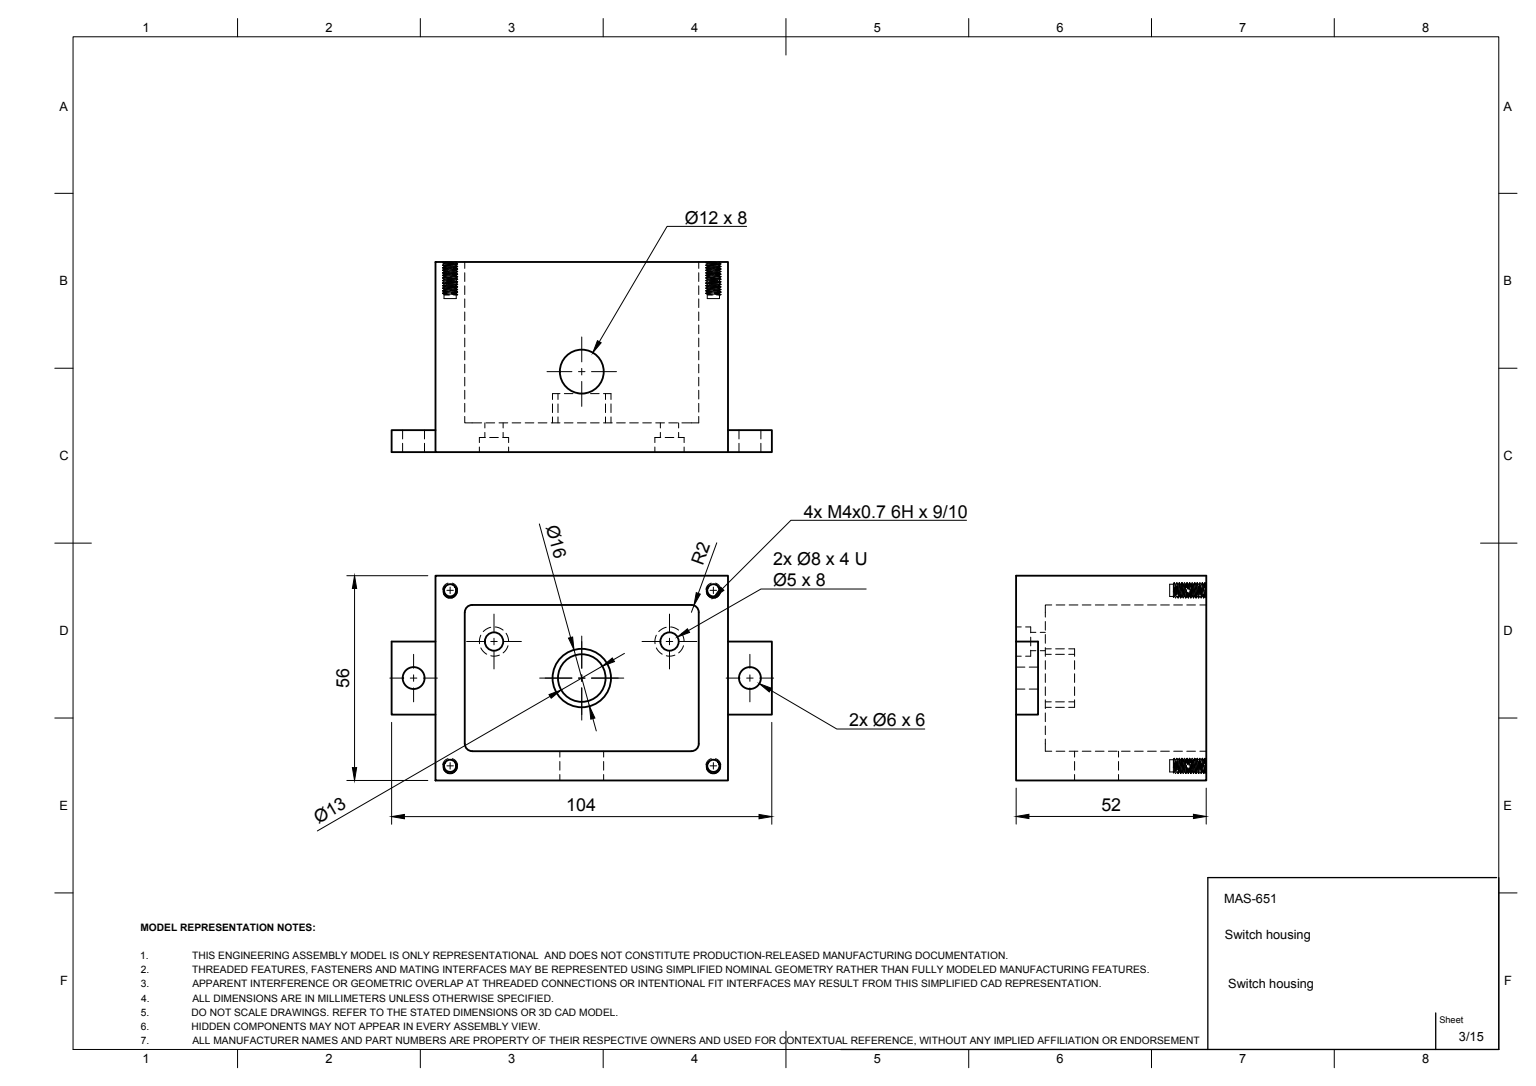
ISO-10303-21;
HEADER;
/* Generated by software containing ST-Developer
 * from STEP Tools, Inc. (www.steptools.com) 
 */

FILE_DESCRIPTION(
/* description */ ('Independent direct-acting normally-closed roller-plunger limit-switch
 CAD. Removable cover, insulated terminal supports, captured bus/conta
ct bridge, native Coil return spring, integral lower travel stop, reus
able instanced hardware and free roller. Manual geometric contact open
ing4mm; no snap-action/contact-force, electrical/current/voltage, envi
ronmental seal, safety-switch, wear, load or life certification. Exter
nal wiring and anchors omitted; fits and application engineering requi
red.'),
/* implementation_level */ '2;1');

FILE_NAME(
/* name */ 'Switch housing.step',
/* time_stamp */ '2026-11-08T07:32:43-08:00',
/* author */ (''),
/* organization */ (''),
/* preprocessor_version */ 'ST-DEVELOPER v20.2',
/* originating_system */ 'Autodesk Translation Framework v15.17.0.0',
/* authorisation */ '');

FILE_SCHEMA (('AUTOMOTIVE_DESIGN { 1 0 10303 214 3 1 1 }'));
ENDSEC;

DATA;
#10=MECHANICAL_DESIGN_GEOMETRIC_PRESENTATION_REPRESENTATION('',(#176),#36482);
#142=SHAPE_REPRESENTATION_RELATIONSHIP('SRR','None',#36555,#159);
#159=ADVANCED_BREP_SHAPE_REPRESENTATION('',(#193),#36465);
#176=STYLED_ITEM('',(#36649),#193);
#193=MANIFOLD_SOLID_BREP('Body1',#9767);
#210=B_SPLINE_SURFACE_WITH_KNOTS('',3,3,((#16536,#16537,#16538,#16539,#16540,
#16541,#16542,#16543,#16544,#16545,#16546,#16547,#16548,#16549,#16550,#16551,
#16552,#16553,#16554,#16555,#16556,#16557,#16558,#16559,#16560,#16561,#16562,
#16563,#16564,#16565,#16566,#16567,#16568,#16569,#16570,#16571,#16572,#16573,
#16574,#16575,#16576,#16577,#16578,#16579,#16580,#16581,#16582,#16583,#16584,
#16585,#16586,#16587,#16588,#16589,#16590,#16591,#16592,#16593,#16594,#16595,
#16596,#16597,#16598,#16599,#16600,#16601,#16602,#16603,#16604,#16605,#16606,
#16607,#16608,#16609,#16610,#16611,#16612,#16613,#16614,#16615,#16616,#16617,
#16618,#16619,#16620,#16621),(#16622,#16623,#16624,#16625,#16626,#16627,
#16628,#16629,#16630,#16631,#16632,#16633,#16634,#16635,#16636,#16637,#16638,
#16639,#16640,#16641,#16642,#16643,#16644,#16645,#16646,#16647,#16648,#16649,
#16650,#16651,#16652,#16653,#16654,#16655,#16656,#16657,#16658,#16659,#16660,
#16661,#16662,#16663,#16664,#16665,#16666,#16667,#16668,#16669,#16670,#16671,
#16672,#16673,#16674,#16675,#16676,#16677,#16678,#16679,#16680,#16681,#16682,
#16683,#16684,#16685,#16686,#16687,#16688,#16689,#16690,#16691,#16692,#16693,
#16694,#16695,#16696,#16697,#16698,#16699,#16700,#16701,#16702,#16703,#16704,
#16705,#16706,#16707),(#16708,#16709,#16710,#16711,#16712,#16713,#16714,
#16715,#16716,#16717,#16718,#16719,#16720,#16721,#16722,#16723,#16724,#16725,
#16726,#16727,#16728,#16729,#16730,#16731,#16732,#16733,#16734,#16735,#16736,
#16737,#16738,#16739,#16740,#16741,#16742,#16743,#16744,#16745,#16746,#16747,
#16748,#16749,#16750,#16751,#16752,#16753,#16754,#16755,#16756,#16757,#16758,
#16759,#16760,#16761,#16762,#16763,#16764,#16765,#16766,#16767,#16768,#16769,
#16770,#16771,#16772,#16773,#16774,#16775,#16776,#16777,#16778,#16779,#16780,
#16781,#16782,#16783,#16784,#16785,#16786,#16787,#16788,#16789,#16790,#16791,
#16792,#16793),(#16794,#16795,#16796,#16797,#16798,#16799,#16800,#16801,
#16802,#16803,#16804,#16805,#16806,#16807,#16808,#16809,#16810,#16811,#16812,
#16813,#16814,#16815,#16816,#16817,#16818,#16819,#16820,#16821,#16822,#16823,
#16824,#16825,#16826,#16827,#16828,#16829,#16830,#16831,#16832,#16833,#16834,
#16835,#16836,#16837,#16838,#16839,#16840,#16841,#16842,#16843,#16844,#16845,
#16846,#16847,#16848,#16849,#16850,#16851,#16852,#16853,#16854,#16855,#16856,
#16857,#16858,#16859,#16860,#16861,#16862,#16863,#16864,#16865,#16866,#16867,
#16868,#16869,#16870,#16871,#16872,#16873,#16874,#16875,#16876,#16877,#16878,
#16879)),.UNSPECIFIED.,.F.,.F.,.F.,(4,4),(4,1,1,1,1,1,1,1,1,1,1,1,1,1,1,
1,1,1,1,1,1,1,1,1,1,1,1,1,1,1,1,1,1,1,1,1,1,1,1,1,1,1,1,1,1,1,1,1,1,1,1,
1,1,1,1,1,1,1,1,1,1,1,1,1,1,1,1,1,1,1,1,1,1,1,1,1,1,1,1,1,1,1,1,4),(0.,
0.0448889834294937),(11.8615800042567,12.8591513772396,13.8567227502226,
14.8542941232055,15.8518654961884,16.8494368691714,17.8470082421543,18.8445796151372,
19.8421509881202,20.8397223611031,21.837293734086,22.834865107069,23.8324364800519,
24.8300078530348,25.8275792260178,26.8251505990007,27.8227219719836,28.8202933449666,
29.8178647179495,30.8154360909324,31.8130074639154,32.8105788368983,33.8081502098812,
34.8057215828642,35.8032929558471,36.80086432883,37.798435701813,38.7960070747959,
39.7935784477789,40.7911498207618,41.7887211937447,42.7862925667277,43.7838639397106,
44.7814353126935,45.7790066856765,46.7765780586594,47.7741494316423,48.7717208046253,
49.7692921776082,50.7668635505911,51.7644349235741,52.762006296557,53.7595776695399,
54.7571490425229,55.7547204155058,56.7522917884887,57.7498631614717,58.7474345344546,
59.7450059074375,60.7425772804205,61.7401486534034,62.7377200263864,63.7352913993693,
64.7328627723522,65.7304341453352,66.7280055183181,67.725576891301,68.723148264284,
69.7207196372669,70.7182910102498,71.7158623832328,72.7134337562157,73.7110051291986,
74.7085765021816,75.7061478751645,76.7037192481474,77.7012906211304,78.6988619941133,
79.6964333670962,80.6940047400792,81.6915761130621,82.689147486045,83.686718859028,
84.6842902320109,85.6818616049939,86.6794329779768,87.6770043509597,88.6745757239427,
89.6721470969256,90.6697184699085,91.6672898428915,92.6648612158744,93.6624325888573,
94.6600039618403),.UNSPECIFIED.);
#211=B_SPLINE_SURFACE_WITH_KNOTS('',3,3,((#16957,#16958,#16959,#16960,#16961,
#16962,#16963,#16964,#16965,#16966,#16967,#16968,#16969,#16970,#16971,#16972,
#16973,#16974,#16975,#16976,#16977,#16978,#16979,#16980,#16981,#16982,#16983,
#16984,#16985,#16986,#16987,#16988,#16989,#16990,#16991,#16992,#16993,#16994,
#16995,#16996,#16997,#16998,#16999,#17000,#17001,#17002,#17003,#17004,#17005,
#17006,#17007,#17008,#17009,#17010,#17011,#17012,#17013,#17014,#17015,#17016,
#17017,#17018,#17019,#17020,#17021,#17022,#17023,#17024,#17025,#17026,#17027,
#17028,#17029,#17030,#17031,#17032,#17033,#17034,#17035,#17036,#17037,#17038,
#17039,#17040,#17041,#17042),(#17043,#17044,#17045,#17046,#17047,#17048,
#17049,#17050,#17051,#17052,#17053,#17054,#17055,#17056,#17057,#17058,#17059,
#17060,#17061,#17062,#17063,#17064,#17065,#17066,#17067,#17068,#17069,#17070,
#17071,#17072,#17073,#17074,#17075,#17076,#17077,#17078,#17079,#17080,#17081,
#17082,#17083,#17084,#17085,#17086,#17087,#17088,#17089,#17090,#17091,#17092,
#17093,#17094,#17095,#17096,#17097,#17098,#17099,#17100,#17101,#17102,#17103,
#17104,#17105,#17106,#17107,#17108,#17109,#17110,#17111,#17112,#17113,#17114,
#17115,#17116,#17117,#17118,#17119,#17120,#17121,#17122,#17123,#17124,#17125,
#17126,#17127,#17128),(#17129,#17130,#17131,#17132,#17133,#17134,#17135,
#17136,#17137,#17138,#17139,#17140,#17141,#17142,#17143,#17144,#17145,#17146,
#17147,#17148,#17149,#17150,#17151,#17152,#17153,#17154,#17155,#17156,#17157,
#17158,#17159,#17160,#17161,#17162,#17163,#17164,#17165,#17166,#17167,#17168,
#17169,#17170,#17171,#17172,#17173,#17174,#17175,#17176,#17177,#17178,#17179,
#17180,#17181,#17182,#17183,#17184,#17185,#17186,#17187,#17188,#17189,#17190,
#17191,#17192,#17193,#17194,#17195,#17196,#17197,#17198,#17199,#17200,#17201,
#17202,#17203,#17204,#17205,#17206,#17207,#17208,#17209,#17210,#17211,#17212,
#17213,#17214),(#17215,#17216,#17217,#17218,#17219,#17220,#17221,#17222,
#17223,#17224,#17225,#17226,#17227,#17228,#17229,#17230,#17231,#17232,#17233,
#17234,#17235,#17236,#17237,#17238,#17239,#17240,#17241,#17242,#17243,#17244,
#17245,#17246,#17247,#17248,#17249,#17250,#17251,#17252,#17253,#17254,#17255,
#17256,#17257,#17258,#17259,#17260,#17261,#17262,#17263,#17264,#17265,#17266,
#17267,#17268,#17269,#17270,#17271,#17272,#17273,#17274,#17275,#17276,#17277,
#17278,#17279,#17280,#17281,#17282,#17283,#17284,#17285,#17286,#17287,#17288,
#17289,#17290,#17291,#17292,#17293,#17294,#17295,#17296,#17297,#17298,#17299,
#17300)),.UNSPECIFIED.,.F.,.F.,.F.,(4,4),(4,1,1,1,1,1,1,1,1,1,1,1,1,1,1,
1,1,1,1,1,1,1,1,1,1,1,1,1,1,1,1,1,1,1,1,1,1,1,1,1,1,1,1,1,1,1,1,1,1,1,1,
1,1,1,1,1,1,1,1,1,1,1,1,1,1,1,1,1,1,1,1,1,1,1,1,1,1,1,1,1,1,1,1,4),(0.,
0.0448889834294937),(14.3981410127769,15.3957123857599,16.3932837587428,
17.3908551317257,18.3884265047087,19.3859978776916,20.3835692506745,21.3811406236575,
22.3787119966404,23.3762833696233,24.3738547426063,25.3714261155892,26.3689974885721,
27.3665688615551,28.364140234538,29.3617116075209,30.3592829805039,31.3568543534868,
32.3544257264697,33.3519970994527,34.3495684724356,35.3471398454185,36.3447112184015,
37.3422825913844,38.3398539643674,39.3374253373503,40.3349967103332,41.3325680833162,
42.3301394562991,43.327710829282,44.325282202265,45.3228535752479,46.3204249482308,
47.3179963212138,48.3155676941967,49.3131390671796,50.3107104401626,51.3082818131455,
52.3058531861284,53.3034245591114,54.3009959320943,55.2985673050772,56.2961386780602,
57.2937100510431,58.291281424026,59.288852797009,60.2864241699919,61.2839955429748,
62.2815669159578,63.2791382889407,64.2767096619236,65.2742810349066,66.2718524078895,
67.2694237808725,68.2669951538554,69.2645665268383,70.2621378998213,71.2597092728042,
72.2572806457871,73.2548520187701,74.252423391753,75.2499947647359,76.2475661377189,
77.2451375107018,78.2427088836847,79.2402802566677,80.2378516296506,81.2354230026336,
82.2329943756165,83.2305657485994,84.2281371215823,85.2257084945653,86.2232798675482,
87.2208512405312,88.2184226135141,89.215993986497,90.21356535948,91.2111367324629,
92.2087081054458,93.2062794784288,94.2038508514117,95.2014222243946,96.1989935973776,
97.1965649703605),.UNSPECIFIED.);
#212=B_SPLINE_SURFACE_WITH_KNOTS('',3,3,((#17509,#17510,#17511,#17512,#17513,
#17514,#17515,#17516,#17517,#17518,#17519,#17520,#17521,#17522,#17523,#17524,
#17525,#17526,#17527,#17528,#17529,#17530,#17531,#17532,#17533,#17534,#17535,
#17536,#17537,#17538,#17539,#17540,#17541,#17542,#17543,#17544,#17545,#17546,
#17547,#17548,#17549,#17550,#17551,#17552,#17553,#17554,#17555,#17556,#17557,
#17558,#17559,#17560,#17561,#17562,#17563,#17564,#17565,#17566,#17567,#17568,
#17569,#17570,#17571,#17572,#17573,#17574,#17575,#17576,#17577,#17578,#17579,
#17580,#17581,#17582,#17583,#17584,#17585,#17586,#17587,#17588,#17589,#17590,
#17591,#17592,#17593,#17594),(#17595,#17596,#17597,#17598,#17599,#17600,
#17601,#17602,#17603,#17604,#17605,#17606,#17607,#17608,#17609,#17610,#17611,
#17612,#17613,#17614,#17615,#17616,#17617,#17618,#17619,#17620,#17621,#17622,
#17623,#17624,#17625,#17626,#17627,#17628,#17629,#17630,#17631,#17632,#17633,
#17634,#17635,#17636,#17637,#17638,#17639,#17640,#17641,#17642,#17643,#17644,
#17645,#17646,#17647,#17648,#17649,#17650,#17651,#17652,#17653,#17654,#17655,
#17656,#17657,#17658,#17659,#17660,#17661,#17662,#17663,#17664,#17665,#17666,
#17667,#17668,#17669,#17670,#17671,#17672,#17673,#17674,#17675,#17676,#17677,
#17678,#17679,#17680),(#17681,#17682,#17683,#17684,#17685,#17686,#17687,
#17688,#17689,#17690,#17691,#17692,#17693,#17694,#17695,#17696,#17697,#17698,
#17699,#17700,#17701,#17702,#17703,#17704,#17705,#17706,#17707,#17708,#17709,
#17710,#17711,#17712,#17713,#17714,#17715,#17716,#17717,#17718,#17719,#17720,
#17721,#17722,#17723,#17724,#17725,#17726,#17727,#17728,#17729,#17730,#17731,
#17732,#17733,#17734,#17735,#17736,#17737,#17738,#17739,#17740,#17741,#17742,
#17743,#17744,#17745,#17746,#17747,#17748,#17749,#17750,#17751,#17752,#17753,
#17754,#17755,#17756,#17757,#17758,#17759,#17760,#17761,#17762,#17763,#17764,
#17765,#17766),(#17767,#17768,#17769,#17770,#17771,#17772,#17773,#17774,
#17775,#17776,#17777,#17778,#17779,#17780,#17781,#17782,#17783,#17784,#17785,
#17786,#17787,#17788,#17789,#17790,#17791,#17792,#17793,#17794,#17795,#17796,
#17797,#17798,#17799,#17800,#17801,#17802,#17803,#17804,#17805,#17806,#17807,
#17808,#17809,#17810,#17811,#17812,#17813,#17814,#17815,#17816,#17817,#17818,
#17819,#17820,#17821,#17822,#17823,#17824,#17825,#17826,#17827,#17828,#17829,
#17830,#17831,#17832,#17833,#17834,#17835,#17836,#17837,#17838,#17839,#17840,
#17841,#17842,#17843,#17844,#17845,#17846,#17847,#17848,#17849,#17850,#17851,
#17852)),.UNSPECIFIED.,.F.,.F.,.F.,(4,4),(4,1,1,1,1,1,1,1,1,1,1,1,1,1,1,
1,1,1,1,1,1,1,1,1,1,1,1,1,1,1,1,1,1,1,1,1,1,1,1,1,1,1,1,1,1,1,1,1,1,1,1,
1,1,1,1,1,1,1,1,1,1,1,1,1,1,1,1,1,1,1,1,1,1,1,1,1,1,1,1,1,1,1,1,4),(0.,
0.0448889834294937),(11.8615800042567,12.8591513772396,13.8567227502226,
14.8542941232055,15.8518654961884,16.8494368691714,17.8470082421543,18.8445796151372,
19.8421509881202,20.8397223611031,21.837293734086,22.834865107069,23.8324364800519,
24.8300078530348,25.8275792260178,26.8251505990007,27.8227219719836,28.8202933449666,
29.8178647179495,30.8154360909324,31.8130074639154,32.8105788368983,33.8081502098812,
34.8057215828642,35.8032929558471,36.80086432883,37.798435701813,38.7960070747959,
39.7935784477789,40.7911498207618,41.7887211937447,42.7862925667277,43.7838639397106,
44.7814353126935,45.7790066856765,46.7765780586594,47.7741494316423,48.7717208046253,
49.7692921776082,50.7668635505911,51.7644349235741,52.762006296557,53.7595776695399,
54.7571490425229,55.7547204155058,56.7522917884887,57.7498631614717,58.7474345344546,
59.7450059074375,60.7425772804205,61.7401486534034,62.7377200263864,63.7352913993693,
64.7328627723522,65.7304341453352,66.7280055183181,67.725576891301,68.723148264284,
69.7207196372669,70.7182910102498,71.7158623832328,72.7134337562157,73.7110051291986,
74.7085765021816,75.7061478751645,76.7037192481474,77.7012906211304,78.6988619941133,
79.6964333670962,80.6940047400792,81.6915761130621,82.689147486045,83.686718859028,
84.6842902320109,85.6818616049939,86.6794329779768,87.6770043509597,88.6745757239427,
89.6721470969256,90.6697184699085,91.6672898428915,92.6648612158744,93.6624325888573,
94.6600039618403),.UNSPECIFIED.);
#213=B_SPLINE_SURFACE_WITH_KNOTS('',3,3,((#17930,#17931,#17932,#17933,#17934,
#17935,#17936,#17937,#17938,#17939,#17940,#17941,#17942,#17943,#17944,#17945,
#17946,#17947,#17948,#17949,#17950,#17951,#17952,#17953,#17954,#17955,#17956,
#17957,#17958,#17959,#17960,#17961,#17962,#17963,#17964,#17965,#17966,#17967,
#17968,#17969,#17970,#17971,#17972,#17973,#17974,#17975,#17976,#17977,#17978,
#17979,#17980,#17981,#17982,#17983,#17984,#17985,#17986,#17987,#17988,#17989,
#17990,#17991,#17992,#17993,#17994,#17995,#17996,#17997,#17998,#17999,#18000,
#18001,#18002,#18003,#18004,#18005,#18006,#18007,#18008,#18009,#18010,#18011,
#18012,#18013,#18014,#18015),(#18016,#18017,#18018,#18019,#18020,#18021,
#18022,#18023,#18024,#18025,#18026,#18027,#18028,#18029,#18030,#18031,#18032,
#18033,#18034,#18035,#18036,#18037,#18038,#18039,#18040,#18041,#18042,#18043,
#18044,#18045,#18046,#18047,#18048,#18049,#18050,#18051,#18052,#18053,#18054,
#18055,#18056,#18057,#18058,#18059,#18060,#18061,#18062,#18063,#18064,#18065,
#18066,#18067,#18068,#18069,#18070,#18071,#18072,#18073,#18074,#18075,#18076,
#18077,#18078,#18079,#18080,#18081,#18082,#18083,#18084,#18085,#18086,#18087,
#18088,#18089,#18090,#18091,#18092,#18093,#18094,#18095,#18096,#18097,#18098,
#18099,#18100,#18101),(#18102,#18103,#18104,#18105,#18106,#18107,#18108,
#18109,#18110,#18111,#18112,#18113,#18114,#18115,#18116,#18117,#18118,#18119,
#18120,#18121,#18122,#18123,#18124,#18125,#18126,#18127,#18128,#18129,#18130,
#18131,#18132,#18133,#18134,#18135,#18136,#18137,#18138,#18139,#18140,#18141,
#18142,#18143,#18144,#18145,#18146,#18147,#18148,#18149,#18150,#18151,#18152,
#18153,#18154,#18155,#18156,#18157,#18158,#18159,#18160,#18161,#18162,#18163,
#18164,#18165,#18166,#18167,#18168,#18169,#18170,#18171,#18172,#18173,#18174,
#18175,#18176,#18177,#18178,#18179,#18180,#18181,#18182,#18183,#18184,#18185,
#18186,#18187),(#18188,#18189,#18190,#18191,#18192,#18193,#18194,#18195,
#18196,#18197,#18198,#18199,#18200,#18201,#18202,#18203,#18204,#18205,#18206,
#18207,#18208,#18209,#18210,#18211,#18212,#18213,#18214,#18215,#18216,#18217,
#18218,#18219,#18220,#18221,#18222,#18223,#18224,#18225,#18226,#18227,#18228,
#18229,#18230,#18231,#18232,#18233,#18234,#18235,#18236,#18237,#18238,#18239,
#18240,#18241,#18242,#18243,#18244,#18245,#18246,#18247,#18248,#18249,#18250,
#18251,#18252,#18253,#18254,#18255,#18256,#18257,#18258,#18259,#18260,#18261,
#18262,#18263,#18264,#18265,#18266,#18267,#18268,#18269,#18270,#18271,#18272,
#18273)),.UNSPECIFIED.,.F.,.F.,.F.,(4,4),(4,1,1,1,1,1,1,1,1,1,1,1,1,1,1,
1,1,1,1,1,1,1,1,1,1,1,1,1,1,1,1,1,1,1,1,1,1,1,1,1,1,1,1,1,1,1,1,1,1,1,1,
1,1,1,1,1,1,1,1,1,1,1,1,1,1,1,1,1,1,1,1,1,1,1,1,1,1,1,1,1,1,1,1,4),(0.,
0.0448889834294937),(14.3981410127769,15.3957123857599,16.3932837587428,
17.3908551317257,18.3884265047087,19.3859978776916,20.3835692506745,21.3811406236575,
22.3787119966404,23.3762833696233,24.3738547426063,25.3714261155892,26.3689974885721,
27.3665688615551,28.364140234538,29.3617116075209,30.3592829805039,31.3568543534868,
32.3544257264697,33.3519970994527,34.3495684724356,35.3471398454185,36.3447112184015,
37.3422825913844,38.3398539643674,39.3374253373503,40.3349967103332,41.3325680833162,
42.3301394562991,43.327710829282,44.325282202265,45.3228535752479,46.3204249482308,
47.3179963212138,48.3155676941967,49.3131390671796,50.3107104401626,51.3082818131455,
52.3058531861284,53.3034245591114,54.3009959320943,55.2985673050772,56.2961386780602,
57.2937100510431,58.291281424026,59.288852797009,60.2864241699919,61.2839955429748,
62.2815669159578,63.2791382889407,64.2767096619237,65.2742810349066,66.2718524078895,
67.2694237808725,68.2669951538554,69.2645665268383,70.2621378998213,71.2597092728042,
72.2572806457871,73.2548520187701,74.252423391753,75.2499947647359,76.2475661377189,
77.2451375107018,78.2427088836847,79.2402802566677,80.2378516296506,81.2354230026336,
82.2329943756165,83.2305657485994,84.2281371215823,85.2257084945653,86.2232798675482,
87.2208512405312,88.2184226135141,89.215993986497,90.21356535948,91.2111367324629,
92.2087081054458,93.2062794784288,94.2038508514117,95.2014222243946,96.1989935973776,
97.1965649703605),.UNSPECIFIED.);
#214=B_SPLINE_SURFACE_WITH_KNOTS('',3,3,((#18482,#18483,#18484,#18485,#18486,
#18487,#18488,#18489,#18490,#18491,#18492,#18493,#18494,#18495,#18496,#18497,
#18498,#18499,#18500,#18501,#18502,#18503,#18504,#18505,#18506,#18507,#18508,
#18509,#18510,#18511,#18512,#18513,#18514,#18515,#18516,#18517,#18518,#18519,
#18520,#18521,#18522,#18523,#18524,#18525,#18526,#18527,#18528,#18529,#18530,
#18531,#18532,#18533,#18534,#18535,#18536,#18537,#18538,#18539,#18540,#18541,
#18542,#18543,#18544,#18545,#18546,#18547,#18548,#18549,#18550,#18551,#18552,
#18553,#18554,#18555,#18556,#18557,#18558,#18559,#18560,#18561,#18562,#18563,
#18564,#18565,#18566,#18567),(#18568,#18569,#18570,#18571,#18572,#18573,
#18574,#18575,#18576,#18577,#18578,#18579,#18580,#18581,#18582,#18583,#18584,
#18585,#18586,#18587,#18588,#18589,#18590,#18591,#18592,#18593,#18594,#18595,
#18596,#18597,#18598,#18599,#18600,#18601,#18602,#18603,#18604,#18605,#18606,
#18607,#18608,#18609,#18610,#18611,#18612,#18613,#18614,#18615,#18616,#18617,
#18618,#18619,#18620,#18621,#18622,#18623,#18624,#18625,#18626,#18627,#18628,
#18629,#18630,#18631,#18632,#18633,#18634,#18635,#18636,#18637,#18638,#18639,
#18640,#18641,#18642,#18643,#18644,#18645,#18646,#18647,#18648,#18649,#18650,
#18651,#18652,#18653),(#18654,#18655,#18656,#18657,#18658,#18659,#18660,
#18661,#18662,#18663,#18664,#18665,#18666,#18667,#18668,#18669,#18670,#18671,
#18672,#18673,#18674,#18675,#18676,#18677,#18678,#18679,#18680,#18681,#18682,
#18683,#18684,#18685,#18686,#18687,#18688,#18689,#18690,#18691,#18692,#18693,
#18694,#18695,#18696,#18697,#18698,#18699,#18700,#18701,#18702,#18703,#18704,
#18705,#18706,#18707,#18708,#18709,#18710,#18711,#18712,#18713,#18714,#18715,
#18716,#18717,#18718,#18719,#18720,#18721,#18722,#18723,#18724,#18725,#18726,
#18727,#18728,#18729,#18730,#18731,#18732,#18733,#18734,#18735,#18736,#18737,
#18738,#18739),(#18740,#18741,#18742,#18743,#18744,#18745,#18746,#18747,
#18748,#18749,#18750,#18751,#18752,#18753,#18754,#18755,#18756,#18757,#18758,
#18759,#18760,#18761,#18762,#18763,#18764,#18765,#18766,#18767,#18768,#18769,
#18770,#18771,#18772,#18773,#18774,#18775,#18776,#18777,#18778,#18779,#18780,
#18781,#18782,#18783,#18784,#18785,#18786,#18787,#18788,#18789,#18790,#18791,
#18792,#18793,#18794,#18795,#18796,#18797,#18798,#18799,#18800,#18801,#18802,
#18803,#18804,#18805,#18806,#18807,#18808,#18809,#18810,#18811,#18812,#18813,
#18814,#18815,#18816,#18817,#18818,#18819,#18820,#18821,#18822,#18823,#18824,
#18825)),.UNSPECIFIED.,.F.,.F.,.F.,(4,4),(4,1,1,1,1,1,1,1,1,1,1,1,1,1,1,
1,1,1,1,1,1,1,1,1,1,1,1,1,1,1,1,1,1,1,1,1,1,1,1,1,1,1,1,1,1,1,1,1,1,1,1,
1,1,1,1,1,1,1,1,1,1,1,1,1,1,1,1,1,1,1,1,1,1,1,1,1,1,1,1,1,1,1,1,4),(0.,
0.0448889834294937),(11.8615800042567,12.8591513772396,13.8567227502225,
14.8542941232055,15.8518654961884,16.8494368691713,17.8470082421543,18.8445796151372,
19.8421509881201,20.8397223611031,21.837293734086,22.8348651070689,23.8324364800519,
24.8300078530348,25.8275792260178,26.8251505990007,27.8227219719836,28.8202933449666,
29.8178647179495,30.8154360909324,31.8130074639154,32.8105788368983,33.8081502098812,
34.8057215828642,35.8032929558471,36.80086432883,37.798435701813,38.7960070747959,
39.7935784477788,40.7911498207618,41.7887211937447,42.7862925667276,43.7838639397106,
44.7814353126935,45.7790066856764,46.7765780586594,47.7741494316423,48.7717208046252,
49.7692921776082,50.7668635505911,51.764434923574,52.762006296557,53.7595776695399,
54.7571490425228,55.7547204155058,56.7522917884887,57.7498631614716,58.7474345344546,
59.7450059074375,60.7425772804204,61.7401486534034,62.7377200263863,63.7352913993692,
64.7328627723522,65.7304341453351,66.728005518318,67.725576891301,68.7231482642839,
69.7207196372668,70.7182910102498,71.7158623832327,72.7134337562156,73.7110051291986,
74.7085765021815,75.7061478751644,76.7037192481474,77.7012906211303,78.6988619941132,
79.6964333670962,80.6940047400791,81.6915761130621,82.689147486045,83.6867188590279,
84.6842902320109,85.6818616049938,86.6794329779767,87.6770043509596,88.6745757239426,
89.6721470969255,90.6697184699085,91.6672898428914,92.6648612158743,93.6624325888573,
94.6600039618402),.UNSPECIFIED.);
#215=B_SPLINE_SURFACE_WITH_KNOTS('',3,3,((#18903,#18904,#18905,#18906,#18907,
#18908,#18909,#18910,#18911,#18912,#18913,#18914,#18915,#18916,#18917,#18918,
#18919,#18920,#18921,#18922,#18923,#18924,#18925,#18926,#18927,#18928,#18929,
#18930,#18931,#18932,#18933,#18934,#18935,#18936,#18937,#18938,#18939,#18940,
#18941,#18942,#18943,#18944,#18945,#18946,#18947,#18948,#18949,#18950,#18951,
#18952,#18953,#18954,#18955,#18956,#18957,#18958,#18959,#18960,#18961,#18962,
#18963,#18964,#18965,#18966,#18967,#18968,#18969,#18970,#18971,#18972,#18973,
#18974,#18975,#18976,#18977,#18978,#18979,#18980,#18981,#18982,#18983,#18984,
#18985,#18986,#18987,#18988),(#18989,#18990,#18991,#18992,#18993,#18994,
#18995,#18996,#18997,#18998,#18999,#19000,#19001,#19002,#19003,#19004,#19005,
#19006,#19007,#19008,#19009,#19010,#19011,#19012,#19013,#19014,#19015,#19016,
#19017,#19018,#19019,#19020,#19021,#19022,#19023,#19024,#19025,#19026,#19027,
#19028,#19029,#19030,#19031,#19032,#19033,#19034,#19035,#19036,#19037,#19038,
#19039,#19040,#19041,#19042,#19043,#19044,#19045,#19046,#19047,#19048,#19049,
#19050,#19051,#19052,#19053,#19054,#19055,#19056,#19057,#19058,#19059,#19060,
#19061,#19062,#19063,#19064,#19065,#19066,#19067,#19068,#19069,#19070,#19071,
#19072,#19073,#19074),(#19075,#19076,#19077,#19078,#19079,#19080,#19081,
#19082,#19083,#19084,#19085,#19086,#19087,#19088,#19089,#19090,#19091,#19092,
#19093,#19094,#19095,#19096,#19097,#19098,#19099,#19100,#19101,#19102,#19103,
#19104,#19105,#19106,#19107,#19108,#19109,#19110,#19111,#19112,#19113,#19114,
#19115,#19116,#19117,#19118,#19119,#19120,#19121,#19122,#19123,#19124,#19125,
#19126,#19127,#19128,#19129,#19130,#19131,#19132,#19133,#19134,#19135,#19136,
#19137,#19138,#19139,#19140,#19141,#19142,#19143,#19144,#19145,#19146,#19147,
#19148,#19149,#19150,#19151,#19152,#19153,#19154,#19155,#19156,#19157,#19158,
#19159,#19160),(#19161,#19162,#19163,#19164,#19165,#19166,#19167,#19168,
#19169,#19170,#19171,#19172,#19173,#19174,#19175,#19176,#19177,#19178,#19179,
#19180,#19181,#19182,#19183,#19184,#19185,#19186,#19187,#19188,#19189,#19190,
#19191,#19192,#19193,#19194,#19195,#19196,#19197,#19198,#19199,#19200,#19201,
#19202,#19203,#19204,#19205,#19206,#19207,#19208,#19209,#19210,#19211,#19212,
#19213,#19214,#19215,#19216,#19217,#19218,#19219,#19220,#19221,#19222,#19223,
#19224,#19225,#19226,#19227,#19228,#19229,#19230,#19231,#19232,#19233,#19234,
#19235,#19236,#19237,#19238,#19239,#19240,#19241,#19242,#19243,#19244,#19245,
#19246)),.UNSPECIFIED.,.F.,.F.,.F.,(4,4),(4,1,1,1,1,1,1,1,1,1,1,1,1,1,1,
1,1,1,1,1,1,1,1,1,1,1,1,1,1,1,1,1,1,1,1,1,1,1,1,1,1,1,1,1,1,1,1,1,1,1,1,
1,1,1,1,1,1,1,1,1,1,1,1,1,1,1,1,1,1,1,1,1,1,1,1,1,1,1,1,1,1,1,1,4),(0.,
0.0448889834294937),(14.3981410127769,15.3957123857599,16.3932837587428,
17.3908551317257,18.3884265047087,19.3859978776916,20.3835692506745,21.3811406236575,
22.3787119966404,23.3762833696233,24.3738547426063,25.3714261155892,26.3689974885721,
27.3665688615551,28.364140234538,29.3617116075209,30.3592829805039,31.3568543534868,
32.3544257264697,33.3519970994527,34.3495684724356,35.3471398454185,36.3447112184015,
37.3422825913844,38.3398539643673,39.3374253373503,40.3349967103332,41.3325680833161,
42.3301394562991,43.327710829282,44.3252822022649,45.3228535752479,46.3204249482308,
47.3179963212137,48.3155676941967,49.3131390671796,50.3107104401625,51.3082818131455,
52.3058531861284,53.3034245591113,54.3009959320943,55.2985673050772,56.2961386780601,
57.2937100510431,58.291281424026,59.2888527970089,60.2864241699919,61.2839955429748,
62.2815669159577,63.2791382889407,64.2767096619236,65.2742810349065,66.2718524078895,
67.2694237808724,68.2669951538553,69.2645665268383,70.2621378998212,71.2597092728041,
72.2572806457871,73.25485201877,74.2524233917529,75.2499947647359,76.2475661377188,
77.2451375107017,78.2427088836847,79.2402802566676,80.2378516296505,81.2354230026335,
82.2329943756164,83.2305657485993,84.2281371215823,85.2257084945652,86.2232798675481,
87.2208512405311,88.218422613514,89.2159939864969,90.2135653594799,91.2111367324628,
92.2087081054457,93.2062794784287,94.2038508514116,95.2014222243945,96.1989935973775,
97.1965649703604),.UNSPECIFIED.);
#216=B_SPLINE_SURFACE_WITH_KNOTS('',3,3,((#19455,#19456,#19457,#19458,#19459,
#19460,#19461,#19462,#19463,#19464,#19465,#19466,#19467,#19468,#19469,#19470,
#19471,#19472,#19473,#19474,#19475,#19476,#19477,#19478,#19479,#19480,#19481,
#19482,#19483,#19484,#19485,#19486,#19487,#19488,#19489,#19490,#19491,#19492,
#19493,#19494,#19495,#19496,#19497,#19498,#19499,#19500,#19501,#19502,#19503,
#19504,#19505,#19506,#19507,#19508,#19509,#19510,#19511,#19512,#19513,#19514,
#19515,#19516,#19517,#19518,#19519,#19520,#19521,#19522,#19523,#19524,#19525,
#19526,#19527,#19528,#19529,#19530,#19531,#19532,#19533,#19534,#19535,#19536,
#19537,#19538,#19539,#19540),(#19541,#19542,#19543,#19544,#19545,#19546,
#19547,#19548,#19549,#19550,#19551,#19552,#19553,#19554,#19555,#19556,#19557,
#19558,#19559,#19560,#19561,#19562,#19563,#19564,#19565,#19566,#19567,#19568,
#19569,#19570,#19571,#19572,#19573,#19574,#19575,#19576,#19577,#19578,#19579,
#19580,#19581,#19582,#19583,#19584,#19585,#19586,#19587,#19588,#19589,#19590,
#19591,#19592,#19593,#19594,#19595,#19596,#19597,#19598,#19599,#19600,#19601,
#19602,#19603,#19604,#19605,#19606,#19607,#19608,#19609,#19610,#19611,#19612,
#19613,#19614,#19615,#19616,#19617,#19618,#19619,#19620,#19621,#19622,#19623,
#19624,#19625,#19626),(#19627,#19628,#19629,#19630,#19631,#19632,#19633,
#19634,#19635,#19636,#19637,#19638,#19639,#19640,#19641,#19642,#19643,#19644,
#19645,#19646,#19647,#19648,#19649,#19650,#19651,#19652,#19653,#19654,#19655,
#19656,#19657,#19658,#19659,#19660,#19661,#19662,#19663,#19664,#19665,#19666,
#19667,#19668,#19669,#19670,#19671,#19672,#19673,#19674,#19675,#19676,#19677,
#19678,#19679,#19680,#19681,#19682,#19683,#19684,#19685,#19686,#19687,#19688,
#19689,#19690,#19691,#19692,#19693,#19694,#19695,#19696,#19697,#19698,#19699,
#19700,#19701,#19702,#19703,#19704,#19705,#19706,#19707,#19708,#19709,#19710,
#19711,#19712),(#19713,#19714,#19715,#19716,#19717,#19718,#19719,#19720,
#19721,#19722,#19723,#19724,#19725,#19726,#19727,#19728,#19729,#19730,#19731,
#19732,#19733,#19734,#19735,#19736,#19737,#19738,#19739,#19740,#19741,#19742,
#19743,#19744,#19745,#19746,#19747,#19748,#19749,#19750,#19751,#19752,#19753,
#19754,#19755,#19756,#19757,#19758,#19759,#19760,#19761,#19762,#19763,#19764,
#19765,#19766,#19767,#19768,#19769,#19770,#19771,#19772,#19773,#19774,#19775,
#19776,#19777,#19778,#19779,#19780,#19781,#19782,#19783,#19784,#19785,#19786,
#19787,#19788,#19789,#19790,#19791,#19792,#19793,#19794,#19795,#19796,#19797,
#19798)),.UNSPECIFIED.,.F.,.F.,.F.,(4,4),(4,1,1,1,1,1,1,1,1,1,1,1,1,1,1,
1,1,1,1,1,1,1,1,1,1,1,1,1,1,1,1,1,1,1,1,1,1,1,1,1,1,1,1,1,1,1,1,1,1,1,1,
1,1,1,1,1,1,1,1,1,1,1,1,1,1,1,1,1,1,1,1,1,1,1,1,1,1,1,1,1,1,1,1,4),(0.,
0.0448889834294937),(11.8615800042567,12.8591513772396,13.8567227502225,
14.8542941232055,15.8518654961884,16.8494368691713,17.8470082421543,18.8445796151372,
19.8421509881202,20.8397223611031,21.837293734086,22.834865107069,23.8324364800519,
24.8300078530348,25.8275792260178,26.8251505990007,27.8227219719836,28.8202933449666,
29.8178647179495,30.8154360909324,31.8130074639154,32.8105788368983,33.8081502098812,
34.8057215828642,35.8032929558471,36.80086432883,37.798435701813,38.7960070747959,
39.7935784477788,40.7911498207618,41.7887211937447,42.7862925667276,43.7838639397106,
44.7814353126935,45.7790066856764,46.7765780586594,47.7741494316423,48.7717208046252,
49.7692921776082,50.7668635505911,51.764434923574,52.762006296557,53.7595776695399,
54.7571490425228,55.7547204155058,56.7522917884887,57.7498631614716,58.7474345344546,
59.7450059074375,60.7425772804204,61.7401486534034,62.7377200263863,63.7352913993692,
64.7328627723522,65.7304341453351,66.728005518318,67.725576891301,68.7231482642839,
69.7207196372669,70.7182910102498,71.7158623832327,72.7134337562156,73.7110051291986,
74.7085765021815,75.7061478751644,76.7037192481474,77.7012906211303,78.6988619941132,
79.6964333670962,80.6940047400791,81.6915761130621,82.689147486045,83.6867188590279,
84.6842902320109,85.6818616049938,86.6794329779767,87.6770043509596,88.6745757239426,
89.6721470969255,90.6697184699085,91.6672898428914,92.6648612158743,93.6624325888573,
94.6600039618402),.UNSPECIFIED.);
#217=B_SPLINE_SURFACE_WITH_KNOTS('',3,3,((#19876,#19877,#19878,#19879,#19880,
#19881,#19882,#19883,#19884,#19885,#19886,#19887,#19888,#19889,#19890,#19891,
#19892,#19893,#19894,#19895,#19896,#19897,#19898,#19899,#19900,#19901,#19902,
#19903,#19904,#19905,#19906,#19907,#19908,#19909,#19910,#19911,#19912,#19913,
#19914,#19915,#19916,#19917,#19918,#19919,#19920,#19921,#19922,#19923,#19924,
#19925,#19926,#19927,#19928,#19929,#19930,#19931,#19932,#19933,#19934,#19935,
#19936,#19937,#19938,#19939,#19940,#19941,#19942,#19943,#19944,#19945,#19946,
#19947,#19948,#19949,#19950,#19951,#19952,#19953,#19954,#19955,#19956,#19957,
#19958,#19959,#19960,#19961),(#19962,#19963,#19964,#19965,#19966,#19967,
#19968,#19969,#19970,#19971,#19972,#19973,#19974,#19975,#19976,#19977,#19978,
#19979,#19980,#19981,#19982,#19983,#19984,#19985,#19986,#19987,#19988,#19989,
#19990,#19991,#19992,#19993,#19994,#19995,#19996,#19997,#19998,#19999,#20000,
#20001,#20002,#20003,#20004,#20005,#20006,#20007,#20008,#20009,#20010,#20011,
#20012,#20013,#20014,#20015,#20016,#20017,#20018,#20019,#20020,#20021,#20022,
#20023,#20024,#20025,#20026,#20027,#20028,#20029,#20030,#20031,#20032,#20033,
#20034,#20035,#20036,#20037,#20038,#20039,#20040,#20041,#20042,#20043,#20044,
#20045,#20046,#20047),(#20048,#20049,#20050,#20051,#20052,#20053,#20054,
#20055,#20056,#20057,#20058,#20059,#20060,#20061,#20062,#20063,#20064,#20065,
#20066,#20067,#20068,#20069,#20070,#20071,#20072,#20073,#20074,#20075,#20076,
#20077,#20078,#20079,#20080,#20081,#20082,#20083,#20084,#20085,#20086,#20087,
#20088,#20089,#20090,#20091,#20092,#20093,#20094,#20095,#20096,#20097,#20098,
#20099,#20100,#20101,#20102,#20103,#20104,#20105,#20106,#20107,#20108,#20109,
#20110,#20111,#20112,#20113,#20114,#20115,#20116,#20117,#20118,#20119,#20120,
#20121,#20122,#20123,#20124,#20125,#20126,#20127,#20128,#20129,#20130,#20131,
#20132,#20133),(#20134,#20135,#20136,#20137,#20138,#20139,#20140,#20141,
#20142,#20143,#20144,#20145,#20146,#20147,#20148,#20149,#20150,#20151,#20152,
#20153,#20154,#20155,#20156,#20157,#20158,#20159,#20160,#20161,#20162,#20163,
#20164,#20165,#20166,#20167,#20168,#20169,#20170,#20171,#20172,#20173,#20174,
#20175,#20176,#20177,#20178,#20179,#20180,#20181,#20182,#20183,#20184,#20185,
#20186,#20187,#20188,#20189,#20190,#20191,#20192,#20193,#20194,#20195,#20196,
#20197,#20198,#20199,#20200,#20201,#20202,#20203,#20204,#20205,#20206,#20207,
#20208,#20209,#20210,#20211,#20212,#20213,#20214,#20215,#20216,#20217,#20218,
#20219)),.UNSPECIFIED.,.F.,.F.,.F.,(4,4),(4,1,1,1,1,1,1,1,1,1,1,1,1,1,1,
1,1,1,1,1,1,1,1,1,1,1,1,1,1,1,1,1,1,1,1,1,1,1,1,1,1,1,1,1,1,1,1,1,1,1,1,
1,1,1,1,1,1,1,1,1,1,1,1,1,1,1,1,1,1,1,1,1,1,1,1,1,1,1,1,1,1,1,1,4),(0.,
0.0448889834294937),(14.3981410127769,15.3957123857599,16.3932837587428,
17.3908551317257,18.3884265047087,19.3859978776916,20.3835692506745,21.3811406236575,
22.3787119966404,23.3762833696233,24.3738547426063,25.3714261155892,26.3689974885721,
27.3665688615551,28.364140234538,29.3617116075209,30.3592829805039,31.3568543534868,
32.3544257264697,33.3519970994527,34.3495684724356,35.3471398454185,36.3447112184015,
37.3422825913844,38.3398539643673,39.3374253373503,40.3349967103332,41.3325680833161,
42.3301394562991,43.327710829282,44.3252822022649,45.3228535752479,46.3204249482308,
47.3179963212137,48.3155676941967,49.3131390671796,50.3107104401625,51.3082818131455,
52.3058531861284,53.3034245591113,54.3009959320943,55.2985673050772,56.2961386780601,
57.2937100510431,58.291281424026,59.2888527970089,60.2864241699919,61.2839955429748,
62.2815669159577,63.2791382889407,64.2767096619236,65.2742810349065,66.2718524078895,
67.2694237808724,68.2669951538553,69.2645665268383,70.2621378998212,71.2597092728041,
72.2572806457871,73.25485201877,74.2524233917529,75.2499947647359,76.2475661377188,
77.2451375107017,78.2427088836847,79.2402802566676,80.2378516296505,81.2354230026335,
82.2329943756164,83.2305657485993,84.2281371215823,85.2257084945652,86.2232798675481,
87.2208512405311,88.218422613514,89.2159939864969,90.2135653594799,91.2111367324628,
92.2087081054457,93.2062794784287,94.2038508514116,95.2014222243945,96.1989935973775,
97.1965649703604),.UNSPECIFIED.);
#235=FACE_BOUND('',#1083,.T.);
#236=FACE_BOUND('',#1084,.T.);
#237=FACE_BOUND('',#1085,.T.);
#238=FACE_BOUND('',#1087,.T.);
#239=FACE_BOUND('',#1091,.T.);
#240=FACE_BOUND('',#1095,.T.);
#241=FACE_BOUND('',#1128,.T.);
#242=FACE_BOUND('',#1133,.T.);
#243=FACE_BOUND('',#1137,.T.);
#244=FACE_BOUND('',#1143,.T.);
#245=FACE_BOUND('',#1146,.T.);
#246=FACE_BOUND('',#1147,.T.);
#247=FACE_BOUND('',#1148,.T.);
#248=FACE_BOUND('',#1149,.T.);
#249=FACE_BOUND('',#1150,.T.);
#250=FACE_BOUND('',#1152,.T.);
#251=FACE_BOUND('',#1153,.T.);
#252=FACE_BOUND('',#1154,.T.);
#253=FACE_BOUND('',#1155,.T.);
#302=PLANE('',#10097);
#303=PLANE('',#10101);
#304=PLANE('',#10105);
#305=PLANE('',#10110);
#306=PLANE('',#10116);
#307=PLANE('',#10122);
#308=PLANE('',#10128);
#309=PLANE('',#10131);
#310=PLANE('',#10134);
#311=PLANE('',#10137);
#312=PLANE('',#10140);
#313=PLANE('',#10141);
#314=PLANE('',#10142);
#315=PLANE('',#10143);
#316=PLANE('',#10150);
#317=PLANE('',#10151);
#318=PLANE('',#10152);
#319=PLANE('',#10153);
#320=PLANE('',#10154);
#321=PLANE('',#10155);
#322=PLANE('',#10156);
#323=PLANE('',#10157);
#324=PLANE('',#10163);
#325=PLANE('',#10164);
#326=PLANE('',#10165);
#327=PLANE('',#10166);
#328=PLANE('',#10167);
#329=PLANE('',#10168);
#330=PLANE('',#10169);
#331=PLANE('',#10170);
#332=PLANE('',#10171);
#439=FACE_OUTER_BOUND('',#977,.T.);
#440=FACE_OUTER_BOUND('',#978,.T.);
#441=FACE_OUTER_BOUND('',#979,.T.);
#442=FACE_OUTER_BOUND('',#980,.T.);
#443=FACE_OUTER_BOUND('',#981,.T.);
#444=FACE_OUTER_BOUND('',#982,.T.);
#445=FACE_OUTER_BOUND('',#983,.T.);
#446=FACE_OUTER_BOUND('',#984,.T.);
#447=FACE_OUTER_BOUND('',#985,.T.);
#448=FACE_OUTER_BOUND('',#986,.T.);
#449=FACE_OUTER_BOUND('',#987,.T.);
#450=FACE_OUTER_BOUND('',#988,.T.);
#451=FACE_OUTER_BOUND('',#989,.T.);
#452=FACE_OUTER_BOUND('',#990,.T.);
#453=FACE_OUTER_BOUND('',#991,.T.);
#454=FACE_OUTER_BOUND('',#992,.T.);
#455=FACE_OUTER_BOUND('',#993,.T.);
#456=FACE_OUTER_BOUND('',#994,.T.);
#457=FACE_OUTER_BOUND('',#995,.T.);
#458=FACE_OUTER_BOUND('',#996,.T.);
#459=FACE_OUTER_BOUND('',#997,.T.);
#460=FACE_OUTER_BOUND('',#998,.T.);
#461=FACE_OUTER_BOUND('',#999,.T.);
#462=FACE_OUTER_BOUND('',#1000,.T.);
#463=FACE_OUTER_BOUND('',#1001,.T.);
#464=FACE_OUTER_BOUND('',#1002,.T.);
#465=FACE_OUTER_BOUND('',#1003,.T.);
#466=FACE_OUTER_BOUND('',#1004,.T.);
#467=FACE_OUTER_BOUND('',#1005,.T.);
#468=FACE_OUTER_BOUND('',#1006,.T.);
#469=FACE_OUTER_BOUND('',#1007,.T.);
#470=FACE_OUTER_BOUND('',#1008,.T.);
#471=FACE_OUTER_BOUND('',#1009,.T.);
#472=FACE_OUTER_BOUND('',#1010,.T.);
#473=FACE_OUTER_BOUND('',#1011,.T.);
#474=FACE_OUTER_BOUND('',#1012,.T.);
#475=FACE_OUTER_BOUND('',#1013,.T.);
#476=FACE_OUTER_BOUND('',#1014,.T.);
#477=FACE_OUTER_BOUND('',#1015,.T.);
#478=FACE_OUTER_BOUND('',#1016,.T.);
#479=FACE_OUTER_BOUND('',#1017,.T.);
#480=FACE_OUTER_BOUND('',#1018,.T.);
#481=FACE_OUTER_BOUND('',#1019,.T.);
#482=FACE_OUTER_BOUND('',#1020,.T.);
#483=FACE_OUTER_BOUND('',#1021,.T.);
#484=FACE_OUTER_BOUND('',#1022,.T.);
#485=FACE_OUTER_BOUND('',#1023,.T.);
#486=FACE_OUTER_BOUND('',#1024,.T.);
#487=FACE_OUTER_BOUND('',#1025,.T.);
#488=FACE_OUTER_BOUND('',#1026,.T.);
#489=FACE_OUTER_BOUND('',#1027,.T.);
#490=FACE_OUTER_BOUND('',#1028,.T.);
#491=FACE_OUTER_BOUND('',#1029,.T.);
#492=FACE_OUTER_BOUND('',#1030,.T.);
#493=FACE_OUTER_BOUND('',#1031,.T.);
#494=FACE_OUTER_BOUND('',#1032,.T.);
#495=FACE_OUTER_BOUND('',#1033,.T.);
#496=FACE_OUTER_BOUND('',#1034,.T.);
#497=FACE_OUTER_BOUND('',#1035,.T.);
#498=FACE_OUTER_BOUND('',#1036,.T.);
#499=FACE_OUTER_BOUND('',#1037,.T.);
#500=FACE_OUTER_BOUND('',#1038,.T.);
#501=FACE_OUTER_BOUND('',#1039,.T.);
#502=FACE_OUTER_BOUND('',#1040,.T.);
#503=FACE_OUTER_BOUND('',#1041,.T.);
#504=FACE_OUTER_BOUND('',#1042,.T.);
#505=FACE_OUTER_BOUND('',#1043,.T.);
#506=FACE_OUTER_BOUND('',#1044,.T.);
#507=FACE_OUTER_BOUND('',#1045,.T.);
#508=FACE_OUTER_BOUND('',#1046,.T.);
#509=FACE_OUTER_BOUND('',#1047,.T.);
#510=FACE_OUTER_BOUND('',#1048,.T.);
#511=FACE_OUTER_BOUND('',#1049,.T.);
#512=FACE_OUTER_BOUND('',#1050,.T.);
#513=FACE_OUTER_BOUND('',#1051,.T.);
#514=FACE_OUTER_BOUND('',#1052,.T.);
#515=FACE_OUTER_BOUND('',#1053,.T.);
#516=FACE_OUTER_BOUND('',#1054,.T.);
#517=FACE_OUTER_BOUND('',#1055,.T.);
#518=FACE_OUTER_BOUND('',#1056,.T.);
#519=FACE_OUTER_BOUND('',#1057,.T.);
#520=FACE_OUTER_BOUND('',#1058,.T.);
#521=FACE_OUTER_BOUND('',#1059,.T.);
#522=FACE_OUTER_BOUND('',#1060,.T.);
#523=FACE_OUTER_BOUND('',#1061,.T.);
#524=FACE_OUTER_BOUND('',#1062,.T.);
#525=FACE_OUTER_BOUND('',#1063,.T.);
#526=FACE_OUTER_BOUND('',#1064,.T.);
#527=FACE_OUTER_BOUND('',#1065,.T.);
#528=FACE_OUTER_BOUND('',#1066,.T.);
#529=FACE_OUTER_BOUND('',#1067,.T.);
#530=FACE_OUTER_BOUND('',#1068,.T.);
#531=FACE_OUTER_BOUND('',#1069,.T.);
#532=FACE_OUTER_BOUND('',#1070,.T.);
#533=FACE_OUTER_BOUND('',#1071,.T.);
#534=FACE_OUTER_BOUND('',#1072,.T.);
#535=FACE_OUTER_BOUND('',#1073,.T.);
#536=FACE_OUTER_BOUND('',#1074,.T.);
#537=FACE_OUTER_BOUND('',#1075,.T.);
#538=FACE_OUTER_BOUND('',#1076,.T.);
#539=FACE_OUTER_BOUND('',#1077,.T.);
#540=FACE_OUTER_BOUND('',#1078,.T.);
#541=FACE_OUTER_BOUND('',#1079,.T.);
#542=FACE_OUTER_BOUND('',#1080,.T.);
#543=FACE_OUTER_BOUND('',#1081,.T.);
#544=FACE_OUTER_BOUND('',#1082,.T.);
#545=FACE_OUTER_BOUND('',#1086,.T.);
#546=FACE_OUTER_BOUND('',#1088,.T.);
#547=FACE_OUTER_BOUND('',#1089,.T.);
#548=FACE_OUTER_BOUND('',#1090,.T.);
#549=FACE_OUTER_BOUND('',#1092,.T.);
#550=FACE_OUTER_BOUND('',#1093,.T.);
#551=FACE_OUTER_BOUND('',#1094,.T.);
#552=FACE_OUTER_BOUND('',#1096,.T.);
#553=FACE_OUTER_BOUND('',#1097,.T.);
#554=FACE_OUTER_BOUND('',#1098,.T.);
#555=FACE_OUTER_BOUND('',#1099,.T.);
#556=FACE_OUTER_BOUND('',#1100,.T.);
#557=FACE_OUTER_BOUND('',#1101,.T.);
#558=FACE_OUTER_BOUND('',#1102,.T.);
#559=FACE_OUTER_BOUND('',#1103,.T.);
#560=FACE_OUTER_BOUND('',#1104,.T.);
#561=FACE_OUTER_BOUND('',#1105,.T.);
#562=FACE_OUTER_BOUND('',#1106,.T.);
#563=FACE_OUTER_BOUND('',#1107,.T.);
#564=FACE_OUTER_BOUND('',#1108,.T.);
#565=FACE_OUTER_BOUND('',#1109,.T.);
#566=FACE_OUTER_BOUND('',#1110,.T.);
#567=FACE_OUTER_BOUND('',#1111,.T.);
#568=FACE_OUTER_BOUND('',#1112,.T.);
#569=FACE_OUTER_BOUND('',#1113,.T.);
#570=FACE_OUTER_BOUND('',#1114,.T.);
#571=FACE_OUTER_BOUND('',#1115,.T.);
#572=FACE_OUTER_BOUND('',#1116,.T.);
#573=FACE_OUTER_BOUND('',#1117,.T.);
#574=FACE_OUTER_BOUND('',#1118,.T.);
#575=FACE_OUTER_BOUND('',#1119,.T.);
#576=FACE_OUTER_BOUND('',#1120,.T.);
#577=FACE_OUTER_BOUND('',#1121,.T.);
#578=FACE_OUTER_BOUND('',#1122,.T.);
#579=FACE_OUTER_BOUND('',#1123,.T.);
#580=FACE_OUTER_BOUND('',#1124,.T.);
#581=FACE_OUTER_BOUND('',#1125,.T.);
#582=FACE_OUTER_BOUND('',#1126,.T.);
#583=FACE_OUTER_BOUND('',#1127,.T.);
#584=FACE_OUTER_BOUND('',#1129,.T.);
#585=FACE_OUTER_BOUND('',#1130,.T.);
#586=FACE_OUTER_BOUND('',#1131,.T.);
#587=FACE_OUTER_BOUND('',#1132,.T.);
#588=FACE_OUTER_BOUND('',#1134,.T.);
#589=FACE_OUTER_BOUND('',#1135,.T.);
#590=FACE_OUTER_BOUND('',#1136,.T.);
#591=FACE_OUTER_BOUND('',#1138,.T.);
#592=FACE_OUTER_BOUND('',#1139,.T.);
#593=FACE_OUTER_BOUND('',#1140,.T.);
#594=FACE_OUTER_BOUND('',#1141,.T.);
#595=FACE_OUTER_BOUND('',#1142,.T.);
#596=FACE_OUTER_BOUND('',#1144,.T.);
#597=FACE_OUTER_BOUND('',#1145,.T.);
#598=FACE_OUTER_BOUND('',#1151,.T.);
#977=EDGE_LOOP('',(#5986,#5987,#5988,#5989,#5990,#5991,#5992,#5993));
#978=EDGE_LOOP('',(#5994,#5995,#5996,#5997));
#979=EDGE_LOOP('',(#5998,#5999,#6000,#6001));
#980=EDGE_LOOP('',(#6002,#6003,#6004,#6005));
#981=EDGE_LOOP('',(#6006,#6007,#6008,#6009));
#982=EDGE_LOOP('',(#6010,#6011,#6012,#6013));
#983=EDGE_LOOP('',(#6014,#6015,#6016,#6017));
#984=EDGE_LOOP('',(#6018,#6019,#6020,#6021));
#985=EDGE_LOOP('',(#6022,#6023,#6024,#6025));
#986=EDGE_LOOP('',(#6026,#6027,#6028,#6029));
#987=EDGE_LOOP('',(#6030,#6031,#6032,#6033));
#988=EDGE_LOOP('',(#6034,#6035,#6036,#6037));
#989=EDGE_LOOP('',(#6038,#6039,#6040,#6041));
#990=EDGE_LOOP('',(#6042,#6043,#6044,#6045));
#991=EDGE_LOOP('',(#6046,#6047,#6048,#6049));
#992=EDGE_LOOP('',(#6050,#6051,#6052,#6053));
#993=EDGE_LOOP('',(#6054,#6055,#6056,#6057));
#994=EDGE_LOOP('',(#6058,#6059,#6060,#6061));
#995=EDGE_LOOP('',(#6062,#6063,#6064,#6065));
#996=EDGE_LOOP('',(#6066,#6067,#6068,#6069));
#997=EDGE_LOOP('',(#6070,#6071,#6072,#6073));
#998=EDGE_LOOP('',(#6074,#6075,#6076,#6077));
#999=EDGE_LOOP('',(#6078,#6079,#6080,#6081));
#1000=EDGE_LOOP('',(#6082,#6083,#6084,#6085));
#1001=EDGE_LOOP('',(#6086,#6087,#6088,#6089));
#1002=EDGE_LOOP('',(#6090,#6091,#6092,#6093,#6094,#6095,#6096,#6097));
#1003=EDGE_LOOP('',(#6098,#6099,#6100,#6101));
#1004=EDGE_LOOP('',(#6102,#6103,#6104,#6105));
#1005=EDGE_LOOP('',(#6106,#6107,#6108,#6109));
#1006=EDGE_LOOP('',(#6110,#6111,#6112,#6113));
#1007=EDGE_LOOP('',(#6114,#6115,#6116,#6117));
#1008=EDGE_LOOP('',(#6118,#6119,#6120,#6121));
#1009=EDGE_LOOP('',(#6122,#6123,#6124,#6125));
#1010=EDGE_LOOP('',(#6126,#6127,#6128,#6129));
#1011=EDGE_LOOP('',(#6130,#6131,#6132,#6133));
#1012=EDGE_LOOP('',(#6134,#6135,#6136,#6137));
#1013=EDGE_LOOP('',(#6138,#6139,#6140,#6141));
#1014=EDGE_LOOP('',(#6142,#6143,#6144,#6145));
#1015=EDGE_LOOP('',(#6146,#6147,#6148,#6149));
#1016=EDGE_LOOP('',(#6150,#6151,#6152,#6153));
#1017=EDGE_LOOP('',(#6154,#6155,#6156,#6157));
#1018=EDGE_LOOP('',(#6158,#6159,#6160,#6161));
#1019=EDGE_LOOP('',(#6162,#6163,#6164,#6165));
#1020=EDGE_LOOP('',(#6166,#6167,#6168,#6169));
#1021=EDGE_LOOP('',(#6170,#6171,#6172,#6173));
#1022=EDGE_LOOP('',(#6174,#6175,#6176,#6177));
#1023=EDGE_LOOP('',(#6178,#6179,#6180,#6181));
#1024=EDGE_LOOP('',(#6182,#6183,#6184,#6185));
#1025=EDGE_LOOP('',(#6186,#6187,#6188,#6189));
#1026=EDGE_LOOP('',(#6190,#6191,#6192,#6193));
#1027=EDGE_LOOP('',(#6194,#6195,#6196,#6197,#6198,#6199,#6200,#6201));
#1028=EDGE_LOOP('',(#6202,#6203,#6204,#6205));
#1029=EDGE_LOOP('',(#6206,#6207,#6208,#6209));
#1030=EDGE_LOOP('',(#6210,#6211,#6212,#6213));
#1031=EDGE_LOOP('',(#6214,#6215,#6216,#6217));
#1032=EDGE_LOOP('',(#6218,#6219,#6220,#6221));
#1033=EDGE_LOOP('',(#6222,#6223,#6224,#6225));
#1034=EDGE_LOOP('',(#6226,#6227,#6228,#6229));
#1035=EDGE_LOOP('',(#6230,#6231,#6232,#6233));
#1036=EDGE_LOOP('',(#6234,#6235,#6236,#6237));
#1037=EDGE_LOOP('',(#6238,#6239,#6240,#6241));
#1038=EDGE_LOOP('',(#6242,#6243,#6244,#6245));
#1039=EDGE_LOOP('',(#6246,#6247,#6248,#6249));
#1040=EDGE_LOOP('',(#6250,#6251,#6252,#6253));
#1041=EDGE_LOOP('',(#6254,#6255,#6256,#6257));
#1042=EDGE_LOOP('',(#6258,#6259,#6260,#6261));
#1043=EDGE_LOOP('',(#6262,#6263,#6264,#6265));
#1044=EDGE_LOOP('',(#6266,#6267,#6268,#6269));
#1045=EDGE_LOOP('',(#6270,#6271,#6272,#6273));
#1046=EDGE_LOOP('',(#6274,#6275,#6276,#6277));
#1047=EDGE_LOOP('',(#6278,#6279,#6280,#6281));
#1048=EDGE_LOOP('',(#6282,#6283,#6284,#6285));
#1049=EDGE_LOOP('',(#6286,#6287,#6288,#6289));
#1050=EDGE_LOOP('',(#6290,#6291,#6292,#6293));
#1051=EDGE_LOOP('',(#6294,#6295,#6296,#6297));
#1052=EDGE_LOOP('',(#6298,#6299,#6300,#6301,#6302,#6303,#6304,#6305));
#1053=EDGE_LOOP('',(#6306,#6307,#6308,#6309));
#1054=EDGE_LOOP('',(#6310,#6311,#6312,#6313));
#1055=EDGE_LOOP('',(#6314,#6315,#6316,#6317));
#1056=EDGE_LOOP('',(#6318,#6319,#6320,#6321));
#1057=EDGE_LOOP('',(#6322,#6323,#6324,#6325));
#1058=EDGE_LOOP('',(#6326,#6327,#6328,#6329));
#1059=EDGE_LOOP('',(#6330,#6331,#6332,#6333));
#1060=EDGE_LOOP('',(#6334,#6335,#6336,#6337));
#1061=EDGE_LOOP('',(#6338,#6339,#6340,#6341));
#1062=EDGE_LOOP('',(#6342,#6343,#6344,#6345));
#1063=EDGE_LOOP('',(#6346,#6347,#6348,#6349));
#1064=EDGE_LOOP('',(#6350,#6351,#6352,#6353));
#1065=EDGE_LOOP('',(#6354,#6355,#6356,#6357));
#1066=EDGE_LOOP('',(#6358,#6359,#6360,#6361));
#1067=EDGE_LOOP('',(#6362,#6363,#6364,#6365));
#1068=EDGE_LOOP('',(#6366,#6367,#6368,#6369));
#1069=EDGE_LOOP('',(#6370,#6371,#6372,#6373));
#1070=EDGE_LOOP('',(#6374,#6375,#6376,#6377));
#1071=EDGE_LOOP('',(#6378,#6379,#6380,#6381));
#1072=EDGE_LOOP('',(#6382,#6383,#6384,#6385));
#1073=EDGE_LOOP('',(#6386,#6387,#6388,#6389));
#1074=EDGE_LOOP('',(#6390,#6391,#6392,#6393));
#1075=EDGE_LOOP('',(#6394,#6395,#6396,#6397));
#1076=EDGE_LOOP('',(#6398,#6399,#6400,#6401));
#1077=EDGE_LOOP('',(#6402,#6403,#6404,#6405));
#1078=EDGE_LOOP('',(#6406,#6407,#6408,#6409));
#1079=EDGE_LOOP('',(#6410,#6411,#6412,#6413));
#1080=EDGE_LOOP('',(#6414,#6415,#6416,#6417));
#1081=EDGE_LOOP('',(#6418,#6419,#6420,#6421));
#1082=EDGE_LOOP('',(#6422,#6423,#6424,#6425,#6426,#6427,#6428,#6429));
#1083=EDGE_LOOP('',(#6430));
#1084=EDGE_LOOP('',(#6431));
#1085=EDGE_LOOP('',(#6432));
#1086=EDGE_LOOP('',(#6433,#6434,#6435,#6436));
#1087=EDGE_LOOP('',(#6437));
#1088=EDGE_LOOP('',(#6438,#6439,#6440,#6441));
#1089=EDGE_LOOP('',(#6442,#6443,#6444,#6445));
#1090=EDGE_LOOP('',(#6446));
#1091=EDGE_LOOP('',(#6447));
#1092=EDGE_LOOP('',(#6448,#6449,#6450,#6451));
#1093=EDGE_LOOP('',(#6452,#6453,#6454,#6455));
#1094=EDGE_LOOP('',(#6456));
#1095=EDGE_LOOP('',(#6457));
#1096=EDGE_LOOP('',(#6458,#6459,#6460,#6461));
#1097=EDGE_LOOP('',(#6462,#6463,#6464,#6465));
#1098=EDGE_LOOP('',(#6466,#6467,#6468,#6469));
#1099=EDGE_LOOP('',(#6470,#6471,#6472,#6473));
#1100=EDGE_LOOP('',(#6474,#6475,#6476,#6477,#6478,#6479,#6480,#6481,#6482,
#6483,#6484,#6485,#6486,#6487,#6488,#6489,#6490,#6491,#6492,#6493,#6494,
#6495,#6496,#6497,#6498,#6499,#6500,#6501,#6502,#6503));
#1101=EDGE_LOOP('',(#6504,#6505,#6506,#6507,#6508,#6509,#6510,#6511,#6512,
#6513,#6514,#6515,#6516,#6517,#6518,#6519,#6520,#6521,#6522,#6523,#6524,
#6525,#6526,#6527,#6528,#6529,#6530,#6531,#6532));
#1102=EDGE_LOOP('',(#6533,#6534,#6535,#6536));
#1103=EDGE_LOOP('',(#6537,#6538,#6539,#6540));
#1104=EDGE_LOOP('',(#6541,#6542,#6543,#6544));
#1105=EDGE_LOOP('',(#6545,#6546,#6547,#6548,#6549,#6550,#6551,#6552,#6553,
#6554,#6555,#6556,#6557,#6558,#6559,#6560,#6561,#6562,#6563,#6564,#6565,
#6566,#6567,#6568,#6569,#6570,#6571,#6572,#6573,#6574));
#1106=EDGE_LOOP('',(#6575,#6576,#6577,#6578,#6579,#6580,#6581,#6582,#6583,
#6584,#6585,#6586,#6587,#6588,#6589,#6590,#6591,#6592,#6593,#6594,#6595,
#6596,#6597,#6598,#6599,#6600,#6601,#6602,#6603));
#1107=EDGE_LOOP('',(#6604,#6605,#6606,#6607));
#1108=EDGE_LOOP('',(#6608,#6609,#6610,#6611));
#1109=EDGE_LOOP('',(#6612,#6613,#6614,#6615));
#1110=EDGE_LOOP('',(#6616,#6617,#6618,#6619,#6620,#6621,#6622,#6623,#6624,
#6625,#6626,#6627,#6628,#6629,#6630,#6631,#6632,#6633,#6634,#6635,#6636,
#6637,#6638,#6639,#6640,#6641,#6642,#6643,#6644,#6645));
#1111=EDGE_LOOP('',(#6646,#6647,#6648,#6649,#6650,#6651,#6652,#6653,#6654,
#6655,#6656,#6657,#6658,#6659,#6660,#6661,#6662,#6663,#6664,#6665,#6666,
#6667,#6668,#6669,#6670,#6671,#6672,#6673,#6674));
#1112=EDGE_LOOP('',(#6675,#6676,#6677,#6678));
#1113=EDGE_LOOP('',(#6679,#6680,#6681,#6682));
#1114=EDGE_LOOP('',(#6683,#6684,#6685,#6686));
#1115=EDGE_LOOP('',(#6687,#6688,#6689,#6690,#6691,#6692,#6693,#6694,#6695,
#6696,#6697,#6698,#6699,#6700,#6701,#6702,#6703,#6704,#6705,#6706,#6707,
#6708,#6709,#6710,#6711,#6712,#6713,#6714,#6715,#6716));
#1116=EDGE_LOOP('',(#6717,#6718,#6719,#6720,#6721,#6722,#6723,#6724,#6725,
#6726,#6727,#6728,#6729,#6730,#6731,#6732,#6733,#6734,#6735,#6736,#6737,
#6738,#6739,#6740,#6741,#6742,#6743,#6744,#6745));
#1117=EDGE_LOOP('',(#6746,#6747,#6748,#6749));
#1118=EDGE_LOOP('',(#6750));
#1119=EDGE_LOOP('',(#6751));
#1120=EDGE_LOOP('',(#6752));
#1121=EDGE_LOOP('',(#6753));
#1122=EDGE_LOOP('',(#6754,#6755,#6756,#6757));
#1123=EDGE_LOOP('',(#6758,#6759,#6760,#6761));
#1124=EDGE_LOOP('',(#6762,#6763,#6764,#6765));
#1125=EDGE_LOOP('',(#6766,#6767,#6768,#6769));
#1126=EDGE_LOOP('',(#6770,#6771,#6772,#6773));
#1127=EDGE_LOOP('',(#6774,#6775,#6776,#6777));
#1128=EDGE_LOOP('',(#6778));
#1129=EDGE_LOOP('',(#6779,#6780,#6781,#6782));
#1130=EDGE_LOOP('',(#6783,#6784,#6785,#6786));
#1131=EDGE_LOOP('',(#6787,#6788,#6789,#6790));
#1132=EDGE_LOOP('',(#6791,#6792,#6793,#6794));
#1133=EDGE_LOOP('',(#6795));
#1134=EDGE_LOOP('',(#6796,#6797,#6798,#6799));
#1135=EDGE_LOOP('',(#6800,#6801,#6802,#6803));
#1136=EDGE_LOOP('',(#6804));
#1137=EDGE_LOOP('',(#6805));
#1138=EDGE_LOOP('',(#6806,#6807,#6808,#6809));
#1139=EDGE_LOOP('',(#6810));
#1140=EDGE_LOOP('',(#6811,#6812,#6813,#6814));
#1141=EDGE_LOOP('',(#6815,#6816,#6817,#6818,#6819,#6820,#6821,#6822));
#1142=EDGE_LOOP('',(#6823,#6824,#6825,#6826));
#1143=EDGE_LOOP('',(#6827));
#1144=EDGE_LOOP('',(#6828,#6829,#6830,#6831,#6832,#6833,#6834,#6835));
#1145=EDGE_LOOP('',(#6836,#6837,#6838,#6839));
#1146=EDGE_LOOP('',(#6840,#6841,#6842,#6843));
#1147=EDGE_LOOP('',(#6844,#6845,#6846,#6847));
#1148=EDGE_LOOP('',(#6848,#6849,#6850,#6851));
#1149=EDGE_LOOP('',(#6852,#6853,#6854,#6855));
#1150=EDGE_LOOP('',(#6856,#6857,#6858,#6859,#6860,#6861,#6862,#6863));
#1151=EDGE_LOOP('',(#6864,#6865,#6866,#6867,#6868,#6869,#6870,#6871,#6872,
#6873,#6874,#6875));
#1152=EDGE_LOOP('',(#6876));
#1153=EDGE_LOOP('',(#6877));
#1154=EDGE_LOOP('',(#6878));
#1155=EDGE_LOOP('',(#6879));
#1582=CIRCLE('',#9975,0.1666);
#1583=CIRCLE('',#9976,0.1666);
#1584=CIRCLE('',#9988,0.1666);
#1585=CIRCLE('',#9990,0.205475);
#1586=CIRCLE('',#10003,0.205475);
#1587=CIRCLE('',#10005,0.1666);
#1588=CIRCLE('',#10006,0.1666);
#1589=CIRCLE('',#10018,0.1666);
#1590=CIRCLE('',#10020,0.205475000000001);
#1591=CIRCLE('',#10033,0.205475000000001);
#1592=CIRCLE('',#10035,0.1666);
#1593=CIRCLE('',#10036,0.1666);
#1594=CIRCLE('',#10048,0.1666);
#1595=CIRCLE('',#10050,0.205475000000001);
#1596=CIRCLE('',#10063,0.205475000000001);
#1597=CIRCLE('',#10065,0.1666);
#1598=CIRCLE('',#10066,0.1666);
#1599=CIRCLE('',#10078,0.1666);
#1600=CIRCLE('',#10080,0.205475);
#1601=CIRCLE('',#10093,0.205475);
#1602=CIRCLE('',#10095,0.2);
#1603=CIRCLE('',#10096,0.2);
#1604=CIRCLE('',#10099,0.2);
#1605=CIRCLE('',#10100,0.2);
#1606=CIRCLE('',#10103,0.2);
#1607=CIRCLE('',#10104,0.2);
#1608=CIRCLE('',#10106,0.2);
#1609=CIRCLE('',#10107,0.8);
#1610=CIRCLE('',#10108,0.25);
#1611=CIRCLE('',#10109,0.25);
#1612=CIRCLE('',#10111,0.6);
#1613=CIRCLE('',#10113,0.2);
#1614=CIRCLE('',#10115,0.6);
#1615=CIRCLE('',#10117,0.4);
#1616=CIRCLE('',#10118,0.25);
#1617=CIRCLE('',#10120,0.4);
#1618=CIRCLE('',#10123,0.4);
#1619=CIRCLE('',#10124,0.25);
#1620=CIRCLE('',#10126,0.4);
#1621=CIRCLE('',#10145,0.3);
#1622=CIRCLE('',#10146,0.3);
#1623=CIRCLE('',#10148,0.3);
#1624=CIRCLE('',#10149,0.3);
#1625=CIRCLE('',#10159,0.65);
#1626=CIRCLE('',#10160,0.65);
#1627=CIRCLE('',#10162,0.8);
#1738=B_SPLINE_CURVE_WITH_KNOTS('',3,(#12707,#12708,#12709,#12710,#12711,
#12712,#12713,#12714,#12715,#12716,#12717,#12718,#12719,#12720,#12721,#12722,
#12723,#12724,#12725,#12726,#12727,#12728),.UNSPECIFIED.,.F.,.F.,(4,3,3,
3,3,3,3,4),(76.708045941327,76.8129957196859,77.8105670926688,78.8081384656518,
79.8057098386347,80.8032812116176,81.8008525846006,82.7984239575835),
 .UNSPECIFIED.);
#1739=B_SPLINE_CURVE_WITH_KNOTS('',3,(#12732,#12733,#12734,#12735,#12736,
#12737,#12738),.UNSPECIFIED.,.F.,.F.,(4,3,4),(-80.783811092309,-79.8057098386347,
-79.2446069498473),.UNSPECIFIED.);
#1740=B_SPLINE_CURVE_WITH_KNOTS('',3,(#12742,#12743,#12744,#12745,#12746,
#12747,#12748,#12749,#12750,#12751,#12752,#12753,#12754,#12755,#12756,#12757,
#12758,#12759,#12760,#12761,#12762,#12763),.UNSPECIFIED.,.F.,.F.,(4,3,3,
3,3,3,3,4),(-79.2446069498473,-78.8081384656518,-77.8105670926688,-76.8129957196859,
-75.815424346703,-74.81785297372,-73.8202816007371,-72.9614216426678),
 .UNSPECIFIED.);
#1741=B_SPLINE_CURVE_WITH_KNOTS('',3,(#12768,#12769,#12770,#12771,#12772,
#12773,#12774,#12775,#12776,#12777,#12778,#12779,#12780,#12781,#12782,#12783,
#12784,#12785,#12786,#12787,#12788,#12789),.UNSPECIFIED.,.F.,.F.,(4,3,3,
3,3,3,3,4),(70.4248606341475,70.8275674817883,71.8251388547712,72.8227102277542,
73.8202816007371,74.81785297372,75.815424346703,76.708045941327),
 .UNSPECIFIED.);
#1742=B_SPLINE_CURVE_WITH_KNOTS('',3,(#12790,#12791,#12792,#12793,#12794,
#12795,#12796,#12797,#12798,#12799,#12800,#12801,#12802,#12803,#12804,#12805,
#12806,#12807,#12808,#12809,#12810,#12811,#12812,#12813,#12814),
 .UNSPECIFIED.,.F.,.F.,(4,3,3,3,3,3,3,3,4),(-72.9614216426678,-72.8227102277542,
-71.8251388547712,-70.8275674817883,-69.8299961088054,-68.8324247358224,
-67.8348533628395,-66.8372819898566,-66.6782363354882),.UNSPECIFIED.);
#1743=B_SPLINE_CURVE_WITH_KNOTS('',3,(#12819,#12820,#12821,#12822,#12823,
#12824,#12825,#12826,#12827,#12828,#12829,#12830,#12831,#12832,#12833,#12834,
#12835,#12836,#12837,#12838,#12839,#12840),.UNSPECIFIED.,.F.,.F.,(4,3,3,
3,3,3,3,4),(64.1416753269678,64.8421392438907,65.8397106168736,66.8372819898565,
67.8348533628395,68.8324247358224,69.8299961088054,70.4248606341475),
 .UNSPECIFIED.);
#1744=B_SPLINE_CURVE_WITH_KNOTS('',3,(#12841,#12842,#12843,#12844,#12845,
#12846,#12847,#12848,#12849,#12850,#12851,#12852,#12853,#12854,#12855,#12856,
#12857,#12858,#12859,#12860,#12861,#12862),.UNSPECIFIED.,.F.,.F.,(4,3,3,
3,3,3,3,4),(-66.6782363354882,-65.8397106168736,-64.8421392438907,-63.8445678709078,
-62.8469964979248,-61.8494251249419,-60.851853751959,-60.3950510283085),
 .UNSPECIFIED.);
#1745=B_SPLINE_CURVE_WITH_KNOTS('',3,(#12867,#12868,#12869,#12870,#12871,
#12872,#12873,#12874,#12875,#12876,#12877,#12878,#12879,#12880,#12881,#12882,
#12883,#12884,#12885,#12886,#12887,#12888),.UNSPECIFIED.,.F.,.F.,(4,3,3,
3,3,3,3,4),(57.8584900197882,58.8567110059931,59.854282378976,60.8518537519589,
61.8494251249419,62.8469964979248,63.8445678709078,64.1416753269678),
 .UNSPECIFIED.);
#1746=B_SPLINE_CURVE_WITH_KNOTS('',3,(#12889,#12890,#12891,#12892,#12893,
#12894,#12895,#12896,#12897,#12898,#12899,#12900,#12901,#12902,#12903,#12904,
#12905,#12906,#12907,#12908,#12909,#12910),.UNSPECIFIED.,.F.,.F.,(4,3,3,
3,3,3,3,4),(-60.3950510283085,-59.854282378976,-58.8567110059931,-57.8591396330102,
-56.8615682600272,-55.8639968870443,-54.8664255140614,-54.1118657211289),
 .UNSPECIFIED.);
#1747=B_SPLINE_CURVE_WITH_KNOTS('',3,(#12915,#12916,#12917,#12918,#12919,
#12920,#12921,#12922,#12923,#12924,#12925,#12926,#12927,#12928,#12929,#12930,
#12931,#12932,#12933,#12934,#12935,#12936),.UNSPECIFIED.,.F.,.F.,(4,3,3,
3,3,3,3,4),(51.5753047126087,51.8737113951126,52.8712827680955,53.8688541410784,
54.8664255140614,55.8639968870443,56.8615682600272,57.8584900197882),
 .UNSPECIFIED.);
#1748=B_SPLINE_CURVE_WITH_KNOTS('',3,(#12937,#12938,#12939,#12940,#12941,
#12942,#12943,#12944,#12945,#12946,#12947,#12948,#12949,#12950,#12951,#12952,
#12953,#12954,#12955,#12956,#12957,#12958,#12959,#12960,#12961),
 .UNSPECIFIED.,.F.,.F.,(4,3,3,3,3,3,3,3,4),(-54.1118657211289,-53.8688541410784,
-52.8712827680955,-51.8737113951126,-50.8761400221296,-49.8785686491467,
-48.8809972761638,-47.8834259031808,-47.8286804139493),.UNSPECIFIED.);
#1749=B_SPLINE_CURVE_WITH_KNOTS('',3,(#12966,#12967,#12968,#12969,#12970,
#12971,#12972,#12973,#12974,#12975,#12976,#12977,#12978,#12979,#12980,#12981,
#12982,#12983,#12984,#12985,#12986,#12987),.UNSPECIFIED.,.F.,.F.,(4,3,3,
3,3,3,3,4),(45.2921194054291,45.888283157215,46.8858545301979,47.8834259031808,
48.8809972761637,49.8785686491467,50.8761400221296,51.5753047126087),
 .UNSPECIFIED.);
#1750=B_SPLINE_CURVE_WITH_KNOTS('',3,(#12988,#12989,#12990,#12991,#12992,
#12993,#12994,#12995,#12996,#12997,#12998,#12999,#13000,#13001,#13002,#13003,
#13004,#13005,#13006,#13007,#13008,#13009),.UNSPECIFIED.,.F.,.F.,(4,3,3,
3,3,3,3,4),(-47.8286804139493,-46.8858545301979,-45.888283157215,-44.890711784232,
-43.8931404112491,-42.8955690382662,-41.8979976652832,-41.5454951067698),
 .UNSPECIFIED.);
#1751=B_SPLINE_CURVE_WITH_KNOTS('',3,(#13014,#13015,#13016,#13017,#13018,
#13019,#13020,#13021,#13022,#13023,#13024,#13025,#13026,#13027,#13028,#13029,
#13030,#13031,#13032,#13033,#13034,#13035),.UNSPECIFIED.,.F.,.F.,(4,3,3,
3,3,3,3,4),(39.0089340982495,39.9028549193174,40.9004262923003,41.8979976652832,
42.8955690382662,43.8931404112491,44.890711784232,45.2921194054291),
 .UNSPECIFIED.);
#1752=B_SPLINE_CURVE_WITH_KNOTS('',3,(#13036,#13037,#13038,#13039,#13040,
#13041,#13042,#13043,#13044,#13045,#13046,#13047,#13048,#13049,#13050,#13051,
#13052,#13053,#13054,#13055,#13056,#13057),.UNSPECIFIED.,.F.,.F.,(4,3,3,
3,3,3,3,4),(-41.5454951067698,-40.9004262923003,-39.9028549193174,-38.9052835463344,
-37.9077121733515,-36.9101408003686,-35.9125694273856,-35.2623097995902),
 .UNSPECIFIED.);
#1753=B_SPLINE_CURVE_WITH_KNOTS('',3,(#13062,#13063,#13064,#13065,#13066,
#13067,#13068,#13069,#13070,#13071,#13072,#13073,#13074,#13075,#13076,#13077,
#13078,#13079,#13080,#13081,#13082,#13083,#13084,#13085,#13086),
 .UNSPECIFIED.,.F.,.F.,(4,3,3,3,3,3,3,3,4),(32.7257487910699,32.9198553084368,
33.9174266814197,34.9149980544027,35.9125694273856,36.9101408003685,37.9077121733515,
38.9052835463344,39.0089340982495),.UNSPECIFIED.);
#1754=B_SPLINE_CURVE_WITH_KNOTS('',3,(#13087,#13088,#13089,#13090,#13091,
#13092,#13093,#13094,#13095,#13096,#13097,#13098,#13099,#13100,#13101,#13102,
#13103,#13104,#13105,#13106,#13107,#13108),.UNSPECIFIED.,.F.,.F.,(4,3,3,
3,3,3,3,4),(-35.2623097995902,-34.9149980544027,-33.9174266814198,-32.9198553084368,
-31.9222839354539,-30.924712562471,-29.927141189488,-28.9791244924106),
 .UNSPECIFIED.);
#1755=B_SPLINE_CURVE_WITH_KNOTS('',3,(#13113,#13114,#13115,#13116,#13117,
#13118,#13119,#13120,#13121,#13122,#13123,#13124,#13125,#13126,#13127,#13128,
#13129,#13130,#13131,#13132,#13133,#13134),.UNSPECIFIED.,.F.,.F.,(4,3,3,
3,3,3,3,4),(26.4425634838903,26.9344270705392,27.9319984435221,28.9295698165051,
29.927141189488,30.9247125624709,31.9222839354539,32.7257487910699),
 .UNSPECIFIED.);
#1756=B_SPLINE_CURVE_WITH_KNOTS('',3,(#13135,#13136,#13137,#13138,#13139,
#13140,#13141,#13142,#13143,#13144,#13145,#13146,#13147,#13148,#13149,#13150,
#13151,#13152,#13153,#13154,#13155,#13156,#13157,#13158,#13159),
 .UNSPECIFIED.,.F.,.F.,(4,3,3,3,3,3,3,3,4),(-28.9791244924106,-28.9295698165051,
-27.9319984435222,-26.9344270705392,-25.9368556975563,-24.9392843245734,
-23.9417129515904,-22.9441415786075,-22.695939185231),.UNSPECIFIED.);
#1757=B_SPLINE_CURVE_WITH_KNOTS('',3,(#13164,#13165,#13166,#13167,#13168,
#13169,#13170,#13171,#13172,#13173,#13174,#13175,#13176,#13177,#13178,#13179,
#13180,#13181,#13182,#13183,#13184,#13185),.UNSPECIFIED.,.F.,.F.,(4,3,3,
3,3,3,3,4),(20.1593781767107,20.9489988326416,21.9465702056245,22.9441415786075,
23.9417129515904,24.9392843245733,25.9368556975563,26.4425634838903),
 .UNSPECIFIED.);
#1758=B_SPLINE_CURVE_WITH_KNOTS('',3,(#13186,#13187,#13188,#13189,#13190,
#13191,#13192,#13193,#13194,#13195,#13196,#13197,#13198,#13199,#13200,#13201,
#13202,#13203,#13204,#13205,#13206,#13207),.UNSPECIFIED.,.F.,.F.,(4,3,3,
3,3,3,3,4),(-22.695939185231,-21.9465702056245,-20.9489988326416,-19.9514274596587,
-18.9538560866757,-17.9562847136928,-16.9587133407099,-16.4127538780514),
 .UNSPECIFIED.);
#1759=B_SPLINE_CURVE_WITH_KNOTS('',3,(#13212,#13213,#13214,#13215,#13216,
#13217,#13218,#13219,#13220,#13221,#13222,#13223,#13224,#13225,#13226,#13227,
#13228,#13229,#13230,#13231,#13232,#13233,#13234,#13235,#13236),
 .UNSPECIFIED.,.F.,.F.,(4,3,3,3,3,3,3,3,4),(13.8761928695311,13.9659992217611,
14.963570594744,15.9611419677269,16.9587133407099,17.9562847136928,18.9538560866757,
19.9514274596587,20.1593781767107),.UNSPECIFIED.);
#1760=B_SPLINE_CURVE_WITH_KNOTS('',3,(#13237,#13238,#13239,#13240,#13241,
#13242,#13243,#13244,#13245,#13246,#13247,#13248,#13249,#13250,#13251,#13252,
#13253,#13254,#13255,#13256,#13257,#13258),.UNSPECIFIED.,.F.,.F.,(4,3,3,
3,3,3,3,4),(-16.4127538780514,-15.9611419677269,-14.963570594744,-13.9659992217611,
-12.9684278487781,-11.9708564757952,-10.9732851028123,-10.1295685708718),
 .UNSPECIFIED.);
#1761=B_SPLINE_CURVE_WITH_KNOTS('',3,(#13264,#13265,#13266,#13267,#13268,
#13269,#13270,#13271,#13272,#13273,#13274,#13275,#13276),.UNSPECIFIED.,
 .F.,.F.,(4,3,3,3,4),(-3.84638326369226,-2.9927141189488,-1.99514274596587,
-0.997571372982934,0.),.UNSPECIFIED.);
#1762=B_SPLINE_CURVE_WITH_KNOTS('',3,(#13279,#13280,#13281,#13282,#13283,
#13284,#13285,#13286,#13287,#13288,#13289,#13290,#13291,#13292,#13293,#13294,
#13295,#13296,#13297),.UNSPECIFIED.,.F.,.F.,(4,3,3,3,3,3,4),(2.01461286527449,
2.9927141189488,3.99028549193174,4.98785686491467,5.9854282378976,6.98299961088054,
7.59300756235157),.UNSPECIFIED.);
#1763=B_SPLINE_CURVE_WITH_KNOTS('',3,(#13303,#13304,#13305,#13306,#13307,
#13308,#13309),.UNSPECIFIED.,.F.,.F.,(4,1,1,1,4),(91.106186954104,91.6672898428914,
92.6648612158743,93.6624325888573,94.6600039618402),.UNSPECIFIED.);
#1764=B_SPLINE_CURVE_WITH_KNOTS('',3,(#13312,#13313,#13314,#13315,#13316,
#13317,#13318,#13319),.UNSPECIFIED.,.F.,.F.,(4,1,1,1,1,4),(91.106186954104,
91.2111367324628,92.2087081054457,93.2062794784287,94.2038508514116,95.1819521050859),
 .UNSPECIFIED.);
#1765=B_SPLINE_CURVE_WITH_KNOTS('',3,(#13324,#13325,#13326,#13327,#13328,
#13329,#13330,#13331,#13332,#13333),.UNSPECIFIED.,.F.,.F.,(4,1,1,1,1,1,
1,4),(84.8230016469245,85.6818616049938,86.6794329779767,87.6770043509596,
88.6745757239426,89.6721470969255,90.6697184699085,91.106186954104),
 .UNSPECIFIED.);
#1766=B_SPLINE_CURVE_WITH_KNOTS('',3,(#13334,#13335,#13336,#13337,#13338,
#13339,#13340,#13341,#13342,#13343),.UNSPECIFIED.,.F.,.F.,(4,1,1,1,1,1,
1,4),(84.8230016469244,85.2257084945652,86.2232798675481,87.2208512405311,
88.218422613514,89.2159939864969,90.2135653594799,91.106186954104),
 .UNSPECIFIED.);
#1767=B_SPLINE_CURVE_WITH_KNOTS('',3,(#13348,#13349,#13350,#13351,#13352,
#13353,#13354,#13355,#13356,#13357,#13358),.UNSPECIFIED.,.F.,.F.,(4,1,1,
1,1,1,1,1,4),(78.5398163397448,78.6988619941132,79.6964333670962,80.6940047400791,
81.6915761130621,82.689147486045,83.6867188590279,84.6842902320109,84.8230016469245),
 .UNSPECIFIED.);
#1768=B_SPLINE_CURVE_WITH_KNOTS('',3,(#13359,#13360,#13361,#13362,#13363,
#13364,#13365,#13366,#13367,#13368),.UNSPECIFIED.,.F.,.F.,(4,1,1,1,1,1,
1,4),(78.5398163397448,79.2402802566676,80.2378516296505,81.2354230026335,
82.2329943756164,83.2305657485993,84.2281371215823,84.8230016469244),
 .UNSPECIFIED.);
#1769=B_SPLINE_CURVE_WITH_KNOTS('',3,(#13373,#13374,#13375,#13376,#13377,
#13378,#13379,#13380,#13381,#13382),.UNSPECIFIED.,.F.,.F.,(4,1,1,1,1,1,
1,4),(72.2566310325652,72.7134337562156,73.7110051291986,74.7085765021815,
75.7061478751644,76.7037192481474,77.7012906211303,78.5398163397448),
 .UNSPECIFIED.);
#1770=B_SPLINE_CURVE_WITH_KNOTS('',3,(#13383,#13384,#13385,#13386,#13387,
#13388,#13389,#13390,#13391,#13392,#13393),.UNSPECIFIED.,.F.,.F.,(4,1,1,
1,1,1,1,1,4),(72.2566310325652,72.2572806457871,73.25485201877,74.2524233917529,
75.2499947647359,76.2475661377188,77.2451375107017,78.2427088836847,78.5398163397448),
 .UNSPECIFIED.);
#1771=B_SPLINE_CURVE_WITH_KNOTS('',3,(#13398,#13399,#13400,#13401,#13402,
#13403,#13404,#13405,#13406,#13407),.UNSPECIFIED.,.F.,.F.,(4,1,1,1,1,1,
1,4),(65.9734457253856,66.728005518318,67.725576891301,68.7231482642839,
69.7207196372669,70.7182910102498,71.7158623832327,72.2566310325652),
 .UNSPECIFIED.);
#1772=B_SPLINE_CURVE_WITH_KNOTS('',3,(#13408,#13409,#13410,#13411,#13412,
#13413,#13414,#13415,#13416,#13417),.UNSPECIFIED.,.F.,.F.,(4,1,1,1,1,1,
1,4),(65.9734457253856,66.2718524078895,67.2694237808724,68.2669951538553,
69.2645665268383,70.2621378998212,71.2597092728041,72.2566310325652),
 .UNSPECIFIED.);
#1773=B_SPLINE_CURVE_WITH_KNOTS('',3,(#13422,#13423,#13424,#13425,#13426,
#13427,#13428,#13429,#13430,#13431,#13432),.UNSPECIFIED.,.F.,.F.,(4,1,1,
1,1,1,1,1,4),(59.690260418206,59.7450059074375,60.7425772804204,61.7401486534034,
62.7377200263863,63.7352913993692,64.7328627723522,65.7304341453351,65.9734457253856),
 .UNSPECIFIED.);
#1774=B_SPLINE_CURVE_WITH_KNOTS('',3,(#13433,#13434,#13435,#13436,#13437,
#13438,#13439,#13440,#13441,#13442),.UNSPECIFIED.,.F.,.F.,(4,1,1,1,1,1,
1,4),(59.690260418206,60.2864241699919,61.2839955429748,62.2815669159577,
63.2791382889407,64.2767096619236,65.2742810349065,65.9734457253856),
 .UNSPECIFIED.);
#1775=B_SPLINE_CURVE_WITH_KNOTS('',3,(#13447,#13448,#13449,#13450,#13451,
#13452,#13453,#13454,#13455,#13456),.UNSPECIFIED.,.F.,.F.,(4,1,1,1,1,1,
1,4),(53.4070751110265,53.7595776695399,54.7571490425228,55.7547204155058,
56.7522917884887,57.7498631614716,58.7474345344546,59.690260418206),
 .UNSPECIFIED.);
#1776=B_SPLINE_CURVE_WITH_KNOTS('',3,(#13457,#13458,#13459,#13460,#13461,
#13462,#13463,#13464,#13465,#13466),.UNSPECIFIED.,.F.,.F.,(4,1,1,1,1,1,
1,4),(53.4070751110264,54.3009959320943,55.2985673050772,56.2961386780601,
57.2937100510431,58.291281424026,59.2888527970089,59.690260418206),
 .UNSPECIFIED.);
#1777=B_SPLINE_CURVE_WITH_KNOTS('',3,(#13471,#13472,#13473,#13474,#13475,
#13476,#13477,#13478,#13479,#13480),.UNSPECIFIED.,.F.,.F.,(4,1,1,1,1,1,
1,4),(47.1238898038469,47.7741494316423,48.7717208046252,49.7692921776082,
50.7668635505911,51.764434923574,52.762006296557,53.4070751110265),
 .UNSPECIFIED.);
#1778=B_SPLINE_CURVE_WITH_KNOTS('',3,(#13481,#13482,#13483,#13484,#13485,
#13486,#13487,#13488,#13489,#13490,#13491),.UNSPECIFIED.,.F.,.F.,(4,1,1,
1,1,1,1,1,4),(47.1238898038469,47.3179963212137,48.3155676941967,49.3131390671796,
50.3107104401625,51.3082818131455,52.3058531861284,53.3034245591113,53.4070751110264),
 .UNSPECIFIED.);
#1779=B_SPLINE_CURVE_WITH_KNOTS('',3,(#13496,#13497,#13498,#13499,#13500,
#13501,#13502,#13503,#13504,#13505),.UNSPECIFIED.,.F.,.F.,(4,1,1,1,1,1,
1,4),(40.8407044966673,41.7887211937447,42.7862925667276,43.7838639397106,
44.7814353126935,45.7790066856764,46.7765780586594,47.1238898038469),
 .UNSPECIFIED.);
#1780=B_SPLINE_CURVE_WITH_KNOTS('',3,(#13506,#13507,#13508,#13509,#13510,
#13511,#13512,#13513,#13514,#13515),.UNSPECIFIED.,.F.,.F.,(4,1,1,1,1,1,
1,4),(40.8407044966673,41.3325680833161,42.3301394562991,43.327710829282,
44.3252822022649,45.3228535752479,46.3204249482308,47.1238898038469),
 .UNSPECIFIED.);
#1781=B_SPLINE_CURVE_WITH_KNOTS('',3,(#13520,#13521,#13522,#13523,#13524,
#13525,#13526,#13527,#13528,#13529,#13530),.UNSPECIFIED.,.F.,.F.,(4,1,1,
1,1,1,1,1,4),(34.5575191894876,34.8057215828642,35.8032929558471,36.80086432883,
37.798435701813,38.7960070747959,39.7935784477788,40.7911498207618,40.8407044966673),
 .UNSPECIFIED.);
#1782=B_SPLINE_CURVE_WITH_KNOTS('',3,(#13531,#13532,#13533,#13534,#13535,
#13536,#13537,#13538,#13539,#13540),.UNSPECIFIED.,.F.,.F.,(4,1,1,1,1,1,
1,4),(34.5575191894876,35.3471398454185,36.3447112184015,37.3422825913844,
38.3398539643673,39.3374253373503,40.3349967103332,40.8407044966673),
 .UNSPECIFIED.);
#1783=B_SPLINE_CURVE_WITH_KNOTS('',3,(#13545,#13546,#13547,#13548,#13549,
#13550,#13551,#13552,#13553,#13554),.UNSPECIFIED.,.F.,.F.,(4,1,1,1,1,1,
1,4),(28.2743338823081,28.8202933449666,29.8178647179495,30.8154360909324,
31.8130074639154,32.8105788368983,33.8081502098812,34.5575191894876),
 .UNSPECIFIED.);
#1784=B_SPLINE_CURVE_WITH_KNOTS('',3,(#13555,#13556,#13557,#13558,#13559,
#13560,#13561,#13562,#13563,#13564,#13565),.UNSPECIFIED.,.F.,.F.,(4,1,1,
1,1,1,1,1,4),(28.2743338823081,28.364140234538,29.3617116075209,30.3592829805039,
31.3568543534868,32.3544257264697,33.3519970994527,34.3495684724356,34.5575191894876),
 .UNSPECIFIED.);
#1785=B_SPLINE_CURVE_WITH_KNOTS('',3,(#13570,#13571,#13572,#13573,#13574,
#13575,#13576,#13577,#13578,#13579),.UNSPECIFIED.,.F.,.F.,(4,1,1,1,1,1,
1,4),(21.9911485751285,22.834865107069,23.8324364800519,24.8300078530348,
25.8275792260178,26.8251505990007,27.8227219719836,28.2743338823081),
 .UNSPECIFIED.);
#1786=B_SPLINE_CURVE_WITH_KNOTS('',3,(#13580,#13581,#13582,#13583,#13584,
#13585,#13586,#13587,#13588,#13589),.UNSPECIFIED.,.F.,.F.,(4,1,1,1,1,1,
1,4),(21.9911485751285,22.3787119966404,23.3762833696233,24.3738547426063,
25.3714261155892,26.3689974885721,27.3665688615551,28.2743338823081),
 .UNSPECIFIED.);
#1787=B_SPLINE_CURVE_WITH_KNOTS('',3,(#13595,#13596,#13597,#13598,#13599),
 .UNSPECIFIED.,.F.,.F.,(4,1,4),(14.3981410127769,15.3957123857599,15.7079632679489),
 .UNSPECIFIED.);
#1788=B_SPLINE_CURVE_WITH_KNOTS('',3,(#13602,#13603,#13604,#13605,#13606),
 .UNSPECIFIED.,.F.,.F.,(4,1,4),(13.8761928695312,14.8542941232055,15.7079632679489),
 .UNSPECIFIED.);
#1789=B_SPLINE_CURVE_WITH_KNOTS('',3,(#13612,#13613,#13614,#13615,#13616,
#13617,#13618,#13619,#13620,#13621,#13622,#13623,#13624,#13625,#13626,#13627,
#13628,#13629,#13630,#13631,#13632,#13633),.UNSPECIFIED.,.F.,.F.,(4,3,3,
3,3,3,3,4),(76.7080459413271,76.8129957196859,77.8105670926688,78.8081384656517,
79.8057098386347,80.8032812116176,81.8008525846006,82.7984239575835),
 .UNSPECIFIED.);
#1790=B_SPLINE_CURVE_WITH_KNOTS('',3,(#13637,#13638,#13639,#13640,#13641,
#13642,#13643),.UNSPECIFIED.,.F.,.F.,(4,3,4),(-80.783811092309,-79.8057098386347,
-79.2446069498473),.UNSPECIFIED.);
#1791=B_SPLINE_CURVE_WITH_KNOTS('',3,(#13647,#13648,#13649,#13650,#13651,
#13652,#13653,#13654,#13655,#13656,#13657,#13658,#13659,#13660,#13661,#13662,
#13663,#13664,#13665,#13666,#13667,#13668),.UNSPECIFIED.,.F.,.F.,(4,3,3,
3,3,3,3,4),(-79.2446069498473,-78.8081384656518,-77.8105670926688,-76.8129957196859,
-75.815424346703,-74.81785297372,-73.8202816007371,-72.9614216426678),
 .UNSPECIFIED.);
#1792=B_SPLINE_CURVE_WITH_KNOTS('',3,(#13673,#13674,#13675,#13676,#13677,
#13678,#13679,#13680,#13681,#13682,#13683,#13684,#13685,#13686,#13687,#13688,
#13689,#13690,#13691,#13692,#13693,#13694),.UNSPECIFIED.,.F.,.F.,(4,3,3,
3,3,3,3,4),(70.4248606341475,70.8275674817883,71.8251388547712,72.8227102277542,
73.8202816007371,74.81785297372,75.815424346703,76.7080459413271),
 .UNSPECIFIED.);
#1793=B_SPLINE_CURVE_WITH_KNOTS('',3,(#13695,#13696,#13697,#13698,#13699,
#13700,#13701,#13702,#13703,#13704,#13705,#13706,#13707,#13708,#13709,#13710,
#13711,#13712,#13713,#13714,#13715,#13716,#13717,#13718,#13719),
 .UNSPECIFIED.,.F.,.F.,(4,3,3,3,3,3,3,3,4),(-72.9614216426678,-72.8227102277542,
-71.8251388547712,-70.8275674817883,-69.8299961088054,-68.8324247358224,
-67.8348533628395,-66.8372819898566,-66.6782363354882),.UNSPECIFIED.);
#1794=B_SPLINE_CURVE_WITH_KNOTS('',3,(#13724,#13725,#13726,#13727,#13728,
#13729,#13730,#13731,#13732,#13733,#13734,#13735,#13736,#13737,#13738,#13739,
#13740,#13741,#13742,#13743,#13744,#13745),.UNSPECIFIED.,.F.,.F.,(4,3,3,
3,3,3,3,4),(64.1416753269678,64.8421392438907,65.8397106168736,66.8372819898565,
67.8348533628395,68.8324247358224,69.8299961088054,70.4248606341475),
 .UNSPECIFIED.);
#1795=B_SPLINE_CURVE_WITH_KNOTS('',3,(#13746,#13747,#13748,#13749,#13750,
#13751,#13752,#13753,#13754,#13755,#13756,#13757,#13758,#13759,#13760,#13761,
#13762,#13763,#13764,#13765,#13766,#13767),.UNSPECIFIED.,.F.,.F.,(4,3,3,
3,3,3,3,4),(-66.6782363354882,-65.8397106168736,-64.8421392438907,-63.8445678709078,
-62.8469964979248,-61.8494251249419,-60.851853751959,-60.3950510283085),
 .UNSPECIFIED.);
#1796=B_SPLINE_CURVE_WITH_KNOTS('',3,(#13772,#13773,#13774,#13775,#13776,
#13777,#13778,#13779,#13780,#13781,#13782,#13783,#13784,#13785,#13786,#13787,
#13788,#13789,#13790,#13791,#13792,#13793),.UNSPECIFIED.,.F.,.F.,(4,3,3,
3,3,3,3,4),(57.8584900197882,58.8567110059931,59.854282378976,60.851853751959,
61.8494251249419,62.8469964979248,63.8445678709078,64.1416753269678),
 .UNSPECIFIED.);
#1797=B_SPLINE_CURVE_WITH_KNOTS('',3,(#13794,#13795,#13796,#13797,#13798,
#13799,#13800,#13801,#13802,#13803,#13804,#13805,#13806,#13807,#13808,#13809,
#13810,#13811,#13812,#13813,#13814,#13815),.UNSPECIFIED.,.F.,.F.,(4,3,3,
3,3,3,3,4),(-60.3950510283085,-59.854282378976,-58.8567110059931,-57.8591396330102,
-56.8615682600272,-55.8639968870443,-54.8664255140614,-54.1118657211289),
 .UNSPECIFIED.);
#1798=B_SPLINE_CURVE_WITH_KNOTS('',3,(#13820,#13821,#13822,#13823,#13824,
#13825,#13826,#13827,#13828,#13829,#13830,#13831,#13832,#13833,#13834,#13835,
#13836,#13837,#13838,#13839,#13840,#13841),.UNSPECIFIED.,.F.,.F.,(4,3,3,
3,3,3,3,4),(51.5753047126086,51.8737113951126,52.8712827680955,53.8688541410784,
54.8664255140613,55.8639968870443,56.8615682600272,57.8584900197882),
 .UNSPECIFIED.);
#1799=B_SPLINE_CURVE_WITH_KNOTS('',3,(#13842,#13843,#13844,#13845,#13846,
#13847,#13848,#13849,#13850,#13851,#13852,#13853,#13854,#13855,#13856,#13857,
#13858,#13859,#13860,#13861,#13862,#13863,#13864,#13865,#13866),
 .UNSPECIFIED.,.F.,.F.,(4,3,3,3,3,3,3,3,4),(-54.1118657211289,-53.8688541410784,
-52.8712827680955,-51.8737113951126,-50.8761400221296,-49.8785686491467,
-48.8809972761638,-47.8834259031808,-47.8286804139494),.UNSPECIFIED.);
#1800=B_SPLINE_CURVE_WITH_KNOTS('',3,(#13871,#13872,#13873,#13874,#13875,
#13876,#13877,#13878,#13879,#13880,#13881,#13882,#13883,#13884,#13885,#13886,
#13887,#13888,#13889,#13890,#13891,#13892),.UNSPECIFIED.,.F.,.F.,(4,3,3,
3,3,3,3,4),(45.2921194054291,45.8882831572149,46.8858545301979,47.8834259031808,
48.8809972761637,49.8785686491467,50.8761400221296,51.5753047126086),
 .UNSPECIFIED.);
#1801=B_SPLINE_CURVE_WITH_KNOTS('',3,(#13893,#13894,#13895,#13896,#13897,
#13898,#13899,#13900,#13901,#13902,#13903,#13904,#13905,#13906,#13907,#13908,
#13909,#13910,#13911,#13912,#13913,#13914),.UNSPECIFIED.,.F.,.F.,(4,3,3,
3,3,3,3,4),(-47.8286804139494,-46.8858545301979,-45.888283157215,-44.890711784232,
-43.8931404112491,-42.8955690382662,-41.8979976652832,-41.5454951067698),
 .UNSPECIFIED.);
#1802=B_SPLINE_CURVE_WITH_KNOTS('',3,(#13919,#13920,#13921,#13922,#13923,
#13924,#13925,#13926,#13927,#13928,#13929,#13930,#13931,#13932,#13933,#13934,
#13935,#13936,#13937,#13938,#13939,#13940),.UNSPECIFIED.,.F.,.F.,(4,3,3,
3,3,3,3,4),(39.0089340982495,39.9028549193173,40.9004262923003,41.8979976652832,
42.8955690382661,43.8931404112491,44.890711784232,45.2921194054291),
 .UNSPECIFIED.);
#1803=B_SPLINE_CURVE_WITH_KNOTS('',3,(#13941,#13942,#13943,#13944,#13945,
#13946,#13947,#13948,#13949,#13950,#13951,#13952,#13953,#13954,#13955,#13956,
#13957,#13958,#13959,#13960,#13961,#13962),.UNSPECIFIED.,.F.,.F.,(4,3,3,
3,3,3,3,4),(-41.5454951067698,-40.9004262923003,-39.9028549193174,-38.9052835463344,
-37.9077121733515,-36.9101408003686,-35.9125694273856,-35.2623097995902),
 .UNSPECIFIED.);
#1804=B_SPLINE_CURVE_WITH_KNOTS('',3,(#13967,#13968,#13969,#13970,#13971,
#13972,#13973,#13974,#13975,#13976,#13977,#13978,#13979,#13980,#13981,#13982,
#13983,#13984,#13985,#13986,#13987,#13988,#13989,#13990,#13991),
 .UNSPECIFIED.,.F.,.F.,(4,3,3,3,3,3,3,3,4),(32.7257487910699,32.9198553084368,
33.9174266814197,34.9149980544027,35.9125694273856,36.9101408003685,37.9077121733515,
38.9052835463344,39.0089340982495),.UNSPECIFIED.);
#1805=B_SPLINE_CURVE_WITH_KNOTS('',3,(#13992,#13993,#13994,#13995,#13996,
#13997,#13998,#13999,#14000,#14001,#14002,#14003,#14004,#14005,#14006,#14007,
#14008,#14009,#14010,#14011,#14012,#14013),.UNSPECIFIED.,.F.,.F.,(4,3,3,
3,3,3,3,4),(-35.2623097995902,-34.9149980544027,-33.9174266814198,-32.9198553084368,
-31.9222839354539,-30.924712562471,-29.927141189488,-28.9791244924106),
 .UNSPECIFIED.);
#1806=B_SPLINE_CURVE_WITH_KNOTS('',3,(#14018,#14019,#14020,#14021,#14022,
#14023,#14024,#14025,#14026,#14027,#14028,#14029,#14030,#14031,#14032,#14033,
#14034,#14035,#14036,#14037,#14038,#14039),.UNSPECIFIED.,.F.,.F.,(4,3,3,
3,3,3,3,4),(26.4425634838903,26.9344270705392,27.9319984435221,28.9295698165051,
29.927141189488,30.9247125624709,31.9222839354539,32.7257487910699),
 .UNSPECIFIED.);
#1807=B_SPLINE_CURVE_WITH_KNOTS('',3,(#14040,#14041,#14042,#14043,#14044,
#14045,#14046,#14047,#14048,#14049,#14050,#14051,#14052,#14053,#14054,#14055,
#14056,#14057,#14058,#14059,#14060,#14061,#14062,#14063,#14064),
 .UNSPECIFIED.,.F.,.F.,(4,3,3,3,3,3,3,3,4),(-28.9791244924106,-28.9295698165051,
-27.9319984435222,-26.9344270705392,-25.9368556975563,-24.9392843245733,
-23.9417129515904,-22.9441415786075,-22.695939185231),.UNSPECIFIED.);
#1808=B_SPLINE_CURVE_WITH_KNOTS('',3,(#14069,#14070,#14071,#14072,#14073,
#14074,#14075,#14076,#14077,#14078,#14079,#14080,#14081,#14082,#14083,#14084,
#14085,#14086,#14087,#14088,#14089,#14090),.UNSPECIFIED.,.F.,.F.,(4,3,3,
3,3,3,3,4),(20.1593781767107,20.9489988326416,21.9465702056245,22.9441415786075,
23.9417129515904,24.9392843245733,25.9368556975563,26.4425634838903),
 .UNSPECIFIED.);
#1809=B_SPLINE_CURVE_WITH_KNOTS('',3,(#14091,#14092,#14093,#14094,#14095,
#14096,#14097,#14098,#14099,#14100,#14101,#14102,#14103,#14104,#14105,#14106,
#14107,#14108,#14109,#14110,#14111,#14112),.UNSPECIFIED.,.F.,.F.,(4,3,3,
3,3,3,3,4),(-22.695939185231,-21.9465702056245,-20.9489988326416,-19.9514274596587,
-18.9538560866757,-17.9562847136928,-16.9587133407099,-16.4127538780514),
 .UNSPECIFIED.);
#1810=B_SPLINE_CURVE_WITH_KNOTS('',3,(#14117,#14118,#14119,#14120,#14121,
#14122,#14123,#14124,#14125,#14126,#14127,#14128,#14129,#14130,#14131,#14132,
#14133,#14134,#14135,#14136,#14137,#14138,#14139,#14140,#14141),
 .UNSPECIFIED.,.F.,.F.,(4,3,3,3,3,3,3,3,4),(13.8761928695311,13.9659992217611,
14.963570594744,15.9611419677269,16.9587133407099,17.9562847136928,18.9538560866757,
19.9514274596587,20.1593781767107),.UNSPECIFIED.);
#1811=B_SPLINE_CURVE_WITH_KNOTS('',3,(#14142,#14143,#14144,#14145,#14146,
#14147,#14148,#14149,#14150,#14151,#14152,#14153,#14154,#14155,#14156,#14157,
#14158,#14159,#14160,#14161,#14162,#14163),.UNSPECIFIED.,.F.,.F.,(4,3,3,
3,3,3,3,4),(-16.4127538780514,-15.9611419677269,-14.963570594744,-13.9659992217611,
-12.9684278487781,-11.9708564757952,-10.9732851028123,-10.1295685708718),
 .UNSPECIFIED.);
#1812=B_SPLINE_CURVE_WITH_KNOTS('',3,(#14169,#14170,#14171,#14172,#14173,
#14174,#14175,#14176,#14177,#14178,#14179,#14180,#14181),.UNSPECIFIED.,
 .F.,.F.,(4,3,3,3,4),(-3.84638326369226,-2.9927141189488,-1.99514274596587,
-0.997571372982934,0.),.UNSPECIFIED.);
#1813=B_SPLINE_CURVE_WITH_KNOTS('',3,(#14184,#14185,#14186,#14187,#14188,
#14189,#14190,#14191,#14192,#14193,#14194,#14195,#14196,#14197,#14198,#14199,
#14200,#14201,#14202),.UNSPECIFIED.,.F.,.F.,(4,3,3,3,3,3,4),(2.01461286527457,
2.9927141189488,3.99028549193173,4.98785686491467,5.9854282378976,6.98299961088054,
7.59300756235157),.UNSPECIFIED.);
#1814=B_SPLINE_CURVE_WITH_KNOTS('',3,(#14208,#14209,#14210,#14211,#14212,
#14213,#14214),.UNSPECIFIED.,.F.,.F.,(4,1,1,1,4),(91.106186954104,91.6672898428914,
92.6648612158743,93.6624325888573,94.6600039618402),.UNSPECIFIED.);
#1815=B_SPLINE_CURVE_WITH_KNOTS('',3,(#14217,#14218,#14219,#14220,#14221,
#14222,#14223,#14224),.UNSPECIFIED.,.F.,.F.,(4,1,1,1,1,4),(91.106186954104,
91.2111367324628,92.2087081054457,93.2062794784287,94.2038508514116,95.1819521050859),
 .UNSPECIFIED.);
#1816=B_SPLINE_CURVE_WITH_KNOTS('',3,(#14229,#14230,#14231,#14232,#14233,
#14234,#14235,#14236,#14237,#14238),.UNSPECIFIED.,.F.,.F.,(4,1,1,1,1,1,
1,4),(84.8230016469244,85.6818616049938,86.6794329779767,87.6770043509596,
88.6745757239426,89.6721470969255,90.6697184699085,91.106186954104),
 .UNSPECIFIED.);
#1817=B_SPLINE_CURVE_WITH_KNOTS('',3,(#14239,#14240,#14241,#14242,#14243,
#14244,#14245,#14246,#14247,#14248),.UNSPECIFIED.,.F.,.F.,(4,1,1,1,1,1,
1,4),(84.8230016469244,85.2257084945652,86.2232798675481,87.2208512405311,
88.218422613514,89.2159939864969,90.2135653594799,91.106186954104),
 .UNSPECIFIED.);
#1818=B_SPLINE_CURVE_WITH_KNOTS('',3,(#14253,#14254,#14255,#14256,#14257,
#14258,#14259,#14260,#14261,#14262,#14263),.UNSPECIFIED.,.F.,.F.,(4,1,1,
1,1,1,1,1,4),(78.5398163397448,78.6988619941132,79.6964333670962,80.6940047400791,
81.6915761130621,82.689147486045,83.6867188590279,84.6842902320109,84.8230016469244),
 .UNSPECIFIED.);
#1819=B_SPLINE_CURVE_WITH_KNOTS('',3,(#14264,#14265,#14266,#14267,#14268,
#14269,#14270,#14271,#14272,#14273),.UNSPECIFIED.,.F.,.F.,(4,1,1,1,1,1,
1,4),(78.5398163397448,79.2402802566676,80.2378516296505,81.2354230026335,
82.2329943756164,83.2305657485993,84.2281371215823,84.8230016469244),
 .UNSPECIFIED.);
#1820=B_SPLINE_CURVE_WITH_KNOTS('',3,(#14278,#14279,#14280,#14281,#14282,
#14283,#14284,#14285,#14286,#14287),.UNSPECIFIED.,.F.,.F.,(4,1,1,1,1,1,
1,4),(72.2566310325652,72.7134337562156,73.7110051291986,74.7085765021815,
75.7061478751644,76.7037192481474,77.7012906211303,78.5398163397448),
 .UNSPECIFIED.);
#1821=B_SPLINE_CURVE_WITH_KNOTS('',3,(#14288,#14289,#14290,#14291,#14292,
#14293,#14294,#14295,#14296,#14297,#14298),.UNSPECIFIED.,.F.,.F.,(4,1,1,
1,1,1,1,1,4),(72.2566310325652,72.2572806457871,73.25485201877,74.2524233917529,
75.2499947647359,76.2475661377188,77.2451375107017,78.2427088836847,78.5398163397448),
 .UNSPECIFIED.);
#1822=B_SPLINE_CURVE_WITH_KNOTS('',3,(#14303,#14304,#14305,#14306,#14307,
#14308,#14309,#14310,#14311,#14312),.UNSPECIFIED.,.F.,.F.,(4,1,1,1,1,1,
1,4),(65.9734457253856,66.728005518318,67.725576891301,68.7231482642839,
69.7207196372668,70.7182910102498,71.7158623832327,72.2566310325652),
 .UNSPECIFIED.);
#1823=B_SPLINE_CURVE_WITH_KNOTS('',3,(#14313,#14314,#14315,#14316,#14317,
#14318,#14319,#14320,#14321,#14322),.UNSPECIFIED.,.F.,.F.,(4,1,1,1,1,1,
1,4),(65.9734457253856,66.2718524078895,67.2694237808724,68.2669951538553,
69.2645665268383,70.2621378998212,71.2597092728041,72.2566310325652),
 .UNSPECIFIED.);
#1824=B_SPLINE_CURVE_WITH_KNOTS('',3,(#14327,#14328,#14329,#14330,#14331,
#14332,#14333,#14334,#14335,#14336,#14337),.UNSPECIFIED.,.F.,.F.,(4,1,1,
1,1,1,1,1,4),(59.690260418206,59.7450059074375,60.7425772804204,61.7401486534034,
62.7377200263863,63.7352913993692,64.7328627723522,65.7304341453351,65.9734457253856),
 .UNSPECIFIED.);
#1825=B_SPLINE_CURVE_WITH_KNOTS('',3,(#14338,#14339,#14340,#14341,#14342,
#14343,#14344,#14345,#14346,#14347),.UNSPECIFIED.,.F.,.F.,(4,1,1,1,1,1,
1,4),(59.690260418206,60.2864241699919,61.2839955429748,62.2815669159577,
63.2791382889407,64.2767096619236,65.2742810349065,65.9734457253856),
 .UNSPECIFIED.);
#1826=B_SPLINE_CURVE_WITH_KNOTS('',3,(#14352,#14353,#14354,#14355,#14356,
#14357,#14358,#14359,#14360,#14361),.UNSPECIFIED.,.F.,.F.,(4,1,1,1,1,1,
1,4),(53.4070751110264,53.7595776695399,54.7571490425228,55.7547204155058,
56.7522917884887,57.7498631614716,58.7474345344546,59.690260418206),
 .UNSPECIFIED.);
#1827=B_SPLINE_CURVE_WITH_KNOTS('',3,(#14362,#14363,#14364,#14365,#14366,
#14367,#14368,#14369,#14370,#14371),.UNSPECIFIED.,.F.,.F.,(4,1,1,1,1,1,
1,4),(53.4070751110264,54.3009959320943,55.2985673050772,56.2961386780601,
57.2937100510431,58.291281424026,59.2888527970089,59.690260418206),
 .UNSPECIFIED.);
#1828=B_SPLINE_CURVE_WITH_KNOTS('',3,(#14376,#14377,#14378,#14379,#14380,
#14381,#14382,#14383,#14384,#14385),.UNSPECIFIED.,.F.,.F.,(4,1,1,1,1,1,
1,4),(47.1238898038469,47.7741494316423,48.7717208046252,49.7692921776082,
50.7668635505911,51.764434923574,52.762006296557,53.4070751110264),
 .UNSPECIFIED.);
#1829=B_SPLINE_CURVE_WITH_KNOTS('',3,(#14386,#14387,#14388,#14389,#14390,
#14391,#14392,#14393,#14394,#14395,#14396),.UNSPECIFIED.,.F.,.F.,(4,1,1,
1,1,1,1,1,4),(47.1238898038469,47.3179963212137,48.3155676941967,49.3131390671796,
50.3107104401625,51.3082818131455,52.3058531861284,53.3034245591113,53.4070751110264),
 .UNSPECIFIED.);
#1830=B_SPLINE_CURVE_WITH_KNOTS('',3,(#14401,#14402,#14403,#14404,#14405,
#14406,#14407,#14408,#14409,#14410),.UNSPECIFIED.,.F.,.F.,(4,1,1,1,1,1,
1,4),(40.8407044966673,41.7887211937447,42.7862925667276,43.7838639397106,
44.7814353126935,45.7790066856764,46.7765780586594,47.1238898038469),
 .UNSPECIFIED.);
#1831=B_SPLINE_CURVE_WITH_KNOTS('',3,(#14411,#14412,#14413,#14414,#14415,
#14416,#14417,#14418,#14419,#14420),.UNSPECIFIED.,.F.,.F.,(4,1,1,1,1,1,
1,4),(40.8407044966673,41.3325680833161,42.3301394562991,43.327710829282,
44.3252822022649,45.3228535752479,46.3204249482308,47.1238898038469),
 .UNSPECIFIED.);
#1832=B_SPLINE_CURVE_WITH_KNOTS('',3,(#14425,#14426,#14427,#14428,#14429,
#14430,#14431,#14432,#14433,#14434,#14435),.UNSPECIFIED.,.F.,.F.,(4,1,1,
1,1,1,1,1,4),(34.5575191894876,34.8057215828642,35.8032929558471,36.80086432883,
37.798435701813,38.7960070747959,39.7935784477788,40.7911498207618,40.8407044966673),
 .UNSPECIFIED.);
#1833=B_SPLINE_CURVE_WITH_KNOTS('',3,(#14436,#14437,#14438,#14439,#14440,
#14441,#14442,#14443,#14444,#14445),.UNSPECIFIED.,.F.,.F.,(4,1,1,1,1,1,
1,4),(34.5575191894876,35.3471398454185,36.3447112184015,37.3422825913844,
38.3398539643673,39.3374253373503,40.3349967103332,40.8407044966673),
 .UNSPECIFIED.);
#1834=B_SPLINE_CURVE_WITH_KNOTS('',3,(#14450,#14451,#14452,#14453,#14454,
#14455,#14456,#14457,#14458,#14459),.UNSPECIFIED.,.F.,.F.,(4,1,1,1,1,1,
1,4),(28.2743338823081,28.8202933449666,29.8178647179495,30.8154360909324,
31.8130074639154,32.8105788368983,33.8081502098812,34.5575191894876),
 .UNSPECIFIED.);
#1835=B_SPLINE_CURVE_WITH_KNOTS('',3,(#14460,#14461,#14462,#14463,#14464,
#14465,#14466,#14467,#14468,#14469,#14470),.UNSPECIFIED.,.F.,.F.,(4,1,1,
1,1,1,1,1,4),(28.2743338823081,28.364140234538,29.3617116075209,30.3592829805039,
31.3568543534868,32.3544257264697,33.3519970994527,34.3495684724356,34.5575191894876),
 .UNSPECIFIED.);
#1836=B_SPLINE_CURVE_WITH_KNOTS('',3,(#14475,#14476,#14477,#14478,#14479,
#14480,#14481,#14482,#14483,#14484),.UNSPECIFIED.,.F.,.F.,(4,1,1,1,1,1,
1,4),(21.9911485751285,22.8348651070689,23.8324364800519,24.8300078530348,
25.8275792260178,26.8251505990007,27.8227219719836,28.2743338823081),
 .UNSPECIFIED.);
#1837=B_SPLINE_CURVE_WITH_KNOTS('',3,(#14485,#14486,#14487,#14488,#14489,
#14490,#14491,#14492,#14493,#14494),.UNSPECIFIED.,.F.,.F.,(4,1,1,1,1,1,
1,4),(21.9911485751285,22.3787119966404,23.3762833696233,24.3738547426063,
25.3714261155892,26.3689974885721,27.3665688615551,28.2743338823081),
 .UNSPECIFIED.);
#1838=B_SPLINE_CURVE_WITH_KNOTS('',3,(#14500,#14501,#14502,#14503,#14504),
 .UNSPECIFIED.,.F.,.F.,(4,1,4),(14.3981410127769,15.3957123857599,15.7079632679489),
 .UNSPECIFIED.);
#1839=B_SPLINE_CURVE_WITH_KNOTS('',3,(#14507,#14508,#14509,#14510,#14511),
 .UNSPECIFIED.,.F.,.F.,(4,1,4),(13.8761928695312,14.8542941232055,15.7079632679489),
 .UNSPECIFIED.);
#1840=B_SPLINE_CURVE_WITH_KNOTS('',3,(#14517,#14518,#14519,#14520,#14521,
#14522,#14523,#14524,#14525,#14526,#14527,#14528,#14529,#14530,#14531,#14532,
#14533,#14534,#14535,#14536,#14537,#14538),.UNSPECIFIED.,.F.,.F.,(4,3,3,
3,3,3,3,4),(76.7080459413271,76.812995719686,77.8105670926689,78.8081384656519,
79.8057098386348,80.8032812116178,81.8008525846007,82.7984239575837),
 .UNSPECIFIED.);
#1841=B_SPLINE_CURVE_WITH_KNOTS('',3,(#14542,#14543,#14544,#14545,#14546,
#14547,#14548),.UNSPECIFIED.,.F.,.F.,(4,3,4),(-80.7838110923091,-79.8057098386348,
-79.2446069498473),.UNSPECIFIED.);
#1842=B_SPLINE_CURVE_WITH_KNOTS('',3,(#14552,#14553,#14554,#14555,#14556,
#14557,#14558,#14559,#14560,#14561,#14562,#14563,#14564,#14565,#14566,#14567,
#14568,#14569,#14570,#14571,#14572,#14573),.UNSPECIFIED.,.F.,.F.,(4,3,3,
3,3,3,3,4),(-79.2446069498473,-78.8081384656519,-77.8105670926689,-76.812995719686,
-75.815424346703,-74.8178529737201,-73.8202816007372,-72.9614216426678),
 .UNSPECIFIED.);
#1843=B_SPLINE_CURVE_WITH_KNOTS('',3,(#14578,#14579,#14580,#14581,#14582,
#14583,#14584,#14585,#14586,#14587,#14588,#14589,#14590,#14591,#14592,#14593,
#14594,#14595,#14596,#14597,#14598,#14599),.UNSPECIFIED.,.F.,.F.,(4,3,3,
3,3,3,3,4),(70.4248606341475,70.8275674817883,71.8251388547713,72.8227102277543,
73.8202816007372,74.8178529737201,75.815424346703,76.7080459413271),
 .UNSPECIFIED.);
#1844=B_SPLINE_CURVE_WITH_KNOTS('',3,(#14600,#14601,#14602,#14603,#14604,
#14605,#14606,#14607,#14608,#14609,#14610,#14611,#14612,#14613,#14614,#14615,
#14616,#14617,#14618,#14619,#14620,#14621,#14622,#14623,#14624),
 .UNSPECIFIED.,.F.,.F.,(4,3,3,3,3,3,3,3,4),(-72.9614216426678,-72.8227102277542,
-71.8251388547713,-70.8275674817884,-69.8299961088054,-68.8324247358225,
-67.8348533628396,-66.8372819898566,-66.6782363354882),.UNSPECIFIED.);
#1845=B_SPLINE_CURVE_WITH_KNOTS('',3,(#14629,#14630,#14631,#14632,#14633,
#14634,#14635,#14636,#14637,#14638,#14639,#14640,#14641,#14642,#14643,#14644,
#14645,#14646,#14647,#14648,#14649,#14650),.UNSPECIFIED.,.F.,.F.,(4,3,3,
3,3,3,3,4),(64.1416753269678,64.8421392438907,65.8397106168737,66.8372819898566,
67.8348533628396,68.8324247358225,69.8299961088054,70.4248606341475),
 .UNSPECIFIED.);
#1846=B_SPLINE_CURVE_WITH_KNOTS('',3,(#14651,#14652,#14653,#14654,#14655,
#14656,#14657,#14658,#14659,#14660,#14661,#14662,#14663,#14664,#14665,#14666,
#14667,#14668,#14669,#14670,#14671,#14672),.UNSPECIFIED.,.F.,.F.,(4,3,3,
3,3,3,3,4),(-66.6782363354882,-65.8397106168737,-64.8421392438908,-63.8445678709078,
-62.8469964979249,-61.849425124942,-60.851853751959,-60.3950510283085),
 .UNSPECIFIED.);
#1847=B_SPLINE_CURVE_WITH_KNOTS('',3,(#14677,#14678,#14679,#14680,#14681,
#14682,#14683,#14684,#14685,#14686,#14687,#14688,#14689,#14690,#14691,#14692,
#14693,#14694,#14695,#14696,#14697,#14698),.UNSPECIFIED.,.F.,.F.,(4,3,3,
3,3,3,3,4),(57.8584900197882,58.8567110059931,59.8542823789761,60.851853751959,
61.849425124942,62.8469964979249,63.8445678709078,64.1416753269678),
 .UNSPECIFIED.);
#1848=B_SPLINE_CURVE_WITH_KNOTS('',3,(#14699,#14700,#14701,#14702,#14703,
#14704,#14705,#14706,#14707,#14708,#14709,#14710,#14711,#14712,#14713,#14714,
#14715,#14716,#14717,#14718,#14719,#14720),.UNSPECIFIED.,.F.,.F.,(4,3,3,
3,3,3,3,4),(-60.3950510283085,-59.8542823789761,-58.8567110059932,-57.8591396330102,
-56.8615682600273,-55.8639968870443,-54.8664255140614,-54.1118657211289),
 .UNSPECIFIED.);
#1849=B_SPLINE_CURVE_WITH_KNOTS('',3,(#14725,#14726,#14727,#14728,#14729,
#14730,#14731,#14732,#14733,#14734,#14735,#14736,#14737,#14738,#14739,#14740,
#14741,#14742,#14743,#14744,#14745,#14746),.UNSPECIFIED.,.F.,.F.,(4,3,3,
3,3,3,3,4),(51.5753047126086,51.8737113951126,52.8712827680955,53.8688541410785,
54.8664255140614,55.8639968870444,56.8615682600273,57.8584900197882),
 .UNSPECIFIED.);
#1850=B_SPLINE_CURVE_WITH_KNOTS('',3,(#14747,#14748,#14749,#14750,#14751,
#14752,#14753,#14754,#14755,#14756,#14757,#14758,#14759,#14760,#14761,#14762,
#14763,#14764,#14765,#14766,#14767,#14768,#14769,#14770,#14771),
 .UNSPECIFIED.,.F.,.F.,(4,3,3,3,3,3,3,3,4),(-54.1118657211289,-53.8688541410785,
-52.8712827680955,-51.8737113951126,-50.8761400221297,-49.8785686491467,
-48.8809972761638,-47.8834259031809,-47.8286804139493),.UNSPECIFIED.);
#1851=B_SPLINE_CURVE_WITH_KNOTS('',3,(#14776,#14777,#14778,#14779,#14780,
#14781,#14782,#14783,#14784,#14785,#14786,#14787,#14788,#14789,#14790,#14791,
#14792,#14793,#14794,#14795,#14796,#14797),.UNSPECIFIED.,.F.,.F.,(4,3,3,
3,3,3,3,4),(45.2921194054291,45.888283157215,46.8858545301979,47.8834259031809,
48.8809972761638,49.8785686491467,50.8761400221297,51.5753047126086),
 .UNSPECIFIED.);
#1852=B_SPLINE_CURVE_WITH_KNOTS('',3,(#14798,#14799,#14800,#14801,#14802,
#14803,#14804,#14805,#14806,#14807,#14808,#14809,#14810,#14811,#14812,#14813,
#14814,#14815,#14816,#14817,#14818,#14819),.UNSPECIFIED.,.F.,.F.,(4,3,3,
3,3,3,3,4),(-47.8286804139493,-46.8858545301979,-45.888283157215,-44.8907117842321,
-43.8931404112491,-42.8955690382662,-41.8979976652833,-41.5454951067698),
 .UNSPECIFIED.);
#1853=B_SPLINE_CURVE_WITH_KNOTS('',3,(#14824,#14825,#14826,#14827,#14828,
#14829,#14830,#14831,#14832,#14833,#14834,#14835,#14836,#14837,#14838,#14839,
#14840,#14841,#14842,#14843,#14844,#14845),.UNSPECIFIED.,.F.,.F.,(4,3,3,
3,3,3,3,4),(39.0089340982495,39.9028549193174,40.9004262923003,41.8979976652833,
42.8955690382662,43.8931404112491,44.8907117842321,45.2921194054291),
 .UNSPECIFIED.);
#1854=B_SPLINE_CURVE_WITH_KNOTS('',3,(#14846,#14847,#14848,#14849,#14850,
#14851,#14852,#14853,#14854,#14855,#14856,#14857,#14858,#14859,#14860,#14861,
#14862,#14863,#14864,#14865,#14866,#14867),.UNSPECIFIED.,.F.,.F.,(4,3,3,
3,3,3,3,4),(-41.5454951067698,-40.9004262923003,-39.9028549193174,-38.9052835463345,
-37.9077121733515,-36.9101408003686,-35.9125694273856,-35.2623097995902),
 .UNSPECIFIED.);
#1855=B_SPLINE_CURVE_WITH_KNOTS('',3,(#14872,#14873,#14874,#14875,#14876,
#14877,#14878,#14879,#14880,#14881,#14882,#14883,#14884,#14885,#14886,#14887,
#14888,#14889,#14890,#14891,#14892,#14893,#14894,#14895,#14896),
 .UNSPECIFIED.,.F.,.F.,(4,3,3,3,3,3,3,3,4),(32.7257487910699,32.9198553084368,
33.9174266814198,34.9149980544027,35.9125694273856,36.9101408003686,37.9077121733515,
38.9052835463345,39.0089340982495),.UNSPECIFIED.);
#1856=B_SPLINE_CURVE_WITH_KNOTS('',3,(#14897,#14898,#14899,#14900,#14901,
#14902,#14903,#14904,#14905,#14906,#14907,#14908,#14909,#14910,#14911,#14912,
#14913,#14914,#14915,#14916,#14917,#14918),.UNSPECIFIED.,.F.,.F.,(4,3,3,
3,3,3,3,4),(-35.2623097995902,-34.9149980544027,-33.9174266814198,-32.9198553084368,
-31.9222839354539,-30.924712562471,-29.927141189488,-28.9791244924106),
 .UNSPECIFIED.);
#1857=B_SPLINE_CURVE_WITH_KNOTS('',3,(#14923,#14924,#14925,#14926,#14927,
#14928,#14929,#14930,#14931,#14932,#14933,#14934,#14935,#14936,#14937,#14938,
#14939,#14940,#14941,#14942,#14943,#14944),.UNSPECIFIED.,.F.,.F.,(4,3,3,
3,3,3,3,4),(26.4425634838903,26.9344270705392,27.9319984435222,28.9295698165051,
29.927141189488,30.924712562471,31.9222839354539,32.7257487910699),
 .UNSPECIFIED.);
#1858=B_SPLINE_CURVE_WITH_KNOTS('',3,(#14945,#14946,#14947,#14948,#14949,
#14950,#14951,#14952,#14953,#14954,#14955,#14956,#14957,#14958,#14959,#14960,
#14961,#14962,#14963,#14964,#14965,#14966,#14967,#14968,#14969),
 .UNSPECIFIED.,.F.,.F.,(4,3,3,3,3,3,3,3,4),(-28.9791244924106,-28.9295698165051,
-27.9319984435222,-26.9344270705392,-25.9368556975563,-24.9392843245734,
-23.9417129515904,-22.9441415786075,-22.695939185231),.UNSPECIFIED.);
#1859=B_SPLINE_CURVE_WITH_KNOTS('',3,(#14974,#14975,#14976,#14977,#14978,
#14979,#14980,#14981,#14982,#14983,#14984,#14985,#14986,#14987,#14988,#14989,
#14990,#14991,#14992,#14993,#14994,#14995),.UNSPECIFIED.,.F.,.F.,(4,3,3,
3,3,3,3,4),(20.1593781767107,20.9489988326416,21.9465702056246,22.9441415786075,
23.9417129515904,24.9392843245734,25.9368556975563,26.4425634838903),
 .UNSPECIFIED.);
#1860=B_SPLINE_CURVE_WITH_KNOTS('',3,(#14996,#14997,#14998,#14999,#15000,
#15001,#15002,#15003,#15004,#15005,#15006,#15007,#15008,#15009,#15010,#15011,
#15012,#15013,#15014,#15015,#15016,#15017),.UNSPECIFIED.,.F.,.F.,(4,3,3,
3,3,3,3,4),(-22.695939185231,-21.9465702056246,-20.9489988326416,-19.9514274596587,
-18.9538560866758,-17.9562847136928,-16.9587133407099,-16.4127538780514),
 .UNSPECIFIED.);
#1861=B_SPLINE_CURVE_WITH_KNOTS('',3,(#15022,#15023,#15024,#15025,#15026,
#15027,#15028,#15029,#15030,#15031,#15032,#15033,#15034,#15035,#15036,#15037,
#15038,#15039,#15040,#15041,#15042,#15043,#15044,#15045,#15046),
 .UNSPECIFIED.,.F.,.F.,(4,3,3,3,3,3,3,3,4),(13.8761928695311,13.9659992217611,
14.963570594744,15.961141967727,16.9587133407099,17.9562847136928,18.9538560866758,
19.9514274596587,20.1593781767107),.UNSPECIFIED.);
#1862=B_SPLINE_CURVE_WITH_KNOTS('',3,(#15047,#15048,#15049,#15050,#15051,
#15052,#15053,#15054,#15055,#15056,#15057,#15058,#15059,#15060,#15061,#15062,
#15063,#15064,#15065,#15066,#15067,#15068),.UNSPECIFIED.,.F.,.F.,(4,3,3,
3,3,3,3,4),(-16.4127538780514,-15.9611419677269,-14.963570594744,-13.9659992217611,
-12.9684278487781,-11.9708564757952,-10.9732851028123,-10.1295685708718),
 .UNSPECIFIED.);
#1863=B_SPLINE_CURVE_WITH_KNOTS('',3,(#15074,#15075,#15076,#15077,#15078,
#15079,#15080,#15081,#15082,#15083,#15084,#15085,#15086),.UNSPECIFIED.,
 .F.,.F.,(4,3,3,3,4),(-3.84638326369226,-2.9927141189488,-1.99514274596587,
-0.997571372982931,0.),.UNSPECIFIED.);
#1864=B_SPLINE_CURVE_WITH_KNOTS('',3,(#15089,#15090,#15091,#15092,#15093,
#15094,#15095,#15096,#15097,#15098,#15099,#15100,#15101,#15102,#15103,#15104,
#15105,#15106,#15107),.UNSPECIFIED.,.F.,.F.,(4,3,3,3,3,3,4),(2.01461286527457,
2.9927141189488,3.99028549193174,4.98785686491468,5.98542823789761,6.98299961088054,
7.59300756235157),.UNSPECIFIED.);
#1865=B_SPLINE_CURVE_WITH_KNOTS('',3,(#15113,#15114,#15115,#15116,#15117,
#15118,#15119),.UNSPECIFIED.,.F.,.F.,(4,1,1,1,4),(91.106186954104,91.6672898428915,
92.6648612158744,93.6624325888573,94.6600039618403),.UNSPECIFIED.);
#1866=B_SPLINE_CURVE_WITH_KNOTS('',3,(#15122,#15123,#15124,#15125,#15126,
#15127,#15128,#15129),.UNSPECIFIED.,.F.,.F.,(4,1,1,1,1,4),(91.106186954104,
91.2111367324629,92.2087081054458,93.2062794784288,94.2038508514117,95.181952105086),
 .UNSPECIFIED.);
#1867=B_SPLINE_CURVE_WITH_KNOTS('',3,(#15134,#15135,#15136,#15137,#15138,
#15139,#15140,#15141,#15142,#15143),.UNSPECIFIED.,.F.,.F.,(4,1,1,1,1,1,
1,4),(84.8230016469244,85.6818616049939,86.6794329779768,87.6770043509597,
88.6745757239427,89.6721470969256,90.6697184699085,91.106186954104),
 .UNSPECIFIED.);
#1868=B_SPLINE_CURVE_WITH_KNOTS('',3,(#15144,#15145,#15146,#15147,#15148,
#15149,#15150,#15151,#15152,#15153),.UNSPECIFIED.,.F.,.F.,(4,1,1,1,1,1,
1,4),(84.8230016469244,85.2257084945653,86.2232798675482,87.2208512405312,
88.2184226135141,89.215993986497,90.21356535948,91.106186954104),
 .UNSPECIFIED.);
#1869=B_SPLINE_CURVE_WITH_KNOTS('',3,(#15158,#15159,#15160,#15161,#15162,
#15163,#15164,#15165,#15166,#15167,#15168),.UNSPECIFIED.,.F.,.F.,(4,1,1,
1,1,1,1,1,4),(78.5398163397448,78.6988619941133,79.6964333670962,80.6940047400792,
81.6915761130621,82.689147486045,83.686718859028,84.6842902320109,84.8230016469244),
 .UNSPECIFIED.);
#1870=B_SPLINE_CURVE_WITH_KNOTS('',3,(#15169,#15170,#15171,#15172,#15173,
#15174,#15175,#15176,#15177,#15178),.UNSPECIFIED.,.F.,.F.,(4,1,1,1,1,1,
1,4),(78.5398163397448,79.2402802566677,80.2378516296506,81.2354230026336,
82.2329943756165,83.2305657485994,84.2281371215823,84.8230016469244),
 .UNSPECIFIED.);
#1871=B_SPLINE_CURVE_WITH_KNOTS('',3,(#15183,#15184,#15185,#15186,#15187,
#15188,#15189,#15190,#15191,#15192),.UNSPECIFIED.,.F.,.F.,(4,1,1,1,1,1,
1,4),(72.2566310325652,72.7134337562157,73.7110051291986,74.7085765021816,
75.7061478751645,76.7037192481474,77.7012906211304,78.5398163397448),
 .UNSPECIFIED.);
#1872=B_SPLINE_CURVE_WITH_KNOTS('',3,(#15193,#15194,#15195,#15196,#15197,
#15198,#15199,#15200,#15201,#15202,#15203),.UNSPECIFIED.,.F.,.F.,(4,1,1,
1,1,1,1,1,4),(72.2566310325652,72.2572806457871,73.2548520187701,74.252423391753,
75.2499947647359,76.2475661377189,77.2451375107018,78.2427088836847,78.5398163397448),
 .UNSPECIFIED.);
#1873=B_SPLINE_CURVE_WITH_KNOTS('',3,(#15208,#15209,#15210,#15211,#15212,
#15213,#15214,#15215,#15216,#15217),.UNSPECIFIED.,.F.,.F.,(4,1,1,1,1,1,
1,4),(65.9734457253856,66.7280055183181,67.725576891301,68.723148264284,
69.7207196372669,70.7182910102498,71.7158623832328,72.2566310325652),
 .UNSPECIFIED.);
#1874=B_SPLINE_CURVE_WITH_KNOTS('',3,(#15218,#15219,#15220,#15221,#15222,
#15223,#15224,#15225,#15226,#15227),.UNSPECIFIED.,.F.,.F.,(4,1,1,1,1,1,
1,4),(65.9734457253856,66.2718524078895,67.2694237808725,68.2669951538554,
69.2645665268383,70.2621378998213,71.2597092728042,72.2566310325652),
 .UNSPECIFIED.);
#1875=B_SPLINE_CURVE_WITH_KNOTS('',3,(#15232,#15233,#15234,#15235,#15236,
#15237,#15238,#15239,#15240,#15241,#15242),.UNSPECIFIED.,.F.,.F.,(4,1,1,
1,1,1,1,1,4),(59.690260418206,59.7450059074375,60.7425772804205,61.7401486534034,
62.7377200263864,63.7352913993693,64.7328627723522,65.7304341453352,65.9734457253856),
 .UNSPECIFIED.);
#1876=B_SPLINE_CURVE_WITH_KNOTS('',3,(#15243,#15244,#15245,#15246,#15247,
#15248,#15249,#15250,#15251,#15252),.UNSPECIFIED.,.F.,.F.,(4,1,1,1,1,1,
1,4),(59.690260418206,60.2864241699919,61.2839955429748,62.2815669159578,
63.2791382889407,64.2767096619237,65.2742810349066,65.9734457253856),
 .UNSPECIFIED.);
#1877=B_SPLINE_CURVE_WITH_KNOTS('',3,(#15257,#15258,#15259,#15260,#15261,
#15262,#15263,#15264,#15265,#15266),.UNSPECIFIED.,.F.,.F.,(4,1,1,1,1,1,
1,4),(53.4070751110264,53.7595776695399,54.7571490425229,55.7547204155058,
56.7522917884887,57.7498631614717,58.7474345344546,59.690260418206),
 .UNSPECIFIED.);
#1878=B_SPLINE_CURVE_WITH_KNOTS('',3,(#15267,#15268,#15269,#15270,#15271,
#15272,#15273,#15274,#15275,#15276),.UNSPECIFIED.,.F.,.F.,(4,1,1,1,1,1,
1,4),(53.4070751110264,54.3009959320943,55.2985673050772,56.2961386780602,
57.2937100510431,58.291281424026,59.288852797009,59.690260418206),
 .UNSPECIFIED.);
#1879=B_SPLINE_CURVE_WITH_KNOTS('',3,(#15281,#15282,#15283,#15284,#15285,
#15286,#15287,#15288,#15289,#15290),.UNSPECIFIED.,.F.,.F.,(4,1,1,1,1,1,
1,4),(47.1238898038469,47.7741494316423,48.7717208046253,49.7692921776082,
50.7668635505911,51.7644349235741,52.762006296557,53.4070751110264),
 .UNSPECIFIED.);
#1880=B_SPLINE_CURVE_WITH_KNOTS('',3,(#15291,#15292,#15293,#15294,#15295,
#15296,#15297,#15298,#15299,#15300,#15301),.UNSPECIFIED.,.F.,.F.,(4,1,1,
1,1,1,1,1,4),(47.1238898038469,47.3179963212138,48.3155676941967,49.3131390671796,
50.3107104401626,51.3082818131455,52.3058531861284,53.3034245591114,53.4070751110264),
 .UNSPECIFIED.);
#1881=B_SPLINE_CURVE_WITH_KNOTS('',3,(#15306,#15307,#15308,#15309,#15310,
#15311,#15312,#15313,#15314,#15315),.UNSPECIFIED.,.F.,.F.,(4,1,1,1,1,1,
1,4),(40.8407044966673,41.7887211937447,42.7862925667277,43.7838639397106,
44.7814353126935,45.7790066856765,46.7765780586594,47.1238898038469),
 .UNSPECIFIED.);
#1882=B_SPLINE_CURVE_WITH_KNOTS('',3,(#15316,#15317,#15318,#15319,#15320,
#15321,#15322,#15323,#15324,#15325),.UNSPECIFIED.,.F.,.F.,(4,1,1,1,1,1,
1,4),(40.8407044966673,41.3325680833162,42.3301394562991,43.327710829282,
44.325282202265,45.3228535752479,46.3204249482308,47.1238898038469),
 .UNSPECIFIED.);
#1883=B_SPLINE_CURVE_WITH_KNOTS('',3,(#15330,#15331,#15332,#15333,#15334,
#15335,#15336,#15337,#15338,#15339,#15340),.UNSPECIFIED.,.F.,.F.,(4,1,1,
1,1,1,1,1,4),(34.5575191894876,34.8057215828642,35.8032929558471,36.80086432883,
37.798435701813,38.7960070747959,39.7935784477789,40.7911498207618,40.8407044966673),
 .UNSPECIFIED.);
#1884=B_SPLINE_CURVE_WITH_KNOTS('',3,(#15341,#15342,#15343,#15344,#15345,
#15346,#15347,#15348,#15349,#15350),.UNSPECIFIED.,.F.,.F.,(4,1,1,1,1,1,
1,4),(34.5575191894876,35.3471398454185,36.3447112184015,37.3422825913844,
38.3398539643674,39.3374253373503,40.3349967103332,40.8407044966673),
 .UNSPECIFIED.);
#1885=B_SPLINE_CURVE_WITH_KNOTS('',3,(#15355,#15356,#15357,#15358,#15359,
#15360,#15361,#15362,#15363,#15364),.UNSPECIFIED.,.F.,.F.,(4,1,1,1,1,1,
1,4),(28.2743338823081,28.8202933449666,29.8178647179495,30.8154360909324,
31.8130074639154,32.8105788368983,33.8081502098812,34.5575191894876),
 .UNSPECIFIED.);
#1886=B_SPLINE_CURVE_WITH_KNOTS('',3,(#15365,#15366,#15367,#15368,#15369,
#15370,#15371,#15372,#15373,#15374,#15375),.UNSPECIFIED.,.F.,.F.,(4,1,1,
1,1,1,1,1,4),(28.2743338823081,28.364140234538,29.3617116075209,30.3592829805039,
31.3568543534868,32.3544257264697,33.3519970994527,34.3495684724356,34.5575191894876),
 .UNSPECIFIED.);
#1887=B_SPLINE_CURVE_WITH_KNOTS('',3,(#15380,#15381,#15382,#15383,#15384,
#15385,#15386,#15387,#15388,#15389),.UNSPECIFIED.,.F.,.F.,(4,1,1,1,1,1,
1,4),(21.9911485751285,22.834865107069,23.8324364800519,24.8300078530348,
25.8275792260178,26.8251505990007,27.8227219719836,28.2743338823081),
 .UNSPECIFIED.);
#1888=B_SPLINE_CURVE_WITH_KNOTS('',3,(#15390,#15391,#15392,#15393,#15394,
#15395,#15396,#15397,#15398,#15399),.UNSPECIFIED.,.F.,.F.,(4,1,1,1,1,1,
1,4),(21.9911485751285,22.3787119966404,23.3762833696233,24.3738547426063,
25.3714261155892,26.3689974885721,27.3665688615551,28.2743338823081),
 .UNSPECIFIED.);
#1889=B_SPLINE_CURVE_WITH_KNOTS('',3,(#15405,#15406,#15407,#15408,#15409),
 .UNSPECIFIED.,.F.,.F.,(4,1,4),(14.3981410127769,15.3957123857599,15.7079632679489),
 .UNSPECIFIED.);
#1890=B_SPLINE_CURVE_WITH_KNOTS('',3,(#15412,#15413,#15414,#15415,#15416),
 .UNSPECIFIED.,.F.,.F.,(4,1,4),(13.8761928695312,14.8542941232055,15.7079632679489),
 .UNSPECIFIED.);
#1891=B_SPLINE_CURVE_WITH_KNOTS('',3,(#15422,#15423,#15424,#15425,#15426,
#15427,#15428,#15429,#15430,#15431,#15432,#15433,#15434,#15435,#15436,#15437,
#15438,#15439,#15440,#15441,#15442,#15443),.UNSPECIFIED.,.F.,.F.,(4,3,3,
3,3,3,3,4),(76.708045941327,76.812995719686,77.8105670926689,78.8081384656519,
79.8057098386348,80.8032812116177,81.8008525846006,82.7984239575836),
 .UNSPECIFIED.);
#1892=B_SPLINE_CURVE_WITH_KNOTS('',3,(#15447,#15448,#15449,#15450,#15451,
#15452,#15453),.UNSPECIFIED.,.F.,.F.,(4,3,4),(-80.7838110923091,-79.8057098386348,
-79.2446069498473),.UNSPECIFIED.);
#1893=B_SPLINE_CURVE_WITH_KNOTS('',3,(#15457,#15458,#15459,#15460,#15461,
#15462,#15463,#15464,#15465,#15466,#15467,#15468,#15469,#15470,#15471,#15472,
#15473,#15474,#15475,#15476,#15477,#15478),.UNSPECIFIED.,.F.,.F.,(4,3,3,
3,3,3,3,4),(-79.2446069498473,-78.8081384656519,-77.8105670926689,-76.812995719686,
-75.815424346703,-74.8178529737201,-73.8202816007372,-72.9614216426678),
 .UNSPECIFIED.);
#1894=B_SPLINE_CURVE_WITH_KNOTS('',3,(#15483,#15484,#15485,#15486,#15487,
#15488,#15489,#15490,#15491,#15492,#15493,#15494,#15495,#15496,#15497,#15498,
#15499,#15500,#15501,#15502,#15503,#15504),.UNSPECIFIED.,.F.,.F.,(4,3,3,
3,3,3,3,4),(70.4248606341475,70.8275674817884,71.8251388547713,72.8227102277542,
73.8202816007372,74.8178529737201,75.815424346703,76.708045941327),
 .UNSPECIFIED.);
#1895=B_SPLINE_CURVE_WITH_KNOTS('',3,(#15505,#15506,#15507,#15508,#15509,
#15510,#15511,#15512,#15513,#15514,#15515,#15516,#15517,#15518,#15519,#15520,
#15521,#15522,#15523,#15524,#15525,#15526,#15527,#15528,#15529),
 .UNSPECIFIED.,.F.,.F.,(4,3,3,3,3,3,3,3,4),(-72.9614216426678,-72.8227102277542,
-71.8251388547713,-70.8275674817884,-69.8299961088054,-68.8324247358225,
-67.8348533628396,-66.8372819898566,-66.6782363354882),.UNSPECIFIED.);
#1896=B_SPLINE_CURVE_WITH_KNOTS('',3,(#15534,#15535,#15536,#15537,#15538,
#15539,#15540,#15541,#15542,#15543,#15544,#15545,#15546,#15547,#15548,#15549,
#15550,#15551,#15552,#15553,#15554,#15555),.UNSPECIFIED.,.F.,.F.,(4,3,3,
3,3,3,3,4),(64.1416753269678,64.8421392438907,65.8397106168737,66.8372819898566,
67.8348533628396,68.8324247358225,69.8299961088054,70.4248606341475),
 .UNSPECIFIED.);
#1897=B_SPLINE_CURVE_WITH_KNOTS('',3,(#15556,#15557,#15558,#15559,#15560,
#15561,#15562,#15563,#15564,#15565,#15566,#15567,#15568,#15569,#15570,#15571,
#15572,#15573,#15574,#15575,#15576,#15577),.UNSPECIFIED.,.F.,.F.,(4,3,3,
3,3,3,3,4),(-66.6782363354882,-65.8397106168737,-64.8421392438908,-63.8445678709078,
-62.8469964979249,-61.849425124942,-60.851853751959,-60.3950510283085),
 .UNSPECIFIED.);
#1898=B_SPLINE_CURVE_WITH_KNOTS('',3,(#15582,#15583,#15584,#15585,#15586,
#15587,#15588,#15589,#15590,#15591,#15592,#15593,#15594,#15595,#15596,#15597,
#15598,#15599,#15600,#15601,#15602,#15603),.UNSPECIFIED.,.F.,.F.,(4,3,3,
3,3,3,3,4),(57.8584900197882,58.8567110059932,59.8542823789761,60.851853751959,
61.849425124942,62.8469964979249,63.8445678709078,64.1416753269678),
 .UNSPECIFIED.);
#1899=B_SPLINE_CURVE_WITH_KNOTS('',3,(#15604,#15605,#15606,#15607,#15608,
#15609,#15610,#15611,#15612,#15613,#15614,#15615,#15616,#15617,#15618,#15619,
#15620,#15621,#15622,#15623,#15624,#15625),.UNSPECIFIED.,.F.,.F.,(4,3,3,
3,3,3,3,4),(-60.3950510283085,-59.8542823789761,-58.8567110059932,-57.8591396330102,
-56.8615682600273,-55.8639968870443,-54.8664255140614,-54.1118657211289),
 .UNSPECIFIED.);
#1900=B_SPLINE_CURVE_WITH_KNOTS('',3,(#15630,#15631,#15632,#15633,#15634,
#15635,#15636,#15637,#15638,#15639,#15640,#15641,#15642,#15643,#15644,#15645,
#15646,#15647,#15648,#15649,#15650,#15651),.UNSPECIFIED.,.F.,.F.,(4,3,3,
3,3,3,3,4),(51.5753047126087,51.8737113951126,52.8712827680955,53.8688541410785,
54.8664255140614,55.8639968870443,56.8615682600273,57.8584900197882),
 .UNSPECIFIED.);
#1901=B_SPLINE_CURVE_WITH_KNOTS('',3,(#15652,#15653,#15654,#15655,#15656,
#15657,#15658,#15659,#15660,#15661,#15662,#15663,#15664,#15665,#15666,#15667,
#15668,#15669,#15670,#15671,#15672,#15673,#15674,#15675,#15676),
 .UNSPECIFIED.,.F.,.F.,(4,3,3,3,3,3,3,3,4),(-54.1118657211289,-53.8688541410785,
-52.8712827680955,-51.8737113951126,-50.8761400221297,-49.8785686491467,
-48.8809972761638,-47.8834259031809,-47.8286804139493),.UNSPECIFIED.);
#1902=B_SPLINE_CURVE_WITH_KNOTS('',3,(#15681,#15682,#15683,#15684,#15685,
#15686,#15687,#15688,#15689,#15690,#15691,#15692,#15693,#15694,#15695,#15696,
#15697,#15698,#15699,#15700,#15701,#15702),.UNSPECIFIED.,.F.,.F.,(4,3,3,
3,3,3,3,4),(45.2921194054291,45.888283157215,46.8858545301979,47.8834259031809,
48.8809972761638,49.8785686491467,50.8761400221297,51.5753047126087),
 .UNSPECIFIED.);
#1903=B_SPLINE_CURVE_WITH_KNOTS('',3,(#15703,#15704,#15705,#15706,#15707,
#15708,#15709,#15710,#15711,#15712,#15713,#15714,#15715,#15716,#15717,#15718,
#15719,#15720,#15721,#15722,#15723,#15724),.UNSPECIFIED.,.F.,.F.,(4,3,3,
3,3,3,3,4),(-47.8286804139493,-46.8858545301979,-45.888283157215,-44.8907117842321,
-43.8931404112491,-42.8955690382662,-41.8979976652833,-41.5454951067698),
 .UNSPECIFIED.);
#1904=B_SPLINE_CURVE_WITH_KNOTS('',3,(#15729,#15730,#15731,#15732,#15733,
#15734,#15735,#15736,#15737,#15738,#15739,#15740,#15741,#15742,#15743,#15744,
#15745,#15746,#15747,#15748,#15749,#15750),.UNSPECIFIED.,.F.,.F.,(4,3,3,
3,3,3,3,4),(39.0089340982495,39.9028549193174,40.9004262923003,41.8979976652833,
42.8955690382662,43.8931404112491,44.8907117842321,45.2921194054291),
 .UNSPECIFIED.);
#1905=B_SPLINE_CURVE_WITH_KNOTS('',3,(#15751,#15752,#15753,#15754,#15755,
#15756,#15757,#15758,#15759,#15760,#15761,#15762,#15763,#15764,#15765,#15766,
#15767,#15768,#15769,#15770,#15771,#15772),.UNSPECIFIED.,.F.,.F.,(4,3,3,
3,3,3,3,4),(-41.5454951067698,-40.9004262923003,-39.9028549193174,-38.9052835463345,
-37.9077121733515,-36.9101408003686,-35.9125694273856,-35.2623097995902),
 .UNSPECIFIED.);
#1906=B_SPLINE_CURVE_WITH_KNOTS('',3,(#15777,#15778,#15779,#15780,#15781,
#15782,#15783,#15784,#15785,#15786,#15787,#15788,#15789,#15790,#15791,#15792,
#15793,#15794,#15795,#15796,#15797,#15798,#15799,#15800,#15801),
 .UNSPECIFIED.,.F.,.F.,(4,3,3,3,3,3,3,3,4),(32.7257487910699,32.9198553084369,
33.9174266814198,34.9149980544027,35.9125694273857,36.9101408003686,37.9077121733515,
38.9052835463345,39.0089340982495),.UNSPECIFIED.);
#1907=B_SPLINE_CURVE_WITH_KNOTS('',3,(#15802,#15803,#15804,#15805,#15806,
#15807,#15808,#15809,#15810,#15811,#15812,#15813,#15814,#15815,#15816,#15817,
#15818,#15819,#15820,#15821,#15822,#15823),.UNSPECIFIED.,.F.,.F.,(4,3,3,
3,3,3,3,4),(-35.2623097995902,-34.9149980544027,-33.9174266814198,-32.9198553084368,
-31.9222839354539,-30.924712562471,-29.927141189488,-28.9791244924106),
 .UNSPECIFIED.);
#1908=B_SPLINE_CURVE_WITH_KNOTS('',3,(#15828,#15829,#15830,#15831,#15832,
#15833,#15834,#15835,#15836,#15837,#15838,#15839,#15840,#15841,#15842,#15843,
#15844,#15845,#15846,#15847,#15848,#15849),.UNSPECIFIED.,.F.,.F.,(4,3,3,
3,3,3,3,4),(26.4425634838903,26.9344270705392,27.9319984435222,28.9295698165051,
29.927141189488,30.924712562471,31.9222839354539,32.7257487910699),
 .UNSPECIFIED.);
#1909=B_SPLINE_CURVE_WITH_KNOTS('',3,(#15850,#15851,#15852,#15853,#15854,
#15855,#15856,#15857,#15858,#15859,#15860,#15861,#15862,#15863,#15864,#15865,
#15866,#15867,#15868,#15869,#15870,#15871,#15872,#15873,#15874),
 .UNSPECIFIED.,.F.,.F.,(4,3,3,3,3,3,3,3,4),(-28.9791244924106,-28.9295698165051,
-27.9319984435222,-26.9344270705392,-25.9368556975563,-24.9392843245734,
-23.9417129515904,-22.9441415786075,-22.695939185231),.UNSPECIFIED.);
#1910=B_SPLINE_CURVE_WITH_KNOTS('',3,(#15879,#15880,#15881,#15882,#15883,
#15884,#15885,#15886,#15887,#15888,#15889,#15890,#15891,#15892,#15893,#15894,
#15895,#15896,#15897,#15898,#15899,#15900),.UNSPECIFIED.,.F.,.F.,(4,3,3,
3,3,3,3,4),(20.1593781767107,20.9489988326416,21.9465702056246,22.9441415786075,
23.9417129515904,24.9392843245734,25.9368556975563,26.4425634838903),
 .UNSPECIFIED.);
#1911=B_SPLINE_CURVE_WITH_KNOTS('',3,(#15901,#15902,#15903,#15904,#15905,
#15906,#15907,#15908,#15909,#15910,#15911,#15912,#15913,#15914,#15915,#15916,
#15917,#15918,#15919,#15920,#15921,#15922),.UNSPECIFIED.,.F.,.F.,(4,3,3,
3,3,3,3,4),(-22.695939185231,-21.9465702056246,-20.9489988326416,-19.9514274596587,
-18.9538560866758,-17.9562847136928,-16.9587133407099,-16.4127538780514),
 .UNSPECIFIED.);
#1912=B_SPLINE_CURVE_WITH_KNOTS('',3,(#15927,#15928,#15929,#15930,#15931,
#15932,#15933,#15934,#15935,#15936,#15937,#15938,#15939,#15940,#15941,#15942,
#15943,#15944,#15945,#15946,#15947,#15948,#15949,#15950,#15951),
 .UNSPECIFIED.,.F.,.F.,(4,3,3,3,3,3,3,3,4),(13.8761928695311,13.9659992217611,
14.963570594744,15.961141967727,16.9587133407099,17.9562847136928,18.9538560866758,
19.9514274596587,20.1593781767107),.UNSPECIFIED.);
#1913=B_SPLINE_CURVE_WITH_KNOTS('',3,(#15952,#15953,#15954,#15955,#15956,
#15957,#15958,#15959,#15960,#15961,#15962,#15963,#15964,#15965,#15966,#15967,
#15968,#15969,#15970,#15971,#15972,#15973),.UNSPECIFIED.,.F.,.F.,(4,3,3,
3,3,3,3,4),(-16.4127538780514,-15.961141967727,-14.963570594744,-13.9659992217611,
-12.9684278487782,-11.9708564757952,-10.9732851028123,-10.1295685708718),
 .UNSPECIFIED.);
#1914=B_SPLINE_CURVE_WITH_KNOTS('',3,(#15979,#15980,#15981,#15982,#15983,
#15984,#15985,#15986,#15987,#15988,#15989,#15990,#15991),.UNSPECIFIED.,
 .F.,.F.,(4,3,3,3,4),(-3.84638326369226,-2.9927141189488,-1.99514274596587,
-0.997571372982934,0.),.UNSPECIFIED.);
#1915=B_SPLINE_CURVE_WITH_KNOTS('',3,(#15994,#15995,#15996,#15997,#15998,
#15999,#16000,#16001,#16002,#16003,#16004,#16005,#16006,#16007,#16008,#16009,
#16010,#16011,#16012),.UNSPECIFIED.,.F.,.F.,(4,3,3,3,3,3,4),(2.01461286527449,
2.99271411894881,3.99028549193174,4.98785686491468,5.98542823789761,6.98299961088054,
7.59300756235157),.UNSPECIFIED.);
#1916=B_SPLINE_CURVE_WITH_KNOTS('',3,(#16018,#16019,#16020,#16021,#16022,
#16023,#16024),.UNSPECIFIED.,.F.,.F.,(4,1,1,1,4),(91.106186954104,91.6672898428915,
92.6648612158744,93.6624325888573,94.6600039618403),.UNSPECIFIED.);
#1917=B_SPLINE_CURVE_WITH_KNOTS('',3,(#16027,#16028,#16029,#16030,#16031,
#16032,#16033,#16034),.UNSPECIFIED.,.F.,.F.,(4,1,1,1,1,4),(91.106186954104,
91.2111367324629,92.2087081054458,93.2062794784288,94.2038508514117,95.181952105086),
 .UNSPECIFIED.);
#1918=B_SPLINE_CURVE_WITH_KNOTS('',3,(#16039,#16040,#16041,#16042,#16043,
#16044,#16045,#16046,#16047,#16048),.UNSPECIFIED.,.F.,.F.,(4,1,1,1,1,1,
1,4),(84.8230016469245,85.6818616049939,86.6794329779768,87.6770043509597,
88.6745757239427,89.6721470969256,90.6697184699085,91.106186954104),
 .UNSPECIFIED.);
#1919=B_SPLINE_CURVE_WITH_KNOTS('',3,(#16049,#16050,#16051,#16052,#16053,
#16054,#16055,#16056,#16057,#16058),.UNSPECIFIED.,.F.,.F.,(4,1,1,1,1,1,
1,4),(84.8230016469244,85.2257084945653,86.2232798675482,87.2208512405312,
88.2184226135141,89.215993986497,90.21356535948,91.106186954104),
 .UNSPECIFIED.);
#1920=B_SPLINE_CURVE_WITH_KNOTS('',3,(#16063,#16064,#16065,#16066,#16067,
#16068,#16069,#16070,#16071,#16072,#16073),.UNSPECIFIED.,.F.,.F.,(4,1,1,
1,1,1,1,1,4),(78.5398163397448,78.6988619941133,79.6964333670962,80.6940047400792,
81.6915761130621,82.689147486045,83.686718859028,84.6842902320109,84.8230016469245),
 .UNSPECIFIED.);
#1921=B_SPLINE_CURVE_WITH_KNOTS('',3,(#16074,#16075,#16076,#16077,#16078,
#16079,#16080,#16081,#16082,#16083),.UNSPECIFIED.,.F.,.F.,(4,1,1,1,1,1,
1,4),(78.5398163397448,79.2402802566677,80.2378516296506,81.2354230026336,
82.2329943756165,83.2305657485994,84.2281371215823,84.8230016469244),
 .UNSPECIFIED.);
#1922=B_SPLINE_CURVE_WITH_KNOTS('',3,(#16088,#16089,#16090,#16091,#16092,
#16093,#16094,#16095,#16096,#16097),.UNSPECIFIED.,.F.,.F.,(4,1,1,1,1,1,
1,4),(72.2566310325652,72.7134337562157,73.7110051291986,74.7085765021816,
75.7061478751645,76.7037192481474,77.7012906211304,78.5398163397448),
 .UNSPECIFIED.);
#1923=B_SPLINE_CURVE_WITH_KNOTS('',3,(#16098,#16099,#16100,#16101,#16102,
#16103,#16104,#16105,#16106,#16107,#16108),.UNSPECIFIED.,.F.,.F.,(4,1,1,
1,1,1,1,1,4),(72.2566310325652,72.2572806457871,73.2548520187701,74.252423391753,
75.2499947647359,76.2475661377189,77.2451375107018,78.2427088836847,78.5398163397448),
 .UNSPECIFIED.);
#1924=B_SPLINE_CURVE_WITH_KNOTS('',3,(#16113,#16114,#16115,#16116,#16117,
#16118,#16119,#16120,#16121,#16122),.UNSPECIFIED.,.F.,.F.,(4,1,1,1,1,1,
1,4),(65.9734457253856,66.7280055183181,67.725576891301,68.723148264284,
69.7207196372669,70.7182910102498,71.7158623832328,72.2566310325652),
 .UNSPECIFIED.);
#1925=B_SPLINE_CURVE_WITH_KNOTS('',3,(#16123,#16124,#16125,#16126,#16127,
#16128,#16129,#16130,#16131,#16132),.UNSPECIFIED.,.F.,.F.,(4,1,1,1,1,1,
1,4),(65.9734457253856,66.2718524078895,67.2694237808725,68.2669951538554,
69.2645665268383,70.2621378998213,71.2597092728042,72.2566310325652),
 .UNSPECIFIED.);
#1926=B_SPLINE_CURVE_WITH_KNOTS('',3,(#16137,#16138,#16139,#16140,#16141,
#16142,#16143,#16144,#16145,#16146,#16147),.UNSPECIFIED.,.F.,.F.,(4,1,1,
1,1,1,1,1,4),(59.690260418206,59.7450059074375,60.7425772804205,61.7401486534034,
62.7377200263864,63.7352913993693,64.7328627723522,65.7304341453352,65.9734457253856),
 .UNSPECIFIED.);
#1927=B_SPLINE_CURVE_WITH_KNOTS('',3,(#16148,#16149,#16150,#16151,#16152,
#16153,#16154,#16155,#16156,#16157),.UNSPECIFIED.,.F.,.F.,(4,1,1,1,1,1,
1,4),(59.690260418206,60.2864241699919,61.2839955429748,62.2815669159578,
63.2791382889407,64.2767096619236,65.2742810349066,65.9734457253856),
 .UNSPECIFIED.);
#1928=B_SPLINE_CURVE_WITH_KNOTS('',3,(#16162,#16163,#16164,#16165,#16166,
#16167,#16168,#16169,#16170,#16171),.UNSPECIFIED.,.F.,.F.,(4,1,1,1,1,1,
1,4),(53.4070751110265,53.7595776695399,54.7571490425229,55.7547204155058,
56.7522917884887,57.7498631614717,58.7474345344546,59.690260418206),
 .UNSPECIFIED.);
#1929=B_SPLINE_CURVE_WITH_KNOTS('',3,(#16172,#16173,#16174,#16175,#16176,
#16177,#16178,#16179,#16180,#16181),.UNSPECIFIED.,.F.,.F.,(4,1,1,1,1,1,
1,4),(53.4070751110264,54.3009959320943,55.2985673050772,56.2961386780602,
57.2937100510431,58.291281424026,59.288852797009,59.690260418206),
 .UNSPECIFIED.);
#1930=B_SPLINE_CURVE_WITH_KNOTS('',3,(#16186,#16187,#16188,#16189,#16190,
#16191,#16192,#16193,#16194,#16195),.UNSPECIFIED.,.F.,.F.,(4,1,1,1,1,1,
1,4),(47.1238898038469,47.7741494316423,48.7717208046253,49.7692921776082,
50.7668635505911,51.7644349235741,52.762006296557,53.4070751110265),
 .UNSPECIFIED.);
#1931=B_SPLINE_CURVE_WITH_KNOTS('',3,(#16196,#16197,#16198,#16199,#16200,
#16201,#16202,#16203,#16204,#16205,#16206),.UNSPECIFIED.,.F.,.F.,(4,1,1,
1,1,1,1,1,4),(47.1238898038469,47.3179963212138,48.3155676941967,49.3131390671796,
50.3107104401626,51.3082818131455,52.3058531861284,53.3034245591114,53.4070751110264),
 .UNSPECIFIED.);
#1932=B_SPLINE_CURVE_WITH_KNOTS('',3,(#16211,#16212,#16213,#16214,#16215,
#16216,#16217,#16218,#16219,#16220),.UNSPECIFIED.,.F.,.F.,(4,1,1,1,1,1,
1,4),(40.8407044966673,41.7887211937447,42.7862925667277,43.7838639397106,
44.7814353126935,45.7790066856765,46.7765780586594,47.1238898038469),
 .UNSPECIFIED.);
#1933=B_SPLINE_CURVE_WITH_KNOTS('',3,(#16221,#16222,#16223,#16224,#16225,
#16226,#16227,#16228,#16229,#16230),.UNSPECIFIED.,.F.,.F.,(4,1,1,1,1,1,
1,4),(40.8407044966673,41.3325680833162,42.3301394562991,43.327710829282,
44.325282202265,45.3228535752479,46.3204249482308,47.1238898038469),
 .UNSPECIFIED.);
#1934=B_SPLINE_CURVE_WITH_KNOTS('',3,(#16235,#16236,#16237,#16238,#16239,
#16240,#16241,#16242,#16243,#16244,#16245),.UNSPECIFIED.,.F.,.F.,(4,1,1,
1,1,1,1,1,4),(34.5575191894876,34.8057215828642,35.8032929558471,36.80086432883,
37.798435701813,38.7960070747959,39.7935784477789,40.7911498207618,40.8407044966673),
 .UNSPECIFIED.);
#1935=B_SPLINE_CURVE_WITH_KNOTS('',3,(#16246,#16247,#16248,#16249,#16250,
#16251,#16252,#16253,#16254,#16255),.UNSPECIFIED.,.F.,.F.,(4,1,1,1,1,1,
1,4),(34.5575191894876,35.3471398454185,36.3447112184015,37.3422825913844,
38.3398539643674,39.3374253373503,40.3349967103332,40.8407044966673),
 .UNSPECIFIED.);
#1936=B_SPLINE_CURVE_WITH_KNOTS('',3,(#16260,#16261,#16262,#16263,#16264,
#16265,#16266,#16267,#16268,#16269),.UNSPECIFIED.,.F.,.F.,(4,1,1,1,1,1,
1,4),(28.2743338823081,28.8202933449666,29.8178647179495,30.8154360909324,
31.8130074639154,32.8105788368983,33.8081502098812,34.5575191894876),
 .UNSPECIFIED.);
#1937=B_SPLINE_CURVE_WITH_KNOTS('',3,(#16270,#16271,#16272,#16273,#16274,
#16275,#16276,#16277,#16278,#16279,#16280),.UNSPECIFIED.,.F.,.F.,(4,1,1,
1,1,1,1,1,4),(28.2743338823081,28.364140234538,29.3617116075209,30.3592829805039,
31.3568543534868,32.3544257264697,33.3519970994527,34.3495684724356,34.5575191894876),
 .UNSPECIFIED.);
#1938=B_SPLINE_CURVE_WITH_KNOTS('',3,(#16285,#16286,#16287,#16288,#16289,
#16290,#16291,#16292,#16293,#16294),.UNSPECIFIED.,.F.,.F.,(4,1,1,1,1,1,
1,4),(21.9911485751285,22.834865107069,23.8324364800519,24.8300078530348,
25.8275792260178,26.8251505990007,27.8227219719836,28.2743338823081),
 .UNSPECIFIED.);
#1939=B_SPLINE_CURVE_WITH_KNOTS('',3,(#16295,#16296,#16297,#16298,#16299,
#16300,#16301,#16302,#16303,#16304),.UNSPECIFIED.,.F.,.F.,(4,1,1,1,1,1,
1,4),(21.9911485751285,22.3787119966404,23.3762833696233,24.3738547426063,
25.3714261155892,26.3689974885721,27.3665688615551,28.2743338823081),
 .UNSPECIFIED.);
#1940=B_SPLINE_CURVE_WITH_KNOTS('',3,(#16310,#16311,#16312,#16313,#16314),
 .UNSPECIFIED.,.F.,.F.,(4,1,4),(14.3981410127769,15.3957123857599,15.7079632679489),
 .UNSPECIFIED.);
#1941=B_SPLINE_CURVE_WITH_KNOTS('',3,(#16317,#16318,#16319,#16320,#16321),
 .UNSPECIFIED.,.F.,.F.,(4,1,4),(13.8761928695312,14.8542941232055,15.7079632679489),
 .UNSPECIFIED.);
#1942=B_SPLINE_CURVE_WITH_KNOTS('',3,(#16404,#16405,#16406,#16407,#16408,
#16409,#16410,#16411,#16412,#16413,#16414,#16415,#16416,#16417,#16418,#16419,
#16420,#16421,#16422,#16423,#16424,#16425,#16426,#16427,#16428,#16429,#16430,
#16431,#16432,#16433,#16434,#16435,#16436,#16437,#16438,#16439,#16440,#16441,
#16442,#16443,#16444,#16445,#16446,#16447,#16448,#16449,#16450,#16451,#16452,
#16453,#16454,#16455,#16456,#16457,#16458),.UNSPECIFIED.,.F.,.F.,(4,3,3,
3,3,3,3,3,3,3,3,3,3,3,3,3,3,3,4),(-0.378621596831442,-0.353562246097462,
-0.339726792951542,-0.324795397581524,-0.299967980662127,-0.289118724731059,
-0.252370044287308,-0.234474300298533,-0.219335629396853,-0.200829495678085,
-0.174827324623006,-0.15584693665932,-0.144923737522316,-0.109696956092963,
-0.0896699638623999,-0.0773387259299598,-0.0372142298588392,-0.00401661180490446,
0.),.UNSPECIFIED.);
#1943=B_SPLINE_CURVE_WITH_KNOTS('',3,(#16459,#16460,#16461,#16462,#16463,
#16464,#16465,#16466,#16467,#16468,#16469,#16470,#16471,#16472,#16473,#16474,
#16475,#16476,#16477,#16478,#16479,#16480,#16481,#16482,#16483,#16484,#16485,
#16486,#16487,#16488,#16489,#16490,#16491,#16492,#16493,#16494,#16495,#16496,
#16497,#16498,#16499,#16500,#16501,#16502,#16503,#16504,#16505,#16506,#16507,
#16508,#16509,#16510,#16511,#16512,#16513),.UNSPECIFIED.,.F.,.F.,(4,3,3,
3,3,3,3,3,3,3,3,3,3,3,3,3,3,3,4),(-0.376940817211619,-0.351602437043448,
-0.332519408379845,-0.318228058131088,-0.288333449384516,-0.272718117105765,
-0.234505377427356,-0.216962131374135,-0.205493408420767,-0.180854828870943,
-0.153734180151122,-0.136643041471865,-0.126205700111191,-0.0954718773410078,
-0.0666269097764766,-0.0558557551097461,-0.0219614248579871,-0.00327040903045905,
0.),.UNSPECIFIED.);
#1944=B_SPLINE_CURVE_WITH_KNOTS('',3,(#16515,#16516,#16517,#16518,#16519,
#16520,#16521,#16522,#16523,#16524,#16525),.UNSPECIFIED.,.F.,.F.,(4,1,1,
1,1,1,1,1,4),(15.7079632679489,15.8518654961884,16.8494368691714,17.8470082421543,
18.8445796151372,19.8421509881202,20.8397223611031,21.837293734086,21.9911485751285),
 .UNSPECIFIED.);
#1945=B_SPLINE_CURVE_WITH_KNOTS('',3,(#16526,#16527,#16528,#16529,#16530,
#16531,#16532,#16533,#16534,#16535),.UNSPECIFIED.,.F.,.F.,(4,1,1,1,1,1,
1,4),(15.7079632679489,16.3932837587428,17.3908551317257,18.3884265047087,
19.3859978776916,20.3835692506745,21.3811406236575,21.9911485751285),
 .UNSPECIFIED.);
#1946=B_SPLINE_CURVE_WITH_KNOTS('',3,(#16880,#16881,#16882,#16883,#16884,
#16885,#16886,#16887,#16888,#16889,#16890,#16891,#16892,#16893,#16894,#16895,
#16896,#16897,#16898,#16899,#16900,#16901,#16902,#16903,#16904,#16905,#16906,
#16907,#16908,#16909,#16910,#16911,#16912,#16913,#16914,#16915,#16916,#16917,
#16918,#16919,#16920,#16921,#16922,#16923,#16924,#16925,#16926,#16927,#16928,
#16929,#16930,#16931),.UNSPECIFIED.,.F.,.F.,(4,3,3,3,3,3,3,3,3,3,3,3,3,
3,3,3,3,4),(0.,0.0336910847235707,0.0587346654534766,0.0734852364994148,
0.109792238871862,0.132864830837164,0.143632030356024,0.17720525627004,
0.195911997060402,0.20761397219,0.244895171883038,0.269599304636634,0.282507756557061,
0.310158174405463,0.327757797512771,0.342580165552076,0.372940760482292,
0.376940817211643),.UNSPECIFIED.);
#1947=B_SPLINE_CURVE_WITH_KNOTS('',3,(#16932,#16933,#16934,#16935,#16936,
#16937,#16938,#16939,#16940,#16941,#16942,#16943,#16944,#16945,#16946,#16947,
#16948,#16949,#16950,#16951,#16952,#16953,#16954,#16955,#16956),
 .UNSPECIFIED.,.F.,.F.,(4,3,3,3,3,3,3,3,4),(-10.1295685708718,-9.97571372982935,
-8.97814235684642,-7.98057098386348,-6.98299961088054,-5.98542823789761,
-4.98785686491468,-3.99028549193174,-3.84638326369226),.UNSPECIFIED.);
#1948=B_SPLINE_CURVE_WITH_KNOTS('',3,(#17301,#17302,#17303,#17304,#17305,
#17306,#17307,#17308,#17309,#17310,#17311,#17312,#17313,#17314,#17315,#17316,
#17317,#17318,#17319,#17320,#17321,#17322),.UNSPECIFIED.,.F.,.F.,(4,3,3,
3,3,3,3,4),(7.59300756235157,7.98057098386348,8.97814235684642,9.97571372982935,
10.9732851028123,11.9708564757952,12.9684278487781,13.8761928695311),
 .UNSPECIFIED.);
#1949=B_SPLINE_CURVE_WITH_KNOTS('',3,(#17323,#17324,#17325,#17326,#17327,
#17328,#17329,#17330,#17331,#17332,#17333,#17334,#17335,#17336,#17337,#17338,
#17339,#17340,#17341,#17342,#17343,#17344,#17345,#17346,#17347,#17348,#17349,
#17350,#17351,#17352,#17353,#17354,#17355,#17356,#17357,#17358,#17359,#17360,
#17361,#17362,#17363,#17364,#17365,#17366,#17367,#17368,#17369,#17370,#17371,
#17372,#17373,#17374),.UNSPECIFIED.,.F.,.F.,(4,3,3,3,3,3,3,3,3,3,3,3,3,
3,3,3,3,4),(0.,0.039679134584082,0.0597937574063347,0.077198275206118,0.0898304469160062,
0.128492621633409,0.153526594220962,0.165101500237275,0.197163594226419,
0.224452129979101,0.234160526966568,0.26945519714964,0.287578609071477,
0.305421511169844,0.333081607138838,0.347224899232131,0.375339207698859,
0.378621596831424),.UNSPECIFIED.);
#1950=B_SPLINE_CURVE_WITH_KNOTS('',3,(#17377,#17378,#17379,#17380,#17381,
#17382,#17383,#17384,#17385,#17386,#17387,#17388,#17389,#17390,#17391,#17392,
#17393,#17394,#17395,#17396,#17397,#17398,#17399,#17400,#17401,#17402,#17403,
#17404,#17405,#17406,#17407,#17408,#17409,#17410,#17411,#17412,#17413,#17414,
#17415,#17416,#17417,#17418,#17419,#17420,#17421,#17422,#17423,#17424,#17425,
#17426,#17427,#17428,#17429,#17430,#17431),.UNSPECIFIED.,.F.,.F.,(4,3,3,
3,3,3,3,3,3,3,3,3,3,3,3,3,3,3,4),(-0.378621596831443,-0.353562246091994,
-0.33972679327765,-0.324795398102486,-0.29996799510237,-0.289118738473772,
-0.252370061457217,-0.234474320899414,-0.219335629080767,-0.200829495678084,
-0.174827314232915,-0.155846896352443,-0.144923681945981,-0.109696914410712,
-0.0896698834676189,-0.0773386968783234,-0.0372142012245099,-0.00401661180490457,
0.),.UNSPECIFIED.);
#1951=B_SPLINE_CURVE_WITH_KNOTS('',3,(#17432,#17433,#17434,#17435,#17436,
#17437,#17438,#17439,#17440,#17441,#17442,#17443,#17444,#17445,#17446,#17447,
#17448,#17449,#17450,#17451,#17452,#17453,#17454,#17455,#17456,#17457,#17458,
#17459,#17460,#17461,#17462,#17463,#17464,#17465,#17466,#17467,#17468,#17469,
#17470,#17471,#17472,#17473,#17474,#17475,#17476,#17477,#17478,#17479,#17480,
#17481,#17482,#17483,#17484,#17485,#17486),.UNSPECIFIED.,.F.,.F.,(4,3,3,
3,3,3,3,3,3,3,3,3,3,3,3,3,3,3,4),(-0.376940817211611,-0.351602437357937,
-0.332519414484987,-0.318228064219006,-0.288333486347302,-0.272718127906801,
-0.234505384447309,-0.21696214863526,-0.205493420723107,-0.180854828870948,
-0.153734168647042,-0.136642926650914,-0.126205451446247,-0.0954716908423004,
-0.0666266083256078,-0.0558556962658209,-0.0219613612575045,-0.00327040903046154,
0.),.UNSPECIFIED.);
#1952=B_SPLINE_CURVE_WITH_KNOTS('',3,(#17488,#17489,#17490,#17491,#17492,
#17493,#17494,#17495,#17496,#17497,#17498),.UNSPECIFIED.,.F.,.F.,(4,1,1,
1,1,1,1,1,4),(15.7079632679489,15.8518654961884,16.8494368691714,17.8470082421543,
18.8445796151372,19.8421509881202,20.8397223611031,21.837293734086,21.9911485751285),
 .UNSPECIFIED.);
#1953=B_SPLINE_CURVE_WITH_KNOTS('',3,(#17499,#17500,#17501,#17502,#17503,
#17504,#17505,#17506,#17507,#17508),.UNSPECIFIED.,.F.,.F.,(4,1,1,1,1,1,
1,4),(15.7079632679489,16.3932837587428,17.3908551317257,18.3884265047087,
19.3859978776916,20.3835692506745,21.3811406236575,21.9911485751285),
 .UNSPECIFIED.);
#1954=B_SPLINE_CURVE_WITH_KNOTS('',3,(#17853,#17854,#17855,#17856,#17857,
#17858,#17859,#17860,#17861,#17862,#17863,#17864,#17865,#17866,#17867,#17868,
#17869,#17870,#17871,#17872,#17873,#17874,#17875,#17876,#17877,#17878,#17879,
#17880,#17881,#17882,#17883,#17884,#17885,#17886,#17887,#17888,#17889,#17890,
#17891,#17892,#17893,#17894,#17895,#17896,#17897,#17898,#17899,#17900,#17901,
#17902,#17903,#17904),.UNSPECIFIED.,.F.,.F.,(4,3,3,3,3,3,3,3,3,3,3,3,3,
3,3,3,3,4),(0.,0.0336910719722371,0.0587346603191241,0.0734852357557152,
0.109792234187795,0.132864822139093,0.143632015204812,0.177205256270034,
0.195911998811098,0.207613973107216,0.244895181060382,0.269599327917347,
0.282507776228681,0.310158203547799,0.327758105582494,0.342580213444175,
0.372940760482282,0.376940817211633),.UNSPECIFIED.);
#1955=B_SPLINE_CURVE_WITH_KNOTS('',3,(#17905,#17906,#17907,#17908,#17909,
#17910,#17911,#17912,#17913,#17914,#17915,#17916,#17917,#17918,#17919,#17920,
#17921,#17922,#17923,#17924,#17925,#17926,#17927,#17928,#17929),
 .UNSPECIFIED.,.F.,.F.,(4,3,3,3,3,3,3,3,4),(-10.1295685708718,-9.97571372982935,
-8.97814235684641,-7.98057098386348,-6.98299961088054,-5.98542823789761,
-4.98785686491467,-3.99028549193174,-3.84638326369226),.UNSPECIFIED.);
#1956=B_SPLINE_CURVE_WITH_KNOTS('',3,(#18274,#18275,#18276,#18277,#18278,
#18279,#18280,#18281,#18282,#18283,#18284,#18285,#18286,#18287,#18288,#18289,
#18290,#18291,#18292,#18293,#18294,#18295),.UNSPECIFIED.,.F.,.F.,(4,3,3,
3,3,3,3,4),(7.59300756235157,7.98057098386348,8.97814235684641,9.97571372982935,
10.9732851028123,11.9708564757952,12.9684278487782,13.8761928695311),
 .UNSPECIFIED.);
#1957=B_SPLINE_CURVE_WITH_KNOTS('',3,(#18296,#18297,#18298,#18299,#18300,
#18301,#18302,#18303,#18304,#18305,#18306,#18307,#18308,#18309,#18310,#18311,
#18312,#18313,#18314,#18315,#18316,#18317,#18318,#18319,#18320,#18321,#18322,
#18323,#18324,#18325,#18326,#18327,#18328,#18329,#18330,#18331,#18332,#18333,
#18334,#18335,#18336,#18337,#18338,#18339,#18340,#18341,#18342,#18343,#18344,
#18345,#18346,#18347),.UNSPECIFIED.,.F.,.F.,(4,3,3,3,3,3,3,3,3,3,3,3,3,
3,3,3,3,4),(0.,0.0396791274481056,0.0597937021224953,0.0771976680457239,
0.0898303082602208,0.12849248988162,0.15352646947755,0.165101472375799,
0.197163594226428,0.224452133325792,0.23416053148377,0.269455200537544,
0.287578557392714,0.305421521052156,0.333081636597174,0.347224904045167,
0.375339207698866,0.378621596831432),.UNSPECIFIED.);
#1958=B_SPLINE_CURVE_WITH_KNOTS('',3,(#18350,#18351,#18352,#18353,#18354,
#18355,#18356,#18357,#18358,#18359,#18360,#18361,#18362,#18363,#18364,#18365,
#18366,#18367,#18368,#18369,#18370,#18371,#18372,#18373,#18374,#18375,#18376,
#18377,#18378,#18379,#18380,#18381,#18382,#18383,#18384,#18385,#18386,#18387,
#18388,#18389,#18390,#18391,#18392,#18393,#18394,#18395,#18396,#18397,#18398,
#18399,#18400,#18401,#18402,#18403,#18404),.UNSPECIFIED.,.F.,.F.,(4,3,3,
3,3,3,3,3,3,3,3,3,3,3,3,3,3,3,4),(-0.378621596831421,-0.353562246109156,
-0.3397267922352,-0.324795396410533,-0.299967947923947,-0.289118693566506,
-0.252370005353849,-0.234474253593686,-0.219335630122499,-0.200829495678059,
-0.174827348196324,-0.155847028127452,-0.144923863657138,-0.109697050694078,
-0.089670146324546,-0.0773387918294275,-0.0372142948109077,-0.00401661180489871,
0.),.UNSPECIFIED.);
#1959=B_SPLINE_CURVE_WITH_KNOTS('',3,(#18405,#18406,#18407,#18408,#18409,
#18410,#18411,#18412,#18413,#18414,#18415,#18416,#18417,#18418,#18419,#18420,
#18421,#18422,#18423,#18424,#18425,#18426,#18427,#18428,#18429,#18430,#18431,
#18432,#18433,#18434,#18435,#18436,#18437,#18438,#18439,#18440,#18441,#18442,
#18443,#18444,#18445,#18446,#18447,#18448,#18449,#18450,#18451,#18452,#18453,
#18454,#18455,#18456,#18457,#18458,#18459),.UNSPECIFIED.,.F.,.F.,(4,3,3,
3,3,3,3,3,3,3,3,3,3,3,3,3,3,3,4),(-0.376940817211661,-0.351602437644044,
-0.332519420023622,-0.318228069756221,-0.288333520013757,-0.272718137738777,
-0.234505390822111,-0.216962164313794,-0.205493431901863,-0.180854828870961,
-0.15373415812608,-0.13664282164838,-0.126205224016848,-0.0954715202702509,
-0.0666263326168646,-0.0558556424387309,-0.0219613030816618,-0.00327040903045922,
0.),.UNSPECIFIED.);
#1960=B_SPLINE_CURVE_WITH_KNOTS('',3,(#18461,#18462,#18463,#18464,#18465,
#18466,#18467,#18468,#18469,#18470,#18471),.UNSPECIFIED.,.F.,.F.,(4,1,1,
1,1,1,1,1,4),(15.7079632679489,15.8518654961884,16.8494368691713,17.8470082421543,
18.8445796151372,19.8421509881201,20.8397223611031,21.837293734086,21.9911485751285),
 .UNSPECIFIED.);
#1961=B_SPLINE_CURVE_WITH_KNOTS('',3,(#18472,#18473,#18474,#18475,#18476,
#18477,#18478,#18479,#18480,#18481),.UNSPECIFIED.,.F.,.F.,(4,1,1,1,1,1,
1,4),(15.7079632679489,16.3932837587428,17.3908551317257,18.3884265047087,
19.3859978776916,20.3835692506745,21.3811406236575,21.9911485751285),
 .UNSPECIFIED.);
#1962=B_SPLINE_CURVE_WITH_KNOTS('',3,(#18826,#18827,#18828,#18829,#18830,
#18831,#18832,#18833,#18834,#18835,#18836,#18837,#18838,#18839,#18840,#18841,
#18842,#18843,#18844,#18845,#18846,#18847,#18848,#18849,#18850,#18851,#18852,
#18853,#18854,#18855,#18856,#18857,#18858,#18859,#18860,#18861,#18862,#18863,
#18864,#18865,#18866,#18867,#18868,#18869,#18870,#18871,#18872,#18873,#18874,
#18875,#18876,#18877),.UNSPECIFIED.,.F.,.F.,(4,3,3,3,3,3,3,3,3,3,3,3,3,
3,3,3,3,4),(0.,0.0336910603093437,0.0587346556237836,0.0734852350726252,
0.109792229900142,0.132864814179886,0.143632001341265,0.177205256270027,
0.195912000411831,0.207613973950097,0.244895189457593,0.269599349217699,
0.282507794231336,0.310158230215905,0.327758387489592,0.342580257274108,
0.372940760482283,0.376940817211633),.UNSPECIFIED.);
#1963=B_SPLINE_CURVE_WITH_KNOTS('',3,(#18878,#18879,#18880,#18881,#18882,
#18883,#18884,#18885,#18886,#18887,#18888,#18889,#18890,#18891,#18892,#18893,
#18894,#18895,#18896,#18897,#18898,#18899,#18900,#18901,#18902),
 .UNSPECIFIED.,.F.,.F.,(4,3,3,3,3,3,3,3,4),(-10.1295685708718,-9.97571372982934,
-8.97814235684641,-7.98057098386347,-6.98299961088054,-5.9854282378976,
-4.98785686491467,-3.99028549193173,-3.84638326369226),.UNSPECIFIED.);
#1964=B_SPLINE_CURVE_WITH_KNOTS('',3,(#19247,#19248,#19249,#19250,#19251,
#19252,#19253,#19254,#19255,#19256,#19257,#19258,#19259,#19260,#19261,#19262,
#19263,#19264,#19265,#19266,#19267,#19268),.UNSPECIFIED.,.F.,.F.,(4,3,3,
3,3,3,3,4),(7.59300756235157,7.98057098386347,8.9781423568464,9.97571372982934,
10.9732851028123,11.9708564757952,12.9684278487781,13.8761928695311),
 .UNSPECIFIED.);
#1965=B_SPLINE_CURVE_WITH_KNOTS('',3,(#19269,#19270,#19271,#19272,#19273,
#19274,#19275,#19276,#19277,#19278,#19279,#19280,#19281,#19282,#19283,#19284,
#19285,#19286,#19287,#19288,#19289,#19290,#19291,#19292,#19293,#19294,#19295,
#19296,#19297,#19298,#19299,#19300,#19301,#19302,#19303,#19304,#19305,#19306,
#19307,#19308,#19309,#19310,#19311,#19312,#19313,#19314,#19315,#19316,#19317,
#19318,#19319,#19320),.UNSPECIFIED.,.F.,.F.,(4,3,3,3,3,3,3,3,3,3,3,3,3,
3,3,3,3,4),(0.,0.0396791507684394,0.0597938827984087,0.0771996525601983,
0.0898307615993676,0.128492920651297,0.153526877334627,0.165101563474246,
0.197163594226425,0.22445212238587,0.234160516714088,0.269455189460283,
0.287578726323234,0.30542148874616,0.333081540294033,0.34722488830939,0.375339207698871,
0.378621596831437),.UNSPECIFIED.);
#1966=B_SPLINE_CURVE_WITH_KNOTS('',3,(#19323,#19324,#19325,#19326,#19327,
#19328,#19329,#19330,#19331,#19332,#19333,#19334,#19335,#19336,#19337,#19338,
#19339,#19340,#19341,#19342,#19343,#19344,#19345,#19346,#19347,#19348,#19349,
#19350,#19351,#19352,#19353,#19354,#19355,#19356,#19357,#19358,#19359,#19360,
#19361,#19362,#19363,#19364,#19365,#19366,#19367,#19368,#19369,#19370,#19371,
#19372,#19373,#19374,#19375,#19376,#19377),.UNSPECIFIED.,.F.,.F.,(4,3,3,
3,3,3,3,3,3,3,3,3,3,3,3,3,3,3,4),(-0.378621596831421,-0.35356224610225,
-0.339726792605717,-0.324795397019123,-0.299967964935665,-0.289118709747788,
-0.252370025571504,-0.234474277842488,-0.219335629751949,-0.200829495678081,
-0.174827335946658,-0.155846980593001,-0.144923798098897,-0.109697001525397,
-0.0896700514919927,-0.0773387576028108,-0.0372142610763827,-0.00401661180489582,
0.),.UNSPECIFIED.);
#1967=B_SPLINE_CURVE_WITH_KNOTS('',3,(#19378,#19379,#19380,#19381,#19382,
#19383,#19384,#19385,#19386,#19387,#19388,#19389,#19390,#19391,#19392,#19393,
#19394,#19395,#19396,#19397,#19398,#19399,#19400,#19401,#19402,#19403,#19404,
#19405,#19406,#19407,#19408,#19409,#19410,#19411,#19412,#19413,#19414,#19415,
#19416,#19417,#19418,#19419,#19420,#19421,#19422,#19423,#19424,#19425,#19426,
#19427,#19428,#19429,#19430,#19431,#19432),.UNSPECIFIED.,.F.,.F.,(4,3,3,
3,3,3,3,3,3,3,3,3,3,3,3,3,3,3,4),(-0.376940817211658,-0.35160243790482,
-0.332519425088979,-0.318228074800829,-0.288333550643748,-0.272718146690274,
-0.234505396639293,-0.21696217861614,-0.205493442096022,-0.18085482887096,
-0.153734148588707,-0.136642726461199,-0.12620501784944,-0.095471365644694,
-0.0666260826793201,-0.0558555936353674,-0.021961250336811,-0.00327040903045685,
0.),.UNSPECIFIED.);
#1968=B_SPLINE_CURVE_WITH_KNOTS('',3,(#19434,#19435,#19436,#19437,#19438,
#19439,#19440,#19441,#19442,#19443,#19444),.UNSPECIFIED.,.F.,.F.,(4,1,1,
1,1,1,1,1,4),(15.7079632679489,15.8518654961884,16.8494368691713,17.8470082421543,
18.8445796151372,19.8421509881202,20.8397223611031,21.837293734086,21.9911485751285),
 .UNSPECIFIED.);
#1969=B_SPLINE_CURVE_WITH_KNOTS('',3,(#19445,#19446,#19447,#19448,#19449,
#19450,#19451,#19452,#19453,#19454),.UNSPECIFIED.,.F.,.F.,(4,1,1,1,1,1,
1,4),(15.7079632679489,16.3932837587428,17.3908551317257,18.3884265047087,
19.3859978776916,20.3835692506745,21.3811406236575,21.9911485751285),
 .UNSPECIFIED.);
#1970=B_SPLINE_CURVE_WITH_KNOTS('',3,(#19799,#19800,#19801,#19802,#19803,
#19804,#19805,#19806,#19807,#19808,#19809,#19810,#19811,#19812,#19813,#19814,
#19815,#19816,#19817,#19818,#19819,#19820,#19821,#19822,#19823,#19824,#19825,
#19826,#19827,#19828,#19829,#19830,#19831,#19832,#19833,#19834,#19835,#19836,
#19837,#19838,#19839,#19840,#19841,#19842,#19843,#19844,#19845,#19846,#19847,
#19848,#19849,#19850),.UNSPECIFIED.,.F.,.F.,(4,3,3,3,3,3,3,3,3,3,3,3,3,
3,3,3,3,4),(0.,0.0336910497355155,0.058734651365868,0.0734852344555961,
0.109792226014928,0.132864806965475,0.143631988775342,0.17720525627004,
0.1959120018626,0.20761397470913,0.244895197064516,0.269599368515367,0.282507810536056,
0.310158254371969,0.327758642889101,0.342580296989548,0.372940760482291,
0.376940817211643),.UNSPECIFIED.);
#1971=B_SPLINE_CURVE_WITH_KNOTS('',3,(#19851,#19852,#19853,#19854,#19855,
#19856,#19857,#19858,#19859,#19860,#19861,#19862,#19863,#19864,#19865,#19866,
#19867,#19868,#19869,#19870,#19871,#19872,#19873,#19874,#19875),
 .UNSPECIFIED.,.F.,.F.,(4,3,3,3,3,3,3,3,4),(-10.1295685708718,-9.97571372982934,
-8.97814235684641,-7.98057098386347,-6.98299961088054,-5.9854282378976,
-4.98785686491467,-3.99028549193173,-3.84638326369226),.UNSPECIFIED.);
#1972=B_SPLINE_CURVE_WITH_KNOTS('',3,(#20220,#20221,#20222,#20223,#20224,
#20225,#20226,#20227,#20228,#20229,#20230,#20231,#20232,#20233,#20234,#20235,
#20236,#20237,#20238,#20239,#20240,#20241),.UNSPECIFIED.,.F.,.F.,(4,3,3,
3,3,3,3,4),(7.59300756235157,7.98057098386347,8.9781423568464,9.97571372982934,
10.9732851028123,11.9708564757952,12.9684278487781,13.8761928695311),
 .UNSPECIFIED.);
#1973=B_SPLINE_CURVE_WITH_KNOTS('',3,(#20242,#20243,#20244,#20245,#20246,
#20247,#20248,#20249,#20250,#20251,#20252,#20253,#20254,#20255,#20256,#20257,
#20258,#20259,#20260,#20261,#20262,#20263,#20264,#20265,#20266,#20267,#20268,
#20269,#20270,#20271,#20272,#20273,#20274,#20275,#20276,#20277,#20278,#20279,
#20280,#20281,#20282,#20283,#20284,#20285,#20286,#20287,#20288,#20289,#20290,
#20291,#20292,#20293),.UNSPECIFIED.,.F.,.F.,(4,3,3,3,3,3,3,3,3,3,3,3,3,
3,3,3,3,4),(0.,0.0396791423592224,0.0597938176449427,0.0771989368507012,
0.0898305980572942,0.128492765250004,0.153526730198623,0.165101530608957,
0.197163594226419,0.224452126331546,0.234160522045081,0.269455193458526,
0.287578665402526,0.305421500398064,0.333081575029239,0.347224893982947,
0.375339207698863,0.378621596831429),.UNSPECIFIED.);
#2445=LINE('',#12705,#3019);
#2446=LINE('',#12740,#3020);
#2447=LINE('',#12767,#3021);
#2448=LINE('',#12818,#3022);
#2449=LINE('',#12866,#3023);
#2450=LINE('',#12914,#3024);
#2451=LINE('',#12965,#3025);
#2452=LINE('',#13013,#3026);
#2453=LINE('',#13061,#3027);
#2454=LINE('',#13112,#3028);
#2455=LINE('',#13163,#3029);
#2456=LINE('',#13211,#3030);
#2457=LINE('',#13262,#3031);
#2458=LINE('',#13301,#3032);
#2459=LINE('',#13323,#3033);
#2460=LINE('',#13347,#3034);
#2461=LINE('',#13372,#3035);
#2462=LINE('',#13397,#3036);
#2463=LINE('',#13421,#3037);
#2464=LINE('',#13446,#3038);
#2465=LINE('',#13470,#3039);
#2466=LINE('',#13495,#3040);
#2467=LINE('',#13519,#3041);
#2468=LINE('',#13544,#3042);
#2469=LINE('',#13569,#3043);
#2470=LINE('',#13593,#3044);
#2471=LINE('',#13610,#3045);
#2472=LINE('',#13645,#3046);
#2473=LINE('',#13672,#3047);
#2474=LINE('',#13723,#3048);
#2475=LINE('',#13771,#3049);
#2476=LINE('',#13819,#3050);
#2477=LINE('',#13870,#3051);
#2478=LINE('',#13918,#3052);
#2479=LINE('',#13966,#3053);
#2480=LINE('',#14017,#3054);
#2481=LINE('',#14068,#3055);
#2482=LINE('',#14116,#3056);
#2483=LINE('',#14167,#3057);
#2484=LINE('',#14206,#3058);
#2485=LINE('',#14228,#3059);
#2486=LINE('',#14252,#3060);
#2487=LINE('',#14277,#3061);
#2488=LINE('',#14302,#3062);
#2489=LINE('',#14326,#3063);
#2490=LINE('',#14351,#3064);
#2491=LINE('',#14375,#3065);
#2492=LINE('',#14400,#3066);
#2493=LINE('',#14424,#3067);
#2494=LINE('',#14449,#3068);
#2495=LINE('',#14474,#3069);
#2496=LINE('',#14498,#3070);
#2497=LINE('',#14515,#3071);
#2498=LINE('',#14550,#3072);
#2499=LINE('',#14577,#3073);
#2500=LINE('',#14628,#3074);
#2501=LINE('',#14676,#3075);
#2502=LINE('',#14724,#3076);
#2503=LINE('',#14775,#3077);
#2504=LINE('',#14823,#3078);
#2505=LINE('',#14871,#3079);
#2506=LINE('',#14922,#3080);
#2507=LINE('',#14973,#3081);
#2508=LINE('',#15021,#3082);
#2509=LINE('',#15072,#3083);
#2510=LINE('',#15111,#3084);
#2511=LINE('',#15133,#3085);
#2512=LINE('',#15157,#3086);
#2513=LINE('',#15182,#3087);
#2514=LINE('',#15207,#3088);
#2515=LINE('',#15231,#3089);
#2516=LINE('',#15256,#3090);
#2517=LINE('',#15280,#3091);
#2518=LINE('',#15305,#3092);
#2519=LINE('',#15329,#3093);
#2520=LINE('',#15354,#3094);
#2521=LINE('',#15379,#3095);
#2522=LINE('',#15403,#3096);
#2523=LINE('',#15420,#3097);
#2524=LINE('',#15455,#3098);
#2525=LINE('',#15482,#3099);
#2526=LINE('',#15533,#3100);
#2527=LINE('',#15581,#3101);
#2528=LINE('',#15629,#3102);
#2529=LINE('',#15680,#3103);
#2530=LINE('',#15728,#3104);
#2531=LINE('',#15776,#3105);
#2532=LINE('',#15827,#3106);
#2533=LINE('',#15878,#3107);
#2534=LINE('',#15926,#3108);
#2535=LINE('',#15977,#3109);
#2536=LINE('',#16016,#3110);
#2537=LINE('',#16038,#3111);
#2538=LINE('',#16062,#3112);
#2539=LINE('',#16087,#3113);
#2540=LINE('',#16112,#3114);
#2541=LINE('',#16136,#3115);
#2542=LINE('',#16161,#3116);
#2543=LINE('',#16185,#3117);
#2544=LINE('',#16210,#3118);
#2545=LINE('',#16234,#3119);
#2546=LINE('',#16259,#3120);
#2547=LINE('',#16284,#3121);
#2548=LINE('',#16308,#3122);
#2549=LINE('',#16327,#3123);
#2550=LINE('',#16330,#3124);
#2551=LINE('',#16333,#3125);
#2552=LINE('',#16335,#3126);
#2553=LINE('',#16336,#3127);
#2554=LINE('',#16341,#3128);
#2555=LINE('',#16345,#3129);
#2556=LINE('',#16347,#3130);
#2557=LINE('',#16348,#3131);
#2558=LINE('',#16354,#3132);
#2559=LINE('',#16357,#3133);
#2560=LINE('',#16359,#3134);
#2561=LINE('',#16361,#3135);
#2562=LINE('',#16371,#3136);
#2563=LINE('',#16372,#3137);
#2564=LINE('',#16380,#3138);
#2565=LINE('',#16389,#3139);
#2566=LINE('',#16391,#3140);
#2567=LINE('',#16400,#3141);
#2568=LINE('',#16402,#3142);
#2569=LINE('',#20303,#3143);
#2570=LINE('',#20309,#3144);
#2571=LINE('',#20314,#3145);
#2572=LINE('',#20316,#3146);
#2573=LINE('',#20318,#3147);
#2574=LINE('',#20319,#3148);
#2575=LINE('',#20322,#3149);
#2576=LINE('',#20324,#3150);
#2577=LINE('',#20325,#3151);
#2578=LINE('',#20328,#3152);
#2579=LINE('',#20330,#3153);
#2580=LINE('',#20331,#3154);
#2581=LINE('',#20333,#3155);
#2582=LINE('',#20337,#3156);
#2583=LINE('',#20339,#3157);
#2584=LINE('',#20341,#3158);
#2585=LINE('',#20342,#3159);
#2586=LINE('',#20346,#3160);
#2587=LINE('',#20348,#3161);
#2588=LINE('',#20350,#3162);
#2589=LINE('',#20351,#3163);
#2590=LINE('',#20353,#3164);
#2591=LINE('',#20354,#3165);
#2592=LINE('',#20356,#3166);
#2593=LINE('',#20361,#3167);
#2594=LINE('',#20366,#3168);
#2595=LINE('',#20369,#3169);
#2596=LINE('',#20374,#3170);
#2597=LINE('',#20376,#3171);
#2598=LINE('',#20378,#3172);
#2599=LINE('',#20379,#3173);
#2600=LINE('',#20381,#3174);
#2601=LINE('',#20383,#3175);
#2602=LINE('',#20385,#3176);
#2603=LINE('',#20386,#3177);
#2604=LINE('',#20389,#3178);
#2605=LINE('',#20391,#3179);
#2606=LINE('',#20392,#3180);
#2607=LINE('',#20394,#3181);
#2608=LINE('',#20395,#3182);
#2609=LINE('',#20396,#3183);
#3019=VECTOR('',#10696,0.2);
#3020=VECTOR('',#10699,0.2);
#3021=VECTOR('',#10704,0.2);
#3022=VECTOR('',#10707,0.2);
#3023=VECTOR('',#10710,0.2);
#3024=VECTOR('',#10713,0.2);
#3025=VECTOR('',#10716,0.2);
#3026=VECTOR('',#10719,0.2);
#3027=VECTOR('',#10722,0.2);
#3028=VECTOR('',#10725,0.2);
#3029=VECTOR('',#10728,0.2);
#3030=VECTOR('',#10731,0.2);
#3031=VECTOR('',#10734,0.2);
#3032=VECTOR('',#10739,0.205475);
#3033=VECTOR('',#10744,0.205475);
#3034=VECTOR('',#10747,0.205475);
#3035=VECTOR('',#10750,0.205475);
#3036=VECTOR('',#10753,0.205475);
#3037=VECTOR('',#10756,0.205475);
#3038=VECTOR('',#10759,0.205475);
#3039=VECTOR('',#10762,0.205475);
#3040=VECTOR('',#10765,0.205475);
#3041=VECTOR('',#10768,0.205475);
#3042=VECTOR('',#10771,0.205475);
#3043=VECTOR('',#10774,0.205475);
#3044=VECTOR('',#10777,0.205475);
#3045=VECTOR('',#10782,0.2);
#3046=VECTOR('',#10785,0.2);
#3047=VECTOR('',#10790,0.2);
#3048=VECTOR('',#10793,0.2);
#3049=VECTOR('',#10796,0.2);
#3050=VECTOR('',#10799,0.2);
#3051=VECTOR('',#10802,0.2);
#3052=VECTOR('',#10805,0.2);
#3053=VECTOR('',#10808,0.2);
#3054=VECTOR('',#10811,0.2);
#3055=VECTOR('',#10814,0.2);
#3056=VECTOR('',#10817,0.2);
#3057=VECTOR('',#10820,0.2);
#3058=VECTOR('',#10825,0.205475000000001);
#3059=VECTOR('',#10830,0.205475000000001);
#3060=VECTOR('',#10833,0.205475000000001);
#3061=VECTOR('',#10836,0.205475000000001);
#3062=VECTOR('',#10839,0.205475000000001);
#3063=VECTOR('',#10842,0.205475000000001);
#3064=VECTOR('',#10845,0.205475000000001);
#3065=VECTOR('',#10848,0.205475000000001);
#3066=VECTOR('',#10851,0.205475000000001);
#3067=VECTOR('',#10854,0.205475000000001);
#3068=VECTOR('',#10857,0.205475000000001);
#3069=VECTOR('',#10860,0.205475000000001);
#3070=VECTOR('',#10863,0.205475000000001);
#3071=VECTOR('',#10868,0.2);
#3072=VECTOR('',#10871,0.2);
#3073=VECTOR('',#10876,0.2);
#3074=VECTOR('',#10879,0.2);
#3075=VECTOR('',#10882,0.2);
#3076=VECTOR('',#10885,0.2);
#3077=VECTOR('',#10888,0.2);
#3078=VECTOR('',#10891,0.2);
#3079=VECTOR('',#10894,0.2);
#3080=VECTOR('',#10897,0.2);
#3081=VECTOR('',#10900,0.2);
#3082=VECTOR('',#10903,0.2);
#3083=VECTOR('',#10906,0.2);
#3084=VECTOR('',#10911,0.205475000000001);
#3085=VECTOR('',#10916,0.205475000000001);
#3086=VECTOR('',#10919,0.205475000000001);
#3087=VECTOR('',#10922,0.205475000000001);
#3088=VECTOR('',#10925,0.205475000000001);
#3089=VECTOR('',#10928,0.205475000000001);
#3090=VECTOR('',#10931,0.205475000000001);
#3091=VECTOR('',#10934,0.205475000000001);
#3092=VECTOR('',#10937,0.205475000000001);
#3093=VECTOR('',#10940,0.205475000000001);
#3094=VECTOR('',#10943,0.205475000000001);
#3095=VECTOR('',#10946,0.205475000000001);
#3096=VECTOR('',#10949,0.205475000000001);
#3097=VECTOR('',#10954,0.2);
#3098=VECTOR('',#10957,0.2);
#3099=VECTOR('',#10962,0.2);
#3100=VECTOR('',#10965,0.2);
#3101=VECTOR('',#10968,0.2);
#3102=VECTOR('',#10971,0.2);
#3103=VECTOR('',#10974,0.2);
#3104=VECTOR('',#10977,0.2);
#3105=VECTOR('',#10980,0.2);
#3106=VECTOR('',#10983,0.2);
#3107=VECTOR('',#10986,0.2);
#3108=VECTOR('',#10989,0.2);
#3109=VECTOR('',#10992,0.2);
#3110=VECTOR('',#10997,0.205475);
#3111=VECTOR('',#11002,0.205475);
#3112=VECTOR('',#11005,0.205475);
#3113=VECTOR('',#11008,0.205475);
#3114=VECTOR('',#11011,0.205475);
#3115=VECTOR('',#11014,0.205475);
#3116=VECTOR('',#11017,0.205475);
#3117=VECTOR('',#11020,0.205475);
#3118=VECTOR('',#11023,0.205475);
#3119=VECTOR('',#11026,0.205475);
#3120=VECTOR('',#11029,0.205475);
#3121=VECTOR('',#11032,0.205475);
#3122=VECTOR('',#11035,0.205475);
#3123=VECTOR('',#11042,1.);
#3124=VECTOR('',#11045,1.);
#3125=VECTOR('',#11048,1.);
#3126=VECTOR('',#11049,1.);
#3127=VECTOR('',#11050,1.);
#3128=VECTOR('',#11055,1.);
#3129=VECTOR('',#11060,1.);
#3130=VECTOR('',#11061,1.);
#3131=VECTOR('',#11062,1.);
#3132=VECTOR('',#11067,1.);
#3133=VECTOR('',#11070,1.);
#3134=VECTOR('',#11073,1.);
#3135=VECTOR('',#11074,1.);
#3136=VECTOR('',#11085,1.);
#3137=VECTOR('',#11086,1.);
#3138=VECTOR('',#11097,0.6);
#3139=VECTOR('',#11108,0.4);
#3140=VECTOR('',#11111,0.25);
#3141=VECTOR('',#11122,0.4);
#3142=VECTOR('',#11125,0.25);
#3143=VECTOR('',#11162,0.3);
#3144=VECTOR('',#11169,0.3);
#3145=VECTOR('',#11174,1.);
#3146=VECTOR('',#11175,1.);
#3147=VECTOR('',#11176,1.);
#3148=VECTOR('',#11177,1.);
#3149=VECTOR('',#11180,1.);
#3150=VECTOR('',#11181,1.);
#3151=VECTOR('',#11182,1.);
#3152=VECTOR('',#11185,1.);
#3153=VECTOR('',#11186,1.);
#3154=VECTOR('',#11187,1.);
#3155=VECTOR('',#11190,1.);
#3156=VECTOR('',#11193,1.);
#3157=VECTOR('',#11194,1.);
#3158=VECTOR('',#11195,1.);
#3159=VECTOR('',#11196,1.);
#3160=VECTOR('',#11199,1.);
#3161=VECTOR('',#11200,1.);
#3162=VECTOR('',#11201,1.);
#3163=VECTOR('',#11202,1.);
#3164=VECTOR('',#11205,1.);
#3165=VECTOR('',#11206,1.);
#3166=VECTOR('',#11209,1.);
#3167=VECTOR('',#11214,0.65);
#3168=VECTOR('',#11221,0.8);
#3169=VECTOR('',#11226,1.);
#3170=VECTOR('',#11231,1.);
#3171=VECTOR('',#11232,1.);
#3172=VECTOR('',#11233,1.);
#3173=VECTOR('',#11234,1.);
#3174=VECTOR('',#11237,1.);
#3175=VECTOR('',#11238,1.);
#3176=VECTOR('',#11239,1.);
#3177=VECTOR('',#11240,1.);
#3178=VECTOR('',#11243,1.);
#3179=VECTOR('',#11244,1.);
#3180=VECTOR('',#11245,1.);
#3181=VECTOR('',#11248,1.);
#3182=VECTOR('',#11249,1.);
#3183=VECTOR('',#11250,1.);
#3593=VERTEX_POINT('',#12703);
#3594=VERTEX_POINT('',#12704);
#3595=VERTEX_POINT('',#12706);
#3596=VERTEX_POINT('',#12729);
#3597=VERTEX_POINT('',#12731);
#3598=VERTEX_POINT('',#12739);
#3599=VERTEX_POINT('',#12765);
#3600=VERTEX_POINT('',#12766);
#3601=VERTEX_POINT('',#12816);
#3602=VERTEX_POINT('',#12817);
#3603=VERTEX_POINT('',#12864);
#3604=VERTEX_POINT('',#12865);
#3605=VERTEX_POINT('',#12912);
#3606=VERTEX_POINT('',#12913);
#3607=VERTEX_POINT('',#12963);
#3608=VERTEX_POINT('',#12964);
#3609=VERTEX_POINT('',#13011);
#3610=VERTEX_POINT('',#13012);
#3611=VERTEX_POINT('',#13059);
#3612=VERTEX_POINT('',#13060);
#3613=VERTEX_POINT('',#13110);
#3614=VERTEX_POINT('',#13111);
#3615=VERTEX_POINT('',#13161);
#3616=VERTEX_POINT('',#13162);
#3617=VERTEX_POINT('',#13209);
#3618=VERTEX_POINT('',#13210);
#3619=VERTEX_POINT('',#13260);
#3620=VERTEX_POINT('',#13261);
#3621=VERTEX_POINT('',#13263);
#3622=VERTEX_POINT('',#13277);
#3623=VERTEX_POINT('',#13299);
#3624=VERTEX_POINT('',#13300);
#3625=VERTEX_POINT('',#13302);
#3626=VERTEX_POINT('',#13310);
#3627=VERTEX_POINT('',#13321);
#3628=VERTEX_POINT('',#13322);
#3629=VERTEX_POINT('',#13345);
#3630=VERTEX_POINT('',#13346);
#3631=VERTEX_POINT('',#13370);
#3632=VERTEX_POINT('',#13371);
#3633=VERTEX_POINT('',#13395);
#3634=VERTEX_POINT('',#13396);
#3635=VERTEX_POINT('',#13419);
#3636=VERTEX_POINT('',#13420);
#3637=VERTEX_POINT('',#13444);
#3638=VERTEX_POINT('',#13445);
#3639=VERTEX_POINT('',#13468);
#3640=VERTEX_POINT('',#13469);
#3641=VERTEX_POINT('',#13493);
#3642=VERTEX_POINT('',#13494);
#3643=VERTEX_POINT('',#13517);
#3644=VERTEX_POINT('',#13518);
#3645=VERTEX_POINT('',#13542);
#3646=VERTEX_POINT('',#13543);
#3647=VERTEX_POINT('',#13567);
#3648=VERTEX_POINT('',#13568);
#3649=VERTEX_POINT('',#13591);
#3650=VERTEX_POINT('',#13592);
#3651=VERTEX_POINT('',#13594);
#3652=VERTEX_POINT('',#13600);
#3653=VERTEX_POINT('',#13608);
#3654=VERTEX_POINT('',#13609);
#3655=VERTEX_POINT('',#13611);
#3656=VERTEX_POINT('',#13634);
#3657=VERTEX_POINT('',#13636);
#3658=VERTEX_POINT('',#13644);
#3659=VERTEX_POINT('',#13670);
#3660=VERTEX_POINT('',#13671);
#3661=VERTEX_POINT('',#13721);
#3662=VERTEX_POINT('',#13722);
#3663=VERTEX_POINT('',#13769);
#3664=VERTEX_POINT('',#13770);
#3665=VERTEX_POINT('',#13817);
#3666=VERTEX_POINT('',#13818);
#3667=VERTEX_POINT('',#13868);
#3668=VERTEX_POINT('',#13869);
#3669=VERTEX_POINT('',#13916);
#3670=VERTEX_POINT('',#13917);
#3671=VERTEX_POINT('',#13964);
#3672=VERTEX_POINT('',#13965);
#3673=VERTEX_POINT('',#14015);
#3674=VERTEX_POINT('',#14016);
#3675=VERTEX_POINT('',#14066);
#3676=VERTEX_POINT('',#14067);
#3677=VERTEX_POINT('',#14114);
#3678=VERTEX_POINT('',#14115);
#3679=VERTEX_POINT('',#14165);
#3680=VERTEX_POINT('',#14166);
#3681=VERTEX_POINT('',#14168);
#3682=VERTEX_POINT('',#14182);
#3683=VERTEX_POINT('',#14204);
#3684=VERTEX_POINT('',#14205);
#3685=VERTEX_POINT('',#14207);
#3686=VERTEX_POINT('',#14215);
#3687=VERTEX_POINT('',#14226);
#3688=VERTEX_POINT('',#14227);
#3689=VERTEX_POINT('',#14250);
#3690=VERTEX_POINT('',#14251);
#3691=VERTEX_POINT('',#14275);
#3692=VERTEX_POINT('',#14276);
#3693=VERTEX_POINT('',#14300);
#3694=VERTEX_POINT('',#14301);
#3695=VERTEX_POINT('',#14324);
#3696=VERTEX_POINT('',#14325);
#3697=VERTEX_POINT('',#14349);
#3698=VERTEX_POINT('',#14350);
#3699=VERTEX_POINT('',#14373);
#3700=VERTEX_POINT('',#14374);
#3701=VERTEX_POINT('',#14398);
#3702=VERTEX_POINT('',#14399);
#3703=VERTEX_POINT('',#14422);
#3704=VERTEX_POINT('',#14423);
#3705=VERTEX_POINT('',#14447);
#3706=VERTEX_POINT('',#14448);
#3707=VERTEX_POINT('',#14472);
#3708=VERTEX_POINT('',#14473);
#3709=VERTEX_POINT('',#14496);
#3710=VERTEX_POINT('',#14497);
#3711=VERTEX_POINT('',#14499);
#3712=VERTEX_POINT('',#14505);
#3713=VERTEX_POINT('',#14513);
#3714=VERTEX_POINT('',#14514);
#3715=VERTEX_POINT('',#14516);
#3716=VERTEX_POINT('',#14539);
#3717=VERTEX_POINT('',#14541);
#3718=VERTEX_POINT('',#14549);
#3719=VERTEX_POINT('',#14575);
#3720=VERTEX_POINT('',#14576);
#3721=VERTEX_POINT('',#14626);
#3722=VERTEX_POINT('',#14627);
#3723=VERTEX_POINT('',#14674);
#3724=VERTEX_POINT('',#14675);
#3725=VERTEX_POINT('',#14722);
#3726=VERTEX_POINT('',#14723);
#3727=VERTEX_POINT('',#14773);
#3728=VERTEX_POINT('',#14774);
#3729=VERTEX_POINT('',#14821);
#3730=VERTEX_POINT('',#14822);
#3731=VERTEX_POINT('',#14869);
#3732=VERTEX_POINT('',#14870);
#3733=VERTEX_POINT('',#14920);
#3734=VERTEX_POINT('',#14921);
#3735=VERTEX_POINT('',#14971);
#3736=VERTEX_POINT('',#14972);
#3737=VERTEX_POINT('',#15019);
#3738=VERTEX_POINT('',#15020);
#3739=VERTEX_POINT('',#15070);
#3740=VERTEX_POINT('',#15071);
#3741=VERTEX_POINT('',#15073);
#3742=VERTEX_POINT('',#15087);
#3743=VERTEX_POINT('',#15109);
#3744=VERTEX_POINT('',#15110);
#3745=VERTEX_POINT('',#15112);
#3746=VERTEX_POINT('',#15120);
#3747=VERTEX_POINT('',#15131);
#3748=VERTEX_POINT('',#15132);
#3749=VERTEX_POINT('',#15155);
#3750=VERTEX_POINT('',#15156);
#3751=VERTEX_POINT('',#15180);
#3752=VERTEX_POINT('',#15181);
#3753=VERTEX_POINT('',#15205);
#3754=VERTEX_POINT('',#15206);
#3755=VERTEX_POINT('',#15229);
#3756=VERTEX_POINT('',#15230);
#3757=VERTEX_POINT('',#15254);
#3758=VERTEX_POINT('',#15255);
#3759=VERTEX_POINT('',#15278);
#3760=VERTEX_POINT('',#15279);
#3761=VERTEX_POINT('',#15303);
#3762=VERTEX_POINT('',#15304);
#3763=VERTEX_POINT('',#15327);
#3764=VERTEX_POINT('',#15328);
#3765=VERTEX_POINT('',#15352);
#3766=VERTEX_POINT('',#15353);
#3767=VERTEX_POINT('',#15377);
#3768=VERTEX_POINT('',#15378);
#3769=VERTEX_POINT('',#15401);
#3770=VERTEX_POINT('',#15402);
#3771=VERTEX_POINT('',#15404);
#3772=VERTEX_POINT('',#15410);
#3773=VERTEX_POINT('',#15418);
#3774=VERTEX_POINT('',#15419);
#3775=VERTEX_POINT('',#15421);
#3776=VERTEX_POINT('',#15444);
#3777=VERTEX_POINT('',#15446);
#3778=VERTEX_POINT('',#15454);
#3779=VERTEX_POINT('',#15480);
#3780=VERTEX_POINT('',#15481);
#3781=VERTEX_POINT('',#15531);
#3782=VERTEX_POINT('',#15532);
#3783=VERTEX_POINT('',#15579);
#3784=VERTEX_POINT('',#15580);
#3785=VERTEX_POINT('',#15627);
#3786=VERTEX_POINT('',#15628);
#3787=VERTEX_POINT('',#15678);
#3788=VERTEX_POINT('',#15679);
#3789=VERTEX_POINT('',#15726);
#3790=VERTEX_POINT('',#15727);
#3791=VERTEX_POINT('',#15774);
#3792=VERTEX_POINT('',#15775);
#3793=VERTEX_POINT('',#15825);
#3794=VERTEX_POINT('',#15826);
#3795=VERTEX_POINT('',#15876);
#3796=VERTEX_POINT('',#15877);
#3797=VERTEX_POINT('',#15924);
#3798=VERTEX_POINT('',#15925);
#3799=VERTEX_POINT('',#15975);
#3800=VERTEX_POINT('',#15976);
#3801=VERTEX_POINT('',#15978);
#3802=VERTEX_POINT('',#15992);
#3803=VERTEX_POINT('',#16014);
#3804=VERTEX_POINT('',#16015);
#3805=VERTEX_POINT('',#16017);
#3806=VERTEX_POINT('',#16025);
#3807=VERTEX_POINT('',#16036);
#3808=VERTEX_POINT('',#16037);
#3809=VERTEX_POINT('',#16060);
#3810=VERTEX_POINT('',#16061);
#3811=VERTEX_POINT('',#16085);
#3812=VERTEX_POINT('',#16086);
#3813=VERTEX_POINT('',#16110);
#3814=VERTEX_POINT('',#16111);
#3815=VERTEX_POINT('',#16134);
#3816=VERTEX_POINT('',#16135);
#3817=VERTEX_POINT('',#16159);
#3818=VERTEX_POINT('',#16160);
#3819=VERTEX_POINT('',#16183);
#3820=VERTEX_POINT('',#16184);
#3821=VERTEX_POINT('',#16208);
#3822=VERTEX_POINT('',#16209);
#3823=VERTEX_POINT('',#16232);
#3824=VERTEX_POINT('',#16233);
#3825=VERTEX_POINT('',#16257);
#3826=VERTEX_POINT('',#16258);
#3827=VERTEX_POINT('',#16282);
#3828=VERTEX_POINT('',#16283);
#3829=VERTEX_POINT('',#16306);
#3830=VERTEX_POINT('',#16307);
#3831=VERTEX_POINT('',#16309);
#3832=VERTEX_POINT('',#16315);
#3833=VERTEX_POINT('',#16323);
#3834=VERTEX_POINT('',#16324);
#3835=VERTEX_POINT('',#16326);
#3836=VERTEX_POINT('',#16328);
#3837=VERTEX_POINT('',#16332);
#3838=VERTEX_POINT('',#16334);
#3839=VERTEX_POINT('',#16338);
#3840=VERTEX_POINT('',#16340);
#3841=VERTEX_POINT('',#16344);
#3842=VERTEX_POINT('',#16346);
#3843=VERTEX_POINT('',#16350);
#3844=VERTEX_POINT('',#16351);
#3845=VERTEX_POINT('',#16353);
#3846=VERTEX_POINT('',#16355);
#3847=VERTEX_POINT('',#16360);
#3848=VERTEX_POINT('',#16363);
#3849=VERTEX_POINT('',#16365);
#3850=VERTEX_POINT('',#16367);
#3851=VERTEX_POINT('',#16370);
#3852=VERTEX_POINT('',#16373);
#3853=VERTEX_POINT('',#16378);
#3854=VERTEX_POINT('',#16382);
#3855=VERTEX_POINT('',#16384);
#3856=VERTEX_POINT('',#16387);
#3857=VERTEX_POINT('',#16393);
#3858=VERTEX_POINT('',#16395);
#3859=VERTEX_POINT('',#16398);
#3860=VERTEX_POINT('',#20300);
#3861=VERTEX_POINT('',#20302);
#3862=VERTEX_POINT('',#20306);
#3863=VERTEX_POINT('',#20308);
#3864=VERTEX_POINT('',#20312);
#3865=VERTEX_POINT('',#20313);
#3866=VERTEX_POINT('',#20315);
#3867=VERTEX_POINT('',#20317);
#3868=VERTEX_POINT('',#20321);
#3869=VERTEX_POINT('',#20323);
#3870=VERTEX_POINT('',#20327);
#3871=VERTEX_POINT('',#20329);
#3872=VERTEX_POINT('',#20335);
#3873=VERTEX_POINT('',#20336);
#3874=VERTEX_POINT('',#20338);
#3875=VERTEX_POINT('',#20340);
#3876=VERTEX_POINT('',#20344);
#3877=VERTEX_POINT('',#20345);
#3878=VERTEX_POINT('',#20347);
#3879=VERTEX_POINT('',#20349);
#3880=VERTEX_POINT('',#20358);
#3881=VERTEX_POINT('',#20360);
#3882=VERTEX_POINT('',#20364);
#3883=VERTEX_POINT('',#20372);
#3884=VERTEX_POINT('',#20373);
#3885=VERTEX_POINT('',#20375);
#3886=VERTEX_POINT('',#20377);
#3887=VERTEX_POINT('',#20382);
#3888=VERTEX_POINT('',#20384);
#3889=VERTEX_POINT('',#20388);
#3890=VERTEX_POINT('',#20390);
#4549=EDGE_CURVE('',#3593,#3594,#2445,.T.);
#4550=EDGE_CURVE('',#3594,#3595,#1738,.T.);
#4551=EDGE_CURVE('',#3595,#3596,#1582,.T.);
#4552=EDGE_CURVE('',#3596,#3597,#1739,.T.);
#4553=EDGE_CURVE('',#3597,#3598,#2446,.T.);
#4554=EDGE_CURVE('',#3598,#3598,#1583,.F.);
#4555=EDGE_CURVE('',#3597,#3593,#1740,.T.);
#4556=EDGE_CURVE('',#3599,#3600,#2447,.T.);
#4557=EDGE_CURVE('',#3600,#3594,#1741,.T.);
#4558=EDGE_CURVE('',#3593,#3599,#1742,.T.);
#4559=EDGE_CURVE('',#3601,#3602,#2448,.T.);
#4560=EDGE_CURVE('',#3602,#3600,#1743,.T.);
#4561=EDGE_CURVE('',#3599,#3601,#1744,.T.);
#4562=EDGE_CURVE('',#3603,#3604,#2449,.T.);
#4563=EDGE_CURVE('',#3604,#3602,#1745,.T.);
#4564=EDGE_CURVE('',#3601,#3603,#1746,.T.);
#4565=EDGE_CURVE('',#3605,#3606,#2450,.T.);
#4566=EDGE_CURVE('',#3606,#3604,#1747,.T.);
#4567=EDGE_CURVE('',#3603,#3605,#1748,.T.);
#4568=EDGE_CURVE('',#3607,#3608,#2451,.T.);
#4569=EDGE_CURVE('',#3608,#3606,#1749,.T.);
#4570=EDGE_CURVE('',#3605,#3607,#1750,.T.);
#4571=EDGE_CURVE('',#3609,#3610,#2452,.T.);
#4572=EDGE_CURVE('',#3610,#3608,#1751,.T.);
#4573=EDGE_CURVE('',#3607,#3609,#1752,.T.);
#4574=EDGE_CURVE('',#3611,#3612,#2453,.T.);
#4575=EDGE_CURVE('',#3612,#3610,#1753,.T.);
#4576=EDGE_CURVE('',#3609,#3611,#1754,.T.);
#4577=EDGE_CURVE('',#3613,#3614,#2454,.T.);
#4578=EDGE_CURVE('',#3614,#3612,#1755,.T.);
#4579=EDGE_CURVE('',#3611,#3613,#1756,.T.);
#4580=EDGE_CURVE('',#3615,#3616,#2455,.T.);
#4581=EDGE_CURVE('',#3616,#3614,#1757,.T.);
#4582=EDGE_CURVE('',#3613,#3615,#1758,.T.);
#4583=EDGE_CURVE('',#3617,#3618,#2456,.T.);
#4584=EDGE_CURVE('',#3618,#3616,#1759,.T.);
#4585=EDGE_CURVE('',#3615,#3617,#1760,.T.);
#4586=EDGE_CURVE('',#3619,#3620,#2457,.T.);
#4587=EDGE_CURVE('',#3619,#3621,#1761,.T.);
#4588=EDGE_CURVE('',#3622,#3621,#1584,.T.);
#4589=EDGE_CURVE('',#3622,#3620,#1762,.T.);
#4590=EDGE_CURVE('',#3623,#3624,#2458,.T.);
#4591=EDGE_CURVE('',#3624,#3625,#1763,.T.);
#4592=EDGE_CURVE('',#3626,#3625,#1585,.T.);
#4593=EDGE_CURVE('',#3623,#3626,#1764,.T.);
#4594=EDGE_CURVE('',#3627,#3628,#2459,.T.);
#4595=EDGE_CURVE('',#3628,#3624,#1765,.T.);
#4596=EDGE_CURVE('',#3627,#3623,#1766,.T.);
#4597=EDGE_CURVE('',#3629,#3630,#2460,.T.);
#4598=EDGE_CURVE('',#3630,#3628,#1767,.T.);
#4599=EDGE_CURVE('',#3629,#3627,#1768,.T.);
#4600=EDGE_CURVE('',#3631,#3632,#2461,.T.);
#4601=EDGE_CURVE('',#3632,#3630,#1769,.T.);
#4602=EDGE_CURVE('',#3631,#3629,#1770,.T.);
#4603=EDGE_CURVE('',#3633,#3634,#2462,.T.);
#4604=EDGE_CURVE('',#3634,#3632,#1771,.T.);
#4605=EDGE_CURVE('',#3633,#3631,#1772,.T.);
#4606=EDGE_CURVE('',#3635,#3636,#2463,.T.);
#4607=EDGE_CURVE('',#3636,#3634,#1773,.T.);
#4608=EDGE_CURVE('',#3635,#3633,#1774,.T.);
#4609=EDGE_CURVE('',#3637,#3638,#2464,.T.);
#4610=EDGE_CURVE('',#3638,#3636,#1775,.T.);
#4611=EDGE_CURVE('',#3637,#3635,#1776,.T.);
#4612=EDGE_CURVE('',#3639,#3640,#2465,.T.);
#4613=EDGE_CURVE('',#3640,#3638,#1777,.T.);
#4614=EDGE_CURVE('',#3639,#3637,#1778,.T.);
#4615=EDGE_CURVE('',#3641,#3642,#2466,.T.);
#4616=EDGE_CURVE('',#3642,#3640,#1779,.T.);
#4617=EDGE_CURVE('',#3641,#3639,#1780,.T.);
#4618=EDGE_CURVE('',#3643,#3644,#2467,.T.);
#4619=EDGE_CURVE('',#3644,#3642,#1781,.T.);
#4620=EDGE_CURVE('',#3643,#3641,#1782,.T.);
#4621=EDGE_CURVE('',#3645,#3646,#2468,.T.);
#4622=EDGE_CURVE('',#3646,#3644,#1783,.T.);
#4623=EDGE_CURVE('',#3645,#3643,#1784,.T.);
#4624=EDGE_CURVE('',#3647,#3648,#2469,.T.);
#4625=EDGE_CURVE('',#3648,#3646,#1785,.T.);
#4626=EDGE_CURVE('',#3647,#3645,#1786,.T.);
#4627=EDGE_CURVE('',#3649,#3650,#2470,.T.);
#4628=EDGE_CURVE('',#3651,#3649,#1787,.T.);
#4629=EDGE_CURVE('',#3652,#3651,#1586,.T.);
#4630=EDGE_CURVE('',#3652,#3650,#1788,.T.);
#4631=EDGE_CURVE('',#3653,#3654,#2471,.T.);
#4632=EDGE_CURVE('',#3654,#3655,#1789,.T.);
#4633=EDGE_CURVE('',#3655,#3656,#1587,.T.);
#4634=EDGE_CURVE('',#3656,#3657,#1790,.T.);
#4635=EDGE_CURVE('',#3657,#3658,#2472,.T.);
#4636=EDGE_CURVE('',#3658,#3658,#1588,.F.);
#4637=EDGE_CURVE('',#3657,#3653,#1791,.T.);
#4638=EDGE_CURVE('',#3659,#3660,#2473,.T.);
#4639=EDGE_CURVE('',#3660,#3654,#1792,.T.);
#4640=EDGE_CURVE('',#3653,#3659,#1793,.T.);
#4641=EDGE_CURVE('',#3661,#3662,#2474,.T.);
#4642=EDGE_CURVE('',#3662,#3660,#1794,.T.);
#4643=EDGE_CURVE('',#3659,#3661,#1795,.T.);
#4644=EDGE_CURVE('',#3663,#3664,#2475,.T.);
#4645=EDGE_CURVE('',#3664,#3662,#1796,.T.);
#4646=EDGE_CURVE('',#3661,#3663,#1797,.T.);
#4647=EDGE_CURVE('',#3665,#3666,#2476,.T.);
#4648=EDGE_CURVE('',#3666,#3664,#1798,.T.);
#4649=EDGE_CURVE('',#3663,#3665,#1799,.T.);
#4650=EDGE_CURVE('',#3667,#3668,#2477,.T.);
#4651=EDGE_CURVE('',#3668,#3666,#1800,.T.);
#4652=EDGE_CURVE('',#3665,#3667,#1801,.T.);
#4653=EDGE_CURVE('',#3669,#3670,#2478,.T.);
#4654=EDGE_CURVE('',#3670,#3668,#1802,.T.);
#4655=EDGE_CURVE('',#3667,#3669,#1803,.T.);
#4656=EDGE_CURVE('',#3671,#3672,#2479,.T.);
#4657=EDGE_CURVE('',#3672,#3670,#1804,.T.);
#4658=EDGE_CURVE('',#3669,#3671,#1805,.T.);
#4659=EDGE_CURVE('',#3673,#3674,#2480,.T.);
#4660=EDGE_CURVE('',#3674,#3672,#1806,.T.);
#4661=EDGE_CURVE('',#3671,#3673,#1807,.T.);
#4662=EDGE_CURVE('',#3675,#3676,#2481,.T.);
#4663=EDGE_CURVE('',#3676,#3674,#1808,.T.);
#4664=EDGE_CURVE('',#3673,#3675,#1809,.T.);
#4665=EDGE_CURVE('',#3677,#3678,#2482,.T.);
#4666=EDGE_CURVE('',#3678,#3676,#1810,.T.);
#4667=EDGE_CURVE('',#3675,#3677,#1811,.T.);
#4668=EDGE_CURVE('',#3679,#3680,#2483,.T.);
#4669=EDGE_CURVE('',#3679,#3681,#1812,.T.);
#4670=EDGE_CURVE('',#3682,#3681,#1589,.T.);
#4671=EDGE_CURVE('',#3682,#3680,#1813,.T.);
#4672=EDGE_CURVE('',#3683,#3684,#2484,.T.);
#4673=EDGE_CURVE('',#3684,#3685,#1814,.T.);
#4674=EDGE_CURVE('',#3686,#3685,#1590,.T.);
#4675=EDGE_CURVE('',#3683,#3686,#1815,.T.);
#4676=EDGE_CURVE('',#3687,#3688,#2485,.T.);
#4677=EDGE_CURVE('',#3688,#3684,#1816,.T.);
#4678=EDGE_CURVE('',#3687,#3683,#1817,.T.);
#4679=EDGE_CURVE('',#3689,#3690,#2486,.T.);
#4680=EDGE_CURVE('',#3690,#3688,#1818,.T.);
#4681=EDGE_CURVE('',#3689,#3687,#1819,.T.);
#4682=EDGE_CURVE('',#3691,#3692,#2487,.T.);
#4683=EDGE_CURVE('',#3692,#3690,#1820,.T.);
#4684=EDGE_CURVE('',#3691,#3689,#1821,.T.);
#4685=EDGE_CURVE('',#3693,#3694,#2488,.T.);
#4686=EDGE_CURVE('',#3694,#3692,#1822,.T.);
#4687=EDGE_CURVE('',#3693,#3691,#1823,.T.);
#4688=EDGE_CURVE('',#3695,#3696,#2489,.T.);
#4689=EDGE_CURVE('',#3696,#3694,#1824,.T.);
#4690=EDGE_CURVE('',#3695,#3693,#1825,.T.);
#4691=EDGE_CURVE('',#3697,#3698,#2490,.T.);
#4692=EDGE_CURVE('',#3698,#3696,#1826,.T.);
#4693=EDGE_CURVE('',#3697,#3695,#1827,.T.);
#4694=EDGE_CURVE('',#3699,#3700,#2491,.T.);
#4695=EDGE_CURVE('',#3700,#3698,#1828,.T.);
#4696=EDGE_CURVE('',#3699,#3697,#1829,.T.);
#4697=EDGE_CURVE('',#3701,#3702,#2492,.T.);
#4698=EDGE_CURVE('',#3702,#3700,#1830,.T.);
#4699=EDGE_CURVE('',#3701,#3699,#1831,.T.);
#4700=EDGE_CURVE('',#3703,#3704,#2493,.T.);
#4701=EDGE_CURVE('',#3704,#3702,#1832,.T.);
#4702=EDGE_CURVE('',#3703,#3701,#1833,.T.);
#4703=EDGE_CURVE('',#3705,#3706,#2494,.T.);
#4704=EDGE_CURVE('',#3706,#3704,#1834,.T.);
#4705=EDGE_CURVE('',#3705,#3703,#1835,.T.);
#4706=EDGE_CURVE('',#3707,#3708,#2495,.T.);
#4707=EDGE_CURVE('',#3708,#3706,#1836,.T.);
#4708=EDGE_CURVE('',#3707,#3705,#1837,.T.);
#4709=EDGE_CURVE('',#3709,#3710,#2496,.T.);
#4710=EDGE_CURVE('',#3711,#3709,#1838,.T.);
#4711=EDGE_CURVE('',#3712,#3711,#1591,.T.);
#4712=EDGE_CURVE('',#3712,#3710,#1839,.T.);
#4713=EDGE_CURVE('',#3713,#3714,#2497,.T.);
#4714=EDGE_CURVE('',#3714,#3715,#1840,.T.);
#4715=EDGE_CURVE('',#3715,#3716,#1592,.T.);
#4716=EDGE_CURVE('',#3716,#3717,#1841,.T.);
#4717=EDGE_CURVE('',#3717,#3718,#2498,.T.);
#4718=EDGE_CURVE('',#3718,#3718,#1593,.F.);
#4719=EDGE_CURVE('',#3717,#3713,#1842,.T.);
#4720=EDGE_CURVE('',#3719,#3720,#2499,.T.);
#4721=EDGE_CURVE('',#3720,#3714,#1843,.T.);
#4722=EDGE_CURVE('',#3713,#3719,#1844,.T.);
#4723=EDGE_CURVE('',#3721,#3722,#2500,.T.);
#4724=EDGE_CURVE('',#3722,#3720,#1845,.T.);
#4725=EDGE_CURVE('',#3719,#3721,#1846,.T.);
#4726=EDGE_CURVE('',#3723,#3724,#2501,.T.);
#4727=EDGE_CURVE('',#3724,#3722,#1847,.T.);
#4728=EDGE_CURVE('',#3721,#3723,#1848,.T.);
#4729=EDGE_CURVE('',#3725,#3726,#2502,.T.);
#4730=EDGE_CURVE('',#3726,#3724,#1849,.T.);
#4731=EDGE_CURVE('',#3723,#3725,#1850,.T.);
#4732=EDGE_CURVE('',#3727,#3728,#2503,.T.);
#4733=EDGE_CURVE('',#3728,#3726,#1851,.T.);
#4734=EDGE_CURVE('',#3725,#3727,#1852,.T.);
#4735=EDGE_CURVE('',#3729,#3730,#2504,.T.);
#4736=EDGE_CURVE('',#3730,#3728,#1853,.T.);
#4737=EDGE_CURVE('',#3727,#3729,#1854,.T.);
#4738=EDGE_CURVE('',#3731,#3732,#2505,.T.);
#4739=EDGE_CURVE('',#3732,#3730,#1855,.T.);
#4740=EDGE_CURVE('',#3729,#3731,#1856,.T.);
#4741=EDGE_CURVE('',#3733,#3734,#2506,.T.);
#4742=EDGE_CURVE('',#3734,#3732,#1857,.T.);
#4743=EDGE_CURVE('',#3731,#3733,#1858,.T.);
#4744=EDGE_CURVE('',#3735,#3736,#2507,.T.);
#4745=EDGE_CURVE('',#3736,#3734,#1859,.T.);
#4746=EDGE_CURVE('',#3733,#3735,#1860,.T.);
#4747=EDGE_CURVE('',#3737,#3738,#2508,.T.);
#4748=EDGE_CURVE('',#3738,#3736,#1861,.T.);
#4749=EDGE_CURVE('',#3735,#3737,#1862,.T.);
#4750=EDGE_CURVE('',#3739,#3740,#2509,.T.);
#4751=EDGE_CURVE('',#3739,#3741,#1863,.T.);
#4752=EDGE_CURVE('',#3742,#3741,#1594,.T.);
#4753=EDGE_CURVE('',#3742,#3740,#1864,.T.);
#4754=EDGE_CURVE('',#3743,#3744,#2510,.T.);
#4755=EDGE_CURVE('',#3744,#3745,#1865,.T.);
#4756=EDGE_CURVE('',#3746,#3745,#1595,.T.);
#4757=EDGE_CURVE('',#3743,#3746,#1866,.T.);
#4758=EDGE_CURVE('',#3747,#3748,#2511,.T.);
#4759=EDGE_CURVE('',#3748,#3744,#1867,.T.);
#4760=EDGE_CURVE('',#3747,#3743,#1868,.T.);
#4761=EDGE_CURVE('',#3749,#3750,#2512,.T.);
#4762=EDGE_CURVE('',#3750,#3748,#1869,.T.);
#4763=EDGE_CURVE('',#3749,#3747,#1870,.T.);
#4764=EDGE_CURVE('',#3751,#3752,#2513,.T.);
#4765=EDGE_CURVE('',#3752,#3750,#1871,.T.);
#4766=EDGE_CURVE('',#3751,#3749,#1872,.T.);
#4767=EDGE_CURVE('',#3753,#3754,#2514,.T.);
#4768=EDGE_CURVE('',#3754,#3752,#1873,.T.);
#4769=EDGE_CURVE('',#3753,#3751,#1874,.T.);
#4770=EDGE_CURVE('',#3755,#3756,#2515,.T.);
#4771=EDGE_CURVE('',#3756,#3754,#1875,.T.);
#4772=EDGE_CURVE('',#3755,#3753,#1876,.T.);
#4773=EDGE_CURVE('',#3757,#3758,#2516,.T.);
#4774=EDGE_CURVE('',#3758,#3756,#1877,.T.);
#4775=EDGE_CURVE('',#3757,#3755,#1878,.T.);
#4776=EDGE_CURVE('',#3759,#3760,#2517,.T.);
#4777=EDGE_CURVE('',#3760,#3758,#1879,.T.);
#4778=EDGE_CURVE('',#3759,#3757,#1880,.T.);
#4779=EDGE_CURVE('',#3761,#3762,#2518,.T.);
#4780=EDGE_CURVE('',#3762,#3760,#1881,.T.);
#4781=EDGE_CURVE('',#3761,#3759,#1882,.T.);
#4782=EDGE_CURVE('',#3763,#3764,#2519,.T.);
#4783=EDGE_CURVE('',#3764,#3762,#1883,.T.);
#4784=EDGE_CURVE('',#3763,#3761,#1884,.T.);
#4785=EDGE_CURVE('',#3765,#3766,#2520,.T.);
#4786=EDGE_CURVE('',#3766,#3764,#1885,.T.);
#4787=EDGE_CURVE('',#3765,#3763,#1886,.T.);
#4788=EDGE_CURVE('',#3767,#3768,#2521,.T.);
#4789=EDGE_CURVE('',#3768,#3766,#1887,.T.);
#4790=EDGE_CURVE('',#3767,#3765,#1888,.T.);
#4791=EDGE_CURVE('',#3769,#3770,#2522,.T.);
#4792=EDGE_CURVE('',#3771,#3769,#1889,.T.);
#4793=EDGE_CURVE('',#3772,#3771,#1596,.T.);
#4794=EDGE_CURVE('',#3772,#3770,#1890,.T.);
#4795=EDGE_CURVE('',#3773,#3774,#2523,.T.);
#4796=EDGE_CURVE('',#3774,#3775,#1891,.T.);
#4797=EDGE_CURVE('',#3775,#3776,#1597,.T.);
#4798=EDGE_CURVE('',#3776,#3777,#1892,.T.);
#4799=EDGE_CURVE('',#3777,#3778,#2524,.T.);
#4800=EDGE_CURVE('',#3778,#3778,#1598,.F.);
#4801=EDGE_CURVE('',#3777,#3773,#1893,.T.);
#4802=EDGE_CURVE('',#3779,#3780,#2525,.T.);
#4803=EDGE_CURVE('',#3780,#3774,#1894,.T.);
#4804=EDGE_CURVE('',#3773,#3779,#1895,.T.);
#4805=EDGE_CURVE('',#3781,#3782,#2526,.T.);
#4806=EDGE_CURVE('',#3782,#3780,#1896,.T.);
#4807=EDGE_CURVE('',#3779,#3781,#1897,.T.);
#4808=EDGE_CURVE('',#3783,#3784,#2527,.T.);
#4809=EDGE_CURVE('',#3784,#3782,#1898,.T.);
#4810=EDGE_CURVE('',#3781,#3783,#1899,.T.);
#4811=EDGE_CURVE('',#3785,#3786,#2528,.T.);
#4812=EDGE_CURVE('',#3786,#3784,#1900,.T.);
#4813=EDGE_CURVE('',#3783,#3785,#1901,.T.);
#4814=EDGE_CURVE('',#3787,#3788,#2529,.T.);
#4815=EDGE_CURVE('',#3788,#3786,#1902,.T.);
#4816=EDGE_CURVE('',#3785,#3787,#1903,.T.);
#4817=EDGE_CURVE('',#3789,#3790,#2530,.T.);
#4818=EDGE_CURVE('',#3790,#3788,#1904,.T.);
#4819=EDGE_CURVE('',#3787,#3789,#1905,.T.);
#4820=EDGE_CURVE('',#3791,#3792,#2531,.T.);
#4821=EDGE_CURVE('',#3792,#3790,#1906,.T.);
#4822=EDGE_CURVE('',#3789,#3791,#1907,.T.);
#4823=EDGE_CURVE('',#3793,#3794,#2532,.T.);
#4824=EDGE_CURVE('',#3794,#3792,#1908,.T.);
#4825=EDGE_CURVE('',#3791,#3793,#1909,.T.);
#4826=EDGE_CURVE('',#3795,#3796,#2533,.T.);
#4827=EDGE_CURVE('',#3796,#3794,#1910,.T.);
#4828=EDGE_CURVE('',#3793,#3795,#1911,.T.);
#4829=EDGE_CURVE('',#3797,#3798,#2534,.T.);
#4830=EDGE_CURVE('',#3798,#3796,#1912,.T.);
#4831=EDGE_CURVE('',#3795,#3797,#1913,.T.);
#4832=EDGE_CURVE('',#3799,#3800,#2535,.T.);
#4833=EDGE_CURVE('',#3799,#3801,#1914,.T.);
#4834=EDGE_CURVE('',#3802,#3801,#1599,.T.);
#4835=EDGE_CURVE('',#3802,#3800,#1915,.T.);
#4836=EDGE_CURVE('',#3803,#3804,#2536,.T.);
#4837=EDGE_CURVE('',#3804,#3805,#1916,.T.);
#4838=EDGE_CURVE('',#3806,#3805,#1600,.T.);
#4839=EDGE_CURVE('',#3803,#3806,#1917,.T.);
#4840=EDGE_CURVE('',#3807,#3808,#2537,.T.);
#4841=EDGE_CURVE('',#3808,#3804,#1918,.T.);
#4842=EDGE_CURVE('',#3807,#3803,#1919,.T.);
#4843=EDGE_CURVE('',#3809,#3810,#2538,.T.);
#4844=EDGE_CURVE('',#3810,#3808,#1920,.T.);
#4845=EDGE_CURVE('',#3809,#3807,#1921,.T.);
#4846=EDGE_CURVE('',#3811,#3812,#2539,.T.);
#4847=EDGE_CURVE('',#3812,#3810,#1922,.T.);
#4848=EDGE_CURVE('',#3811,#3809,#1923,.T.);
#4849=EDGE_CURVE('',#3813,#3814,#2540,.T.);
#4850=EDGE_CURVE('',#3814,#3812,#1924,.T.);
#4851=EDGE_CURVE('',#3813,#3811,#1925,.T.);
#4852=EDGE_CURVE('',#3815,#3816,#2541,.T.);
#4853=EDGE_CURVE('',#3816,#3814,#1926,.T.);
#4854=EDGE_CURVE('',#3815,#3813,#1927,.T.);
#4855=EDGE_CURVE('',#3817,#3818,#2542,.T.);
#4856=EDGE_CURVE('',#3818,#3816,#1928,.T.);
#4857=EDGE_CURVE('',#3817,#3815,#1929,.T.);
#4858=EDGE_CURVE('',#3819,#3820,#2543,.T.);
#4859=EDGE_CURVE('',#3820,#3818,#1930,.T.);
#4860=EDGE_CURVE('',#3819,#3817,#1931,.T.);
#4861=EDGE_CURVE('',#3821,#3822,#2544,.T.);
#4862=EDGE_CURVE('',#3822,#3820,#1932,.T.);
#4863=EDGE_CURVE('',#3821,#3819,#1933,.T.);
#4864=EDGE_CURVE('',#3823,#3824,#2545,.T.);
#4865=EDGE_CURVE('',#3824,#3822,#1934,.T.);
#4866=EDGE_CURVE('',#3823,#3821,#1935,.T.);
#4867=EDGE_CURVE('',#3825,#3826,#2546,.T.);
#4868=EDGE_CURVE('',#3826,#3824,#1936,.T.);
#4869=EDGE_CURVE('',#3825,#3823,#1937,.T.);
#4870=EDGE_CURVE('',#3827,#3828,#2547,.T.);
#4871=EDGE_CURVE('',#3828,#3826,#1938,.T.);
#4872=EDGE_CURVE('',#3827,#3825,#1939,.T.);
#4873=EDGE_CURVE('',#3829,#3830,#2548,.T.);
#4874=EDGE_CURVE('',#3831,#3829,#1940,.T.);
#4875=EDGE_CURVE('',#3832,#3831,#1601,.T.);
#4876=EDGE_CURVE('',#3832,#3830,#1941,.T.);
#4877=EDGE_CURVE('',#3833,#3834,#1602,.T.);
#4878=EDGE_CURVE('',#3833,#3835,#2549,.T.);
#4879=EDGE_CURVE('',#3835,#3836,#1603,.T.);
#4880=EDGE_CURVE('',#3836,#3834,#2550,.T.);
#4881=EDGE_CURVE('',#3833,#3837,#2551,.T.);
#4882=EDGE_CURVE('',#3838,#3837,#2552,.T.);
#4883=EDGE_CURVE('',#3835,#3838,#2553,.T.);
#4884=EDGE_CURVE('',#3839,#3837,#1604,.T.);
#4885=EDGE_CURVE('',#3839,#3840,#2554,.T.);
#4886=EDGE_CURVE('',#3840,#3838,#1605,.T.);
#4887=EDGE_CURVE('',#3839,#3841,#2555,.T.);
#4888=EDGE_CURVE('',#3842,#3841,#2556,.T.);
#4889=EDGE_CURVE('',#3840,#3842,#2557,.T.);
#4890=EDGE_CURVE('',#3843,#3844,#1606,.T.);
#4891=EDGE_CURVE('',#3843,#3845,#2558,.T.);
#4892=EDGE_CURVE('',#3845,#3846,#1607,.T.);
#4893=EDGE_CURVE('',#3846,#3844,#2559,.T.);
#4894=EDGE_CURVE('',#3843,#3834,#2560,.T.);
#4895=EDGE_CURVE('',#3847,#3844,#2561,.T.);
#4896=EDGE_CURVE('',#3847,#3841,#1608,.T.);
#4897=EDGE_CURVE('',#3848,#3848,#1609,.T.);
#4898=EDGE_CURVE('',#3849,#3849,#1610,.T.);
#4899=EDGE_CURVE('',#3850,#3850,#1611,.T.);
#4900=EDGE_CURVE('',#3851,#3846,#2562,.T.);
#4901=EDGE_CURVE('',#3847,#3851,#2563,.T.);
#4902=EDGE_CURVE('',#3852,#3852,#1612,.T.);
#4903=EDGE_CURVE('',#3851,#3842,#1613,.T.);
#4904=EDGE_CURVE('',#3853,#3853,#1614,.T.);
#4905=EDGE_CURVE('',#3853,#3852,#2564,.T.);
#4906=EDGE_CURVE('',#3854,#3854,#1615,.T.);
#4907=EDGE_CURVE('',#3855,#3855,#1616,.T.);
#4908=EDGE_CURVE('',#3856,#3856,#1617,.T.);
#4909=EDGE_CURVE('',#3856,#3854,#2565,.T.);
#4910=EDGE_CURVE('',#3855,#3850,#2566,.T.);
#4911=EDGE_CURVE('',#3857,#3857,#1618,.T.);
#4912=EDGE_CURVE('',#3858,#3858,#1619,.T.);
#4913=EDGE_CURVE('',#3859,#3859,#1620,.T.);
#4914=EDGE_CURVE('',#3859,#3857,#2567,.T.);
#4915=EDGE_CURVE('',#3858,#3849,#2568,.T.);
#4916=EDGE_CURVE('',#3775,#3806,#1942,.T.);
#4917=EDGE_CURVE('',#3805,#3776,#1943,.T.);
#4918=EDGE_CURVE('',#3830,#3828,#1944,.T.);
#4919=EDGE_CURVE('',#3829,#3827,#1945,.T.);
#4920=EDGE_CURVE('',#3801,#3832,#1946,.T.);
#4921=EDGE_CURVE('',#3797,#3799,#1947,.T.);
#4922=EDGE_CURVE('',#3800,#3798,#1948,.T.);
#4923=EDGE_CURVE('',#3831,#3802,#1949,.T.);
#4924=EDGE_CURVE('',#3715,#3746,#1950,.T.);
#4925=EDGE_CURVE('',#3745,#3716,#1951,.T.);
#4926=EDGE_CURVE('',#3770,#3768,#1952,.T.);
#4927=EDGE_CURVE('',#3769,#3767,#1953,.T.);
#4928=EDGE_CURVE('',#3741,#3772,#1954,.T.);
#4929=EDGE_CURVE('',#3737,#3739,#1955,.T.);
#4930=EDGE_CURVE('',#3740,#3738,#1956,.T.);
#4931=EDGE_CURVE('',#3771,#3742,#1957,.T.);
#4932=EDGE_CURVE('',#3655,#3686,#1958,.T.);
#4933=EDGE_CURVE('',#3685,#3656,#1959,.T.);
#4934=EDGE_CURVE('',#3710,#3708,#1960,.T.);
#4935=EDGE_CURVE('',#3709,#3707,#1961,.T.);
#4936=EDGE_CURVE('',#3681,#3712,#1962,.T.);
#4937=EDGE_CURVE('',#3677,#3679,#1963,.T.);
#4938=EDGE_CURVE('',#3680,#3678,#1964,.T.);
#4939=EDGE_CURVE('',#3711,#3682,#1965,.T.);
#4940=EDGE_CURVE('',#3595,#3626,#1966,.T.);
#4941=EDGE_CURVE('',#3625,#3596,#1967,.T.);
#4942=EDGE_CURVE('',#3650,#3648,#1968,.T.);
#4943=EDGE_CURVE('',#3649,#3647,#1969,.T.);
#4944=EDGE_CURVE('',#3621,#3652,#1970,.T.);
#4945=EDGE_CURVE('',#3617,#3619,#1971,.T.);
#4946=EDGE_CURVE('',#3620,#3618,#1972,.T.);
#4947=EDGE_CURVE('',#3651,#3622,#1973,.T.);
#4948=EDGE_CURVE('',#3860,#3860,#1621,.T.);
#4949=EDGE_CURVE('',#3860,#3861,#2569,.T.);
#4950=EDGE_CURVE('',#3861,#3861,#1622,.T.);
#4951=EDGE_CURVE('',#3862,#3862,#1623,.T.);
#4952=EDGE_CURVE('',#3862,#3863,#2570,.T.);
#4953=EDGE_CURVE('',#3863,#3863,#1624,.T.);
#4954=EDGE_CURVE('',#3864,#3865,#2571,.T.);
#4955=EDGE_CURVE('',#3866,#3865,#2572,.T.);
#4956=EDGE_CURVE('',#3867,#3866,#2573,.T.);
#4957=EDGE_CURVE('',#3864,#3867,#2574,.T.);
#4958=EDGE_CURVE('',#3868,#3864,#2575,.T.);
#4959=EDGE_CURVE('',#3869,#3867,#2576,.T.);
#4960=EDGE_CURVE('',#3868,#3869,#2577,.T.);
#4961=EDGE_CURVE('',#3870,#3868,#2578,.T.);
#4962=EDGE_CURVE('',#3871,#3869,#2579,.T.);
#4963=EDGE_CURVE('',#3870,#3871,#2580,.T.);
#4964=EDGE_CURVE('',#3871,#3866,#2581,.T.);
#4965=EDGE_CURVE('',#3872,#3873,#2582,.T.);
#4966=EDGE_CURVE('',#3873,#3874,#2583,.T.);
#4967=EDGE_CURVE('',#3875,#3874,#2584,.T.);
#4968=EDGE_CURVE('',#3872,#3875,#2585,.T.);
#4969=EDGE_CURVE('',#3876,#3877,#2586,.T.);
#4970=EDGE_CURVE('',#3878,#3877,#2587,.T.);
#4971=EDGE_CURVE('',#3879,#3878,#2588,.T.);
#4972=EDGE_CURVE('',#3876,#3879,#2589,.T.);
#4973=EDGE_CURVE('',#3873,#3876,#2590,.T.);
#4974=EDGE_CURVE('',#3874,#3879,#2591,.T.);
#4975=EDGE_CURVE('',#3875,#3878,#2592,.T.);
#4976=EDGE_CURVE('',#3880,#3880,#1625,.T.);
#4977=EDGE_CURVE('',#3880,#3881,#2593,.T.);
#4978=EDGE_CURVE('',#3881,#3881,#1626,.T.);
#4979=EDGE_CURVE('',#3882,#3882,#1627,.T.);
#4980=EDGE_CURVE('',#3882,#3848,#2594,.T.);
#4981=EDGE_CURVE('',#3845,#3836,#2595,.T.);
#4982=EDGE_CURVE('',#3883,#3884,#2596,.T.);
#4983=EDGE_CURVE('',#3884,#3885,#2597,.T.);
#4984=EDGE_CURVE('',#3886,#3885,#2598,.T.);
#4985=EDGE_CURVE('',#3883,#3886,#2599,.T.);
#4986=EDGE_CURVE('',#3865,#3883,#2600,.T.);
#4987=EDGE_CURVE('',#3887,#3886,#2601,.T.);
#4988=EDGE_CURVE('',#3888,#3887,#2602,.T.);
#4989=EDGE_CURVE('',#3888,#3870,#2603,.T.);
#4990=EDGE_CURVE('',#3889,#3888,#2604,.T.);
#4991=EDGE_CURVE('',#3890,#3887,#2605,.T.);
#4992=EDGE_CURVE('',#3889,#3890,#2606,.T.);
#4993=EDGE_CURVE('',#3877,#3889,#2607,.T.);
#4994=EDGE_CURVE('',#3885,#3890,#2608,.T.);
#4995=EDGE_CURVE('',#3884,#3872,#2609,.T.);
#5986=ORIENTED_EDGE('',*,*,#4549,.T.);
#5987=ORIENTED_EDGE('',*,*,#4550,.T.);
#5988=ORIENTED_EDGE('',*,*,#4551,.T.);
#5989=ORIENTED_EDGE('',*,*,#4552,.T.);
#5990=ORIENTED_EDGE('',*,*,#4553,.T.);
#5991=ORIENTED_EDGE('',*,*,#4554,.T.);
#5992=ORIENTED_EDGE('',*,*,#4553,.F.);
#5993=ORIENTED_EDGE('',*,*,#4555,.T.);
#5994=ORIENTED_EDGE('',*,*,#4556,.T.);
#5995=ORIENTED_EDGE('',*,*,#4557,.T.);
#5996=ORIENTED_EDGE('',*,*,#4549,.F.);
#5997=ORIENTED_EDGE('',*,*,#4558,.T.);
#5998=ORIENTED_EDGE('',*,*,#4559,.T.);
#5999=ORIENTED_EDGE('',*,*,#4560,.T.);
#6000=ORIENTED_EDGE('',*,*,#4556,.F.);
#6001=ORIENTED_EDGE('',*,*,#4561,.T.);
#6002=ORIENTED_EDGE('',*,*,#4562,.T.);
#6003=ORIENTED_EDGE('',*,*,#4563,.T.);
#6004=ORIENTED_EDGE('',*,*,#4559,.F.);
#6005=ORIENTED_EDGE('',*,*,#4564,.T.);
#6006=ORIENTED_EDGE('',*,*,#4565,.T.);
#6007=ORIENTED_EDGE('',*,*,#4566,.T.);
#6008=ORIENTED_EDGE('',*,*,#4562,.F.);
#6009=ORIENTED_EDGE('',*,*,#4567,.T.);
#6010=ORIENTED_EDGE('',*,*,#4568,.T.);
#6011=ORIENTED_EDGE('',*,*,#4569,.T.);
#6012=ORIENTED_EDGE('',*,*,#4565,.F.);
#6013=ORIENTED_EDGE('',*,*,#4570,.T.);
#6014=ORIENTED_EDGE('',*,*,#4571,.T.);
#6015=ORIENTED_EDGE('',*,*,#4572,.T.);
#6016=ORIENTED_EDGE('',*,*,#4568,.F.);
#6017=ORIENTED_EDGE('',*,*,#4573,.T.);
#6018=ORIENTED_EDGE('',*,*,#4574,.T.);
#6019=ORIENTED_EDGE('',*,*,#4575,.T.);
#6020=ORIENTED_EDGE('',*,*,#4571,.F.);
#6021=ORIENTED_EDGE('',*,*,#4576,.T.);
#6022=ORIENTED_EDGE('',*,*,#4577,.T.);
#6023=ORIENTED_EDGE('',*,*,#4578,.T.);
#6024=ORIENTED_EDGE('',*,*,#4574,.F.);
#6025=ORIENTED_EDGE('',*,*,#4579,.T.);
#6026=ORIENTED_EDGE('',*,*,#4580,.T.);
#6027=ORIENTED_EDGE('',*,*,#4581,.T.);
#6028=ORIENTED_EDGE('',*,*,#4577,.F.);
#6029=ORIENTED_EDGE('',*,*,#4582,.T.);
#6030=ORIENTED_EDGE('',*,*,#4583,.T.);
#6031=ORIENTED_EDGE('',*,*,#4584,.T.);
#6032=ORIENTED_EDGE('',*,*,#4580,.F.);
#6033=ORIENTED_EDGE('',*,*,#4585,.T.);
#6034=ORIENTED_EDGE('',*,*,#4586,.F.);
#6035=ORIENTED_EDGE('',*,*,#4587,.T.);
#6036=ORIENTED_EDGE('',*,*,#4588,.F.);
#6037=ORIENTED_EDGE('',*,*,#4589,.T.);
#6038=ORIENTED_EDGE('',*,*,#4590,.T.);
#6039=ORIENTED_EDGE('',*,*,#4591,.T.);
#6040=ORIENTED_EDGE('',*,*,#4592,.F.);
#6041=ORIENTED_EDGE('',*,*,#4593,.F.);
#6042=ORIENTED_EDGE('',*,*,#4594,.T.);
#6043=ORIENTED_EDGE('',*,*,#4595,.T.);
#6044=ORIENTED_EDGE('',*,*,#4590,.F.);
#6045=ORIENTED_EDGE('',*,*,#4596,.F.);
#6046=ORIENTED_EDGE('',*,*,#4597,.T.);
#6047=ORIENTED_EDGE('',*,*,#4598,.T.);
#6048=ORIENTED_EDGE('',*,*,#4594,.F.);
#6049=ORIENTED_EDGE('',*,*,#4599,.F.);
#6050=ORIENTED_EDGE('',*,*,#4600,.T.);
#6051=ORIENTED_EDGE('',*,*,#4601,.T.);
#6052=ORIENTED_EDGE('',*,*,#4597,.F.);
#6053=ORIENTED_EDGE('',*,*,#4602,.F.);
#6054=ORIENTED_EDGE('',*,*,#4603,.T.);
#6055=ORIENTED_EDGE('',*,*,#4604,.T.);
#6056=ORIENTED_EDGE('',*,*,#4600,.F.);
#6057=ORIENTED_EDGE('',*,*,#4605,.F.);
#6058=ORIENTED_EDGE('',*,*,#4606,.T.);
#6059=ORIENTED_EDGE('',*,*,#4607,.T.);
#6060=ORIENTED_EDGE('',*,*,#4603,.F.);
#6061=ORIENTED_EDGE('',*,*,#4608,.F.);
#6062=ORIENTED_EDGE('',*,*,#4609,.T.);
#6063=ORIENTED_EDGE('',*,*,#4610,.T.);
#6064=ORIENTED_EDGE('',*,*,#4606,.F.);
#6065=ORIENTED_EDGE('',*,*,#4611,.F.);
#6066=ORIENTED_EDGE('',*,*,#4612,.T.);
#6067=ORIENTED_EDGE('',*,*,#4613,.T.);
#6068=ORIENTED_EDGE('',*,*,#4609,.F.);
#6069=ORIENTED_EDGE('',*,*,#4614,.F.);
#6070=ORIENTED_EDGE('',*,*,#4615,.T.);
#6071=ORIENTED_EDGE('',*,*,#4616,.T.);
#6072=ORIENTED_EDGE('',*,*,#4612,.F.);
#6073=ORIENTED_EDGE('',*,*,#4617,.F.);
#6074=ORIENTED_EDGE('',*,*,#4618,.T.);
#6075=ORIENTED_EDGE('',*,*,#4619,.T.);
#6076=ORIENTED_EDGE('',*,*,#4615,.F.);
#6077=ORIENTED_EDGE('',*,*,#4620,.F.);
#6078=ORIENTED_EDGE('',*,*,#4621,.T.);
#6079=ORIENTED_EDGE('',*,*,#4622,.T.);
#6080=ORIENTED_EDGE('',*,*,#4618,.F.);
#6081=ORIENTED_EDGE('',*,*,#4623,.F.);
#6082=ORIENTED_EDGE('',*,*,#4624,.T.);
#6083=ORIENTED_EDGE('',*,*,#4625,.T.);
#6084=ORIENTED_EDGE('',*,*,#4621,.F.);
#6085=ORIENTED_EDGE('',*,*,#4626,.F.);
#6086=ORIENTED_EDGE('',*,*,#4627,.F.);
#6087=ORIENTED_EDGE('',*,*,#4628,.F.);
#6088=ORIENTED_EDGE('',*,*,#4629,.F.);
#6089=ORIENTED_EDGE('',*,*,#4630,.T.);
#6090=ORIENTED_EDGE('',*,*,#4631,.T.);
#6091=ORIENTED_EDGE('',*,*,#4632,.T.);
#6092=ORIENTED_EDGE('',*,*,#4633,.T.);
#6093=ORIENTED_EDGE('',*,*,#4634,.T.);
#6094=ORIENTED_EDGE('',*,*,#4635,.T.);
#6095=ORIENTED_EDGE('',*,*,#4636,.T.);
#6096=ORIENTED_EDGE('',*,*,#4635,.F.);
#6097=ORIENTED_EDGE('',*,*,#4637,.T.);
#6098=ORIENTED_EDGE('',*,*,#4638,.T.);
#6099=ORIENTED_EDGE('',*,*,#4639,.T.);
#6100=ORIENTED_EDGE('',*,*,#4631,.F.);
#6101=ORIENTED_EDGE('',*,*,#4640,.T.);
#6102=ORIENTED_EDGE('',*,*,#4641,.T.);
#6103=ORIENTED_EDGE('',*,*,#4642,.T.);
#6104=ORIENTED_EDGE('',*,*,#4638,.F.);
#6105=ORIENTED_EDGE('',*,*,#4643,.T.);
#6106=ORIENTED_EDGE('',*,*,#4644,.T.);
#6107=ORIENTED_EDGE('',*,*,#4645,.T.);
#6108=ORIENTED_EDGE('',*,*,#4641,.F.);
#6109=ORIENTED_EDGE('',*,*,#4646,.T.);
#6110=ORIENTED_EDGE('',*,*,#4647,.T.);
#6111=ORIENTED_EDGE('',*,*,#4648,.T.);
#6112=ORIENTED_EDGE('',*,*,#4644,.F.);
#6113=ORIENTED_EDGE('',*,*,#4649,.T.);
#6114=ORIENTED_EDGE('',*,*,#4650,.T.);
#6115=ORIENTED_EDGE('',*,*,#4651,.T.);
#6116=ORIENTED_EDGE('',*,*,#4647,.F.);
#6117=ORIENTED_EDGE('',*,*,#4652,.T.);
#6118=ORIENTED_EDGE('',*,*,#4653,.T.);
#6119=ORIENTED_EDGE('',*,*,#4654,.T.);
#6120=ORIENTED_EDGE('',*,*,#4650,.F.);
#6121=ORIENTED_EDGE('',*,*,#4655,.T.);
#6122=ORIENTED_EDGE('',*,*,#4656,.T.);
#6123=ORIENTED_EDGE('',*,*,#4657,.T.);
#6124=ORIENTED_EDGE('',*,*,#4653,.F.);
#6125=ORIENTED_EDGE('',*,*,#4658,.T.);
#6126=ORIENTED_EDGE('',*,*,#4659,.T.);
#6127=ORIENTED_EDGE('',*,*,#4660,.T.);
#6128=ORIENTED_EDGE('',*,*,#4656,.F.);
#6129=ORIENTED_EDGE('',*,*,#4661,.T.);
#6130=ORIENTED_EDGE('',*,*,#4662,.T.);
#6131=ORIENTED_EDGE('',*,*,#4663,.T.);
#6132=ORIENTED_EDGE('',*,*,#4659,.F.);
#6133=ORIENTED_EDGE('',*,*,#4664,.T.);
#6134=ORIENTED_EDGE('',*,*,#4665,.T.);
#6135=ORIENTED_EDGE('',*,*,#4666,.T.);
#6136=ORIENTED_EDGE('',*,*,#4662,.F.);
#6137=ORIENTED_EDGE('',*,*,#4667,.T.);
#6138=ORIENTED_EDGE('',*,*,#4668,.F.);
#6139=ORIENTED_EDGE('',*,*,#4669,.T.);
#6140=ORIENTED_EDGE('',*,*,#4670,.F.);
#6141=ORIENTED_EDGE('',*,*,#4671,.T.);
#6142=ORIENTED_EDGE('',*,*,#4672,.T.);
#6143=ORIENTED_EDGE('',*,*,#4673,.T.);
#6144=ORIENTED_EDGE('',*,*,#4674,.F.);
#6145=ORIENTED_EDGE('',*,*,#4675,.F.);
#6146=ORIENTED_EDGE('',*,*,#4676,.T.);
#6147=ORIENTED_EDGE('',*,*,#4677,.T.);
#6148=ORIENTED_EDGE('',*,*,#4672,.F.);
#6149=ORIENTED_EDGE('',*,*,#4678,.F.);
#6150=ORIENTED_EDGE('',*,*,#4679,.T.);
#6151=ORIENTED_EDGE('',*,*,#4680,.T.);
#6152=ORIENTED_EDGE('',*,*,#4676,.F.);
#6153=ORIENTED_EDGE('',*,*,#4681,.F.);
#6154=ORIENTED_EDGE('',*,*,#4682,.T.);
#6155=ORIENTED_EDGE('',*,*,#4683,.T.);
#6156=ORIENTED_EDGE('',*,*,#4679,.F.);
#6157=ORIENTED_EDGE('',*,*,#4684,.F.);
#6158=ORIENTED_EDGE('',*,*,#4685,.T.);
#6159=ORIENTED_EDGE('',*,*,#4686,.T.);
#6160=ORIENTED_EDGE('',*,*,#4682,.F.);
#6161=ORIENTED_EDGE('',*,*,#4687,.F.);
#6162=ORIENTED_EDGE('',*,*,#4688,.T.);
#6163=ORIENTED_EDGE('',*,*,#4689,.T.);
#6164=ORIENTED_EDGE('',*,*,#4685,.F.);
#6165=ORIENTED_EDGE('',*,*,#4690,.F.);
#6166=ORIENTED_EDGE('',*,*,#4691,.T.);
#6167=ORIENTED_EDGE('',*,*,#4692,.T.);
#6168=ORIENTED_EDGE('',*,*,#4688,.F.);
#6169=ORIENTED_EDGE('',*,*,#4693,.F.);
#6170=ORIENTED_EDGE('',*,*,#4694,.T.);
#6171=ORIENTED_EDGE('',*,*,#4695,.T.);
#6172=ORIENTED_EDGE('',*,*,#4691,.F.);
#6173=ORIENTED_EDGE('',*,*,#4696,.F.);
#6174=ORIENTED_EDGE('',*,*,#4697,.T.);
#6175=ORIENTED_EDGE('',*,*,#4698,.T.);
#6176=ORIENTED_EDGE('',*,*,#4694,.F.);
#6177=ORIENTED_EDGE('',*,*,#4699,.F.);
#6178=ORIENTED_EDGE('',*,*,#4700,.T.);
#6179=ORIENTED_EDGE('',*,*,#4701,.T.);
#6180=ORIENTED_EDGE('',*,*,#4697,.F.);
#6181=ORIENTED_EDGE('',*,*,#4702,.F.);
#6182=ORIENTED_EDGE('',*,*,#4703,.T.);
#6183=ORIENTED_EDGE('',*,*,#4704,.T.);
#6184=ORIENTED_EDGE('',*,*,#4700,.F.);
#6185=ORIENTED_EDGE('',*,*,#4705,.F.);
#6186=ORIENTED_EDGE('',*,*,#4706,.T.);
#6187=ORIENTED_EDGE('',*,*,#4707,.T.);
#6188=ORIENTED_EDGE('',*,*,#4703,.F.);
#6189=ORIENTED_EDGE('',*,*,#4708,.F.);
#6190=ORIENTED_EDGE('',*,*,#4709,.F.);
#6191=ORIENTED_EDGE('',*,*,#4710,.F.);
#6192=ORIENTED_EDGE('',*,*,#4711,.F.);
#6193=ORIENTED_EDGE('',*,*,#4712,.T.);
#6194=ORIENTED_EDGE('',*,*,#4713,.T.);
#6195=ORIENTED_EDGE('',*,*,#4714,.T.);
#6196=ORIENTED_EDGE('',*,*,#4715,.T.);
#6197=ORIENTED_EDGE('',*,*,#4716,.T.);
#6198=ORIENTED_EDGE('',*,*,#4717,.T.);
#6199=ORIENTED_EDGE('',*,*,#4718,.T.);
#6200=ORIENTED_EDGE('',*,*,#4717,.F.);
#6201=ORIENTED_EDGE('',*,*,#4719,.T.);
#6202=ORIENTED_EDGE('',*,*,#4720,.T.);
#6203=ORIENTED_EDGE('',*,*,#4721,.T.);
#6204=ORIENTED_EDGE('',*,*,#4713,.F.);
#6205=ORIENTED_EDGE('',*,*,#4722,.T.);
#6206=ORIENTED_EDGE('',*,*,#4723,.T.);
#6207=ORIENTED_EDGE('',*,*,#4724,.T.);
#6208=ORIENTED_EDGE('',*,*,#4720,.F.);
#6209=ORIENTED_EDGE('',*,*,#4725,.T.);
#6210=ORIENTED_EDGE('',*,*,#4726,.T.);
#6211=ORIENTED_EDGE('',*,*,#4727,.T.);
#6212=ORIENTED_EDGE('',*,*,#4723,.F.);
#6213=ORIENTED_EDGE('',*,*,#4728,.T.);
#6214=ORIENTED_EDGE('',*,*,#4729,.T.);
#6215=ORIENTED_EDGE('',*,*,#4730,.T.);
#6216=ORIENTED_EDGE('',*,*,#4726,.F.);
#6217=ORIENTED_EDGE('',*,*,#4731,.T.);
#6218=ORIENTED_EDGE('',*,*,#4732,.T.);
#6219=ORIENTED_EDGE('',*,*,#4733,.T.);
#6220=ORIENTED_EDGE('',*,*,#4729,.F.);
#6221=ORIENTED_EDGE('',*,*,#4734,.T.);
#6222=ORIENTED_EDGE('',*,*,#4735,.T.);
#6223=ORIENTED_EDGE('',*,*,#4736,.T.);
#6224=ORIENTED_EDGE('',*,*,#4732,.F.);
#6225=ORIENTED_EDGE('',*,*,#4737,.T.);
#6226=ORIENTED_EDGE('',*,*,#4738,.T.);
#6227=ORIENTED_EDGE('',*,*,#4739,.T.);
#6228=ORIENTED_EDGE('',*,*,#4735,.F.);
#6229=ORIENTED_EDGE('',*,*,#4740,.T.);
#6230=ORIENTED_EDGE('',*,*,#4741,.T.);
#6231=ORIENTED_EDGE('',*,*,#4742,.T.);
#6232=ORIENTED_EDGE('',*,*,#4738,.F.);
#6233=ORIENTED_EDGE('',*,*,#4743,.T.);
#6234=ORIENTED_EDGE('',*,*,#4744,.T.);
#6235=ORIENTED_EDGE('',*,*,#4745,.T.);
#6236=ORIENTED_EDGE('',*,*,#4741,.F.);
#6237=ORIENTED_EDGE('',*,*,#4746,.T.);
#6238=ORIENTED_EDGE('',*,*,#4747,.T.);
#6239=ORIENTED_EDGE('',*,*,#4748,.T.);
#6240=ORIENTED_EDGE('',*,*,#4744,.F.);
#6241=ORIENTED_EDGE('',*,*,#4749,.T.);
#6242=ORIENTED_EDGE('',*,*,#4750,.F.);
#6243=ORIENTED_EDGE('',*,*,#4751,.T.);
#6244=ORIENTED_EDGE('',*,*,#4752,.F.);
#6245=ORIENTED_EDGE('',*,*,#4753,.T.);
#6246=ORIENTED_EDGE('',*,*,#4754,.T.);
#6247=ORIENTED_EDGE('',*,*,#4755,.T.);
#6248=ORIENTED_EDGE('',*,*,#4756,.F.);
#6249=ORIENTED_EDGE('',*,*,#4757,.F.);
#6250=ORIENTED_EDGE('',*,*,#4758,.T.);
#6251=ORIENTED_EDGE('',*,*,#4759,.T.);
#6252=ORIENTED_EDGE('',*,*,#4754,.F.);
#6253=ORIENTED_EDGE('',*,*,#4760,.F.);
#6254=ORIENTED_EDGE('',*,*,#4761,.T.);
#6255=ORIENTED_EDGE('',*,*,#4762,.T.);
#6256=ORIENTED_EDGE('',*,*,#4758,.F.);
#6257=ORIENTED_EDGE('',*,*,#4763,.F.);
#6258=ORIENTED_EDGE('',*,*,#4764,.T.);
#6259=ORIENTED_EDGE('',*,*,#4765,.T.);
#6260=ORIENTED_EDGE('',*,*,#4761,.F.);
#6261=ORIENTED_EDGE('',*,*,#4766,.F.);
#6262=ORIENTED_EDGE('',*,*,#4767,.T.);
#6263=ORIENTED_EDGE('',*,*,#4768,.T.);
#6264=ORIENTED_EDGE('',*,*,#4764,.F.);
#6265=ORIENTED_EDGE('',*,*,#4769,.F.);
#6266=ORIENTED_EDGE('',*,*,#4770,.T.);
#6267=ORIENTED_EDGE('',*,*,#4771,.T.);
#6268=ORIENTED_EDGE('',*,*,#4767,.F.);
#6269=ORIENTED_EDGE('',*,*,#4772,.F.);
#6270=ORIENTED_EDGE('',*,*,#4773,.T.);
#6271=ORIENTED_EDGE('',*,*,#4774,.T.);
#6272=ORIENTED_EDGE('',*,*,#4770,.F.);
#6273=ORIENTED_EDGE('',*,*,#4775,.F.);
#6274=ORIENTED_EDGE('',*,*,#4776,.T.);
#6275=ORIENTED_EDGE('',*,*,#4777,.T.);
#6276=ORIENTED_EDGE('',*,*,#4773,.F.);
#6277=ORIENTED_EDGE('',*,*,#4778,.F.);
#6278=ORIENTED_EDGE('',*,*,#4779,.T.);
#6279=ORIENTED_EDGE('',*,*,#4780,.T.);
#6280=ORIENTED_EDGE('',*,*,#4776,.F.);
#6281=ORIENTED_EDGE('',*,*,#4781,.F.);
#6282=ORIENTED_EDGE('',*,*,#4782,.T.);
#6283=ORIENTED_EDGE('',*,*,#4783,.T.);
#6284=ORIENTED_EDGE('',*,*,#4779,.F.);
#6285=ORIENTED_EDGE('',*,*,#4784,.F.);
#6286=ORIENTED_EDGE('',*,*,#4785,.T.);
#6287=ORIENTED_EDGE('',*,*,#4786,.T.);
#6288=ORIENTED_EDGE('',*,*,#4782,.F.);
#6289=ORIENTED_EDGE('',*,*,#4787,.F.);
#6290=ORIENTED_EDGE('',*,*,#4788,.T.);
#6291=ORIENTED_EDGE('',*,*,#4789,.T.);
#6292=ORIENTED_EDGE('',*,*,#4785,.F.);
#6293=ORIENTED_EDGE('',*,*,#4790,.F.);
#6294=ORIENTED_EDGE('',*,*,#4791,.F.);
#6295=ORIENTED_EDGE('',*,*,#4792,.F.);
#6296=ORIENTED_EDGE('',*,*,#4793,.F.);
#6297=ORIENTED_EDGE('',*,*,#4794,.T.);
#6298=ORIENTED_EDGE('',*,*,#4795,.T.);
#6299=ORIENTED_EDGE('',*,*,#4796,.T.);
#6300=ORIENTED_EDGE('',*,*,#4797,.T.);
#6301=ORIENTED_EDGE('',*,*,#4798,.T.);
#6302=ORIENTED_EDGE('',*,*,#4799,.T.);
#6303=ORIENTED_EDGE('',*,*,#4800,.T.);
#6304=ORIENTED_EDGE('',*,*,#4799,.F.);
#6305=ORIENTED_EDGE('',*,*,#4801,.T.);
#6306=ORIENTED_EDGE('',*,*,#4802,.T.);
#6307=ORIENTED_EDGE('',*,*,#4803,.T.);
#6308=ORIENTED_EDGE('',*,*,#4795,.F.);
#6309=ORIENTED_EDGE('',*,*,#4804,.T.);
#6310=ORIENTED_EDGE('',*,*,#4805,.T.);
#6311=ORIENTED_EDGE('',*,*,#4806,.T.);
#6312=ORIENTED_EDGE('',*,*,#4802,.F.);
#6313=ORIENTED_EDGE('',*,*,#4807,.T.);
#6314=ORIENTED_EDGE('',*,*,#4808,.T.);
#6315=ORIENTED_EDGE('',*,*,#4809,.T.);
#6316=ORIENTED_EDGE('',*,*,#4805,.F.);
#6317=ORIENTED_EDGE('',*,*,#4810,.T.);
#6318=ORIENTED_EDGE('',*,*,#4811,.T.);
#6319=ORIENTED_EDGE('',*,*,#4812,.T.);
#6320=ORIENTED_EDGE('',*,*,#4808,.F.);
#6321=ORIENTED_EDGE('',*,*,#4813,.T.);
#6322=ORIENTED_EDGE('',*,*,#4814,.T.);
#6323=ORIENTED_EDGE('',*,*,#4815,.T.);
#6324=ORIENTED_EDGE('',*,*,#4811,.F.);
#6325=ORIENTED_EDGE('',*,*,#4816,.T.);
#6326=ORIENTED_EDGE('',*,*,#4817,.T.);
#6327=ORIENTED_EDGE('',*,*,#4818,.T.);
#6328=ORIENTED_EDGE('',*,*,#4814,.F.);
#6329=ORIENTED_EDGE('',*,*,#4819,.T.);
#6330=ORIENTED_EDGE('',*,*,#4820,.T.);
#6331=ORIENTED_EDGE('',*,*,#4821,.T.);
#6332=ORIENTED_EDGE('',*,*,#4817,.F.);
#6333=ORIENTED_EDGE('',*,*,#4822,.T.);
#6334=ORIENTED_EDGE('',*,*,#4823,.T.);
#6335=ORIENTED_EDGE('',*,*,#4824,.T.);
#6336=ORIENTED_EDGE('',*,*,#4820,.F.);
#6337=ORIENTED_EDGE('',*,*,#4825,.T.);
#6338=ORIENTED_EDGE('',*,*,#4826,.T.);
#6339=ORIENTED_EDGE('',*,*,#4827,.T.);
#6340=ORIENTED_EDGE('',*,*,#4823,.F.);
#6341=ORIENTED_EDGE('',*,*,#4828,.T.);
#6342=ORIENTED_EDGE('',*,*,#4829,.T.);
#6343=ORIENTED_EDGE('',*,*,#4830,.T.);
#6344=ORIENTED_EDGE('',*,*,#4826,.F.);
#6345=ORIENTED_EDGE('',*,*,#4831,.T.);
#6346=ORIENTED_EDGE('',*,*,#4832,.F.);
#6347=ORIENTED_EDGE('',*,*,#4833,.T.);
#6348=ORIENTED_EDGE('',*,*,#4834,.F.);
#6349=ORIENTED_EDGE('',*,*,#4835,.T.);
#6350=ORIENTED_EDGE('',*,*,#4836,.T.);
#6351=ORIENTED_EDGE('',*,*,#4837,.T.);
#6352=ORIENTED_EDGE('',*,*,#4838,.F.);
#6353=ORIENTED_EDGE('',*,*,#4839,.F.);
#6354=ORIENTED_EDGE('',*,*,#4840,.T.);
#6355=ORIENTED_EDGE('',*,*,#4841,.T.);
#6356=ORIENTED_EDGE('',*,*,#4836,.F.);
#6357=ORIENTED_EDGE('',*,*,#4842,.F.);
#6358=ORIENTED_EDGE('',*,*,#4843,.T.);
#6359=ORIENTED_EDGE('',*,*,#4844,.T.);
#6360=ORIENTED_EDGE('',*,*,#4840,.F.);
#6361=ORIENTED_EDGE('',*,*,#4845,.F.);
#6362=ORIENTED_EDGE('',*,*,#4846,.T.);
#6363=ORIENTED_EDGE('',*,*,#4847,.T.);
#6364=ORIENTED_EDGE('',*,*,#4843,.F.);
#6365=ORIENTED_EDGE('',*,*,#4848,.F.);
#6366=ORIENTED_EDGE('',*,*,#4849,.T.);
#6367=ORIENTED_EDGE('',*,*,#4850,.T.);
#6368=ORIENTED_EDGE('',*,*,#4846,.F.);
#6369=ORIENTED_EDGE('',*,*,#4851,.F.);
#6370=ORIENTED_EDGE('',*,*,#4852,.T.);
#6371=ORIENTED_EDGE('',*,*,#4853,.T.);
#6372=ORIENTED_EDGE('',*,*,#4849,.F.);
#6373=ORIENTED_EDGE('',*,*,#4854,.F.);
#6374=ORIENTED_EDGE('',*,*,#4855,.T.);
#6375=ORIENTED_EDGE('',*,*,#4856,.T.);
#6376=ORIENTED_EDGE('',*,*,#4852,.F.);
#6377=ORIENTED_EDGE('',*,*,#4857,.F.);
#6378=ORIENTED_EDGE('',*,*,#4858,.T.);
#6379=ORIENTED_EDGE('',*,*,#4859,.T.);
#6380=ORIENTED_EDGE('',*,*,#4855,.F.);
#6381=ORIENTED_EDGE('',*,*,#4860,.F.);
#6382=ORIENTED_EDGE('',*,*,#4861,.T.);
#6383=ORIENTED_EDGE('',*,*,#4862,.T.);
#6384=ORIENTED_EDGE('',*,*,#4858,.F.);
#6385=ORIENTED_EDGE('',*,*,#4863,.F.);
#6386=ORIENTED_EDGE('',*,*,#4864,.T.);
#6387=ORIENTED_EDGE('',*,*,#4865,.T.);
#6388=ORIENTED_EDGE('',*,*,#4861,.F.);
#6389=ORIENTED_EDGE('',*,*,#4866,.F.);
#6390=ORIENTED_EDGE('',*,*,#4867,.T.);
#6391=ORIENTED_EDGE('',*,*,#4868,.T.);
#6392=ORIENTED_EDGE('',*,*,#4864,.F.);
#6393=ORIENTED_EDGE('',*,*,#4869,.F.);
#6394=ORIENTED_EDGE('',*,*,#4870,.T.);
#6395=ORIENTED_EDGE('',*,*,#4871,.T.);
#6396=ORIENTED_EDGE('',*,*,#4867,.F.);
#6397=ORIENTED_EDGE('',*,*,#4872,.F.);
#6398=ORIENTED_EDGE('',*,*,#4873,.F.);
#6399=ORIENTED_EDGE('',*,*,#4874,.F.);
#6400=ORIENTED_EDGE('',*,*,#4875,.F.);
#6401=ORIENTED_EDGE('',*,*,#4876,.T.);
#6402=ORIENTED_EDGE('',*,*,#4877,.F.);
#6403=ORIENTED_EDGE('',*,*,#4878,.T.);
#6404=ORIENTED_EDGE('',*,*,#4879,.T.);
#6405=ORIENTED_EDGE('',*,*,#4880,.T.);
#6406=ORIENTED_EDGE('',*,*,#4878,.F.);
#6407=ORIENTED_EDGE('',*,*,#4881,.T.);
#6408=ORIENTED_EDGE('',*,*,#4882,.F.);
#6409=ORIENTED_EDGE('',*,*,#4883,.F.);
#6410=ORIENTED_EDGE('',*,*,#4884,.F.);
#6411=ORIENTED_EDGE('',*,*,#4885,.T.);
#6412=ORIENTED_EDGE('',*,*,#4886,.T.);
#6413=ORIENTED_EDGE('',*,*,#4882,.T.);
#6414=ORIENTED_EDGE('',*,*,#4885,.F.);
#6415=ORIENTED_EDGE('',*,*,#4887,.T.);
#6416=ORIENTED_EDGE('',*,*,#4888,.F.);
#6417=ORIENTED_EDGE('',*,*,#4889,.F.);
#6418=ORIENTED_EDGE('',*,*,#4890,.F.);
#6419=ORIENTED_EDGE('',*,*,#4891,.T.);
#6420=ORIENTED_EDGE('',*,*,#4892,.T.);
#6421=ORIENTED_EDGE('',*,*,#4893,.T.);
#6422=ORIENTED_EDGE('',*,*,#4877,.T.);
#6423=ORIENTED_EDGE('',*,*,#4894,.F.);
#6424=ORIENTED_EDGE('',*,*,#4890,.T.);
#6425=ORIENTED_EDGE('',*,*,#4895,.F.);
#6426=ORIENTED_EDGE('',*,*,#4896,.T.);
#6427=ORIENTED_EDGE('',*,*,#4887,.F.);
#6428=ORIENTED_EDGE('',*,*,#4884,.T.);
#6429=ORIENTED_EDGE('',*,*,#4881,.F.);
#6430=ORIENTED_EDGE('',*,*,#4897,.T.);
#6431=ORIENTED_EDGE('',*,*,#4898,.T.);
#6432=ORIENTED_EDGE('',*,*,#4899,.T.);
#6433=ORIENTED_EDGE('',*,*,#4893,.F.);
#6434=ORIENTED_EDGE('',*,*,#4900,.F.);
#6435=ORIENTED_EDGE('',*,*,#4901,.F.);
#6436=ORIENTED_EDGE('',*,*,#4895,.T.);
#6437=ORIENTED_EDGE('',*,*,#4902,.T.);
#6438=ORIENTED_EDGE('',*,*,#4896,.F.);
#6439=ORIENTED_EDGE('',*,*,#4901,.T.);
#6440=ORIENTED_EDGE('',*,*,#4903,.T.);
#6441=ORIENTED_EDGE('',*,*,#4888,.T.);
#6442=ORIENTED_EDGE('',*,*,#4904,.F.);
#6443=ORIENTED_EDGE('',*,*,#4905,.T.);
#6444=ORIENTED_EDGE('',*,*,#4902,.F.);
#6445=ORIENTED_EDGE('',*,*,#4905,.F.);
#6446=ORIENTED_EDGE('',*,*,#4906,.F.);
#6447=ORIENTED_EDGE('',*,*,#4907,.T.);
#6448=ORIENTED_EDGE('',*,*,#4908,.F.);
#6449=ORIENTED_EDGE('',*,*,#4909,.T.);
#6450=ORIENTED_EDGE('',*,*,#4906,.T.);
#6451=ORIENTED_EDGE('',*,*,#4909,.F.);
#6452=ORIENTED_EDGE('',*,*,#4907,.F.);
#6453=ORIENTED_EDGE('',*,*,#4910,.T.);
#6454=ORIENTED_EDGE('',*,*,#4899,.F.);
#6455=ORIENTED_EDGE('',*,*,#4910,.F.);
#6456=ORIENTED_EDGE('',*,*,#4911,.F.);
#6457=ORIENTED_EDGE('',*,*,#4912,.T.);
#6458=ORIENTED_EDGE('',*,*,#4913,.F.);
#6459=ORIENTED_EDGE('',*,*,#4914,.T.);
#6460=ORIENTED_EDGE('',*,*,#4911,.T.);
#6461=ORIENTED_EDGE('',*,*,#4914,.F.);
#6462=ORIENTED_EDGE('',*,*,#4912,.F.);
#6463=ORIENTED_EDGE('',*,*,#4915,.T.);
#6464=ORIENTED_EDGE('',*,*,#4898,.F.);
#6465=ORIENTED_EDGE('',*,*,#4915,.F.);
#6466=ORIENTED_EDGE('',*,*,#4797,.F.);
#6467=ORIENTED_EDGE('',*,*,#4916,.T.);
#6468=ORIENTED_EDGE('',*,*,#4838,.T.);
#6469=ORIENTED_EDGE('',*,*,#4917,.T.);
#6470=ORIENTED_EDGE('',*,*,#4873,.T.);
#6471=ORIENTED_EDGE('',*,*,#4918,.T.);
#6472=ORIENTED_EDGE('',*,*,#4870,.F.);
#6473=ORIENTED_EDGE('',*,*,#4919,.F.);
#6474=ORIENTED_EDGE('',*,*,#4917,.F.);
#6475=ORIENTED_EDGE('',*,*,#4837,.F.);
#6476=ORIENTED_EDGE('',*,*,#4841,.F.);
#6477=ORIENTED_EDGE('',*,*,#4844,.F.);
#6478=ORIENTED_EDGE('',*,*,#4847,.F.);
#6479=ORIENTED_EDGE('',*,*,#4850,.F.);
#6480=ORIENTED_EDGE('',*,*,#4853,.F.);
#6481=ORIENTED_EDGE('',*,*,#4856,.F.);
#6482=ORIENTED_EDGE('',*,*,#4859,.F.);
#6483=ORIENTED_EDGE('',*,*,#4862,.F.);
#6484=ORIENTED_EDGE('',*,*,#4865,.F.);
#6485=ORIENTED_EDGE('',*,*,#4868,.F.);
#6486=ORIENTED_EDGE('',*,*,#4871,.F.);
#6487=ORIENTED_EDGE('',*,*,#4918,.F.);
#6488=ORIENTED_EDGE('',*,*,#4876,.F.);
#6489=ORIENTED_EDGE('',*,*,#4920,.F.);
#6490=ORIENTED_EDGE('',*,*,#4833,.F.);
#6491=ORIENTED_EDGE('',*,*,#4921,.F.);
#6492=ORIENTED_EDGE('',*,*,#4831,.F.);
#6493=ORIENTED_EDGE('',*,*,#4828,.F.);
#6494=ORIENTED_EDGE('',*,*,#4825,.F.);
#6495=ORIENTED_EDGE('',*,*,#4822,.F.);
#6496=ORIENTED_EDGE('',*,*,#4819,.F.);
#6497=ORIENTED_EDGE('',*,*,#4816,.F.);
#6498=ORIENTED_EDGE('',*,*,#4813,.F.);
#6499=ORIENTED_EDGE('',*,*,#4810,.F.);
#6500=ORIENTED_EDGE('',*,*,#4807,.F.);
#6501=ORIENTED_EDGE('',*,*,#4804,.F.);
#6502=ORIENTED_EDGE('',*,*,#4801,.F.);
#6503=ORIENTED_EDGE('',*,*,#4798,.F.);
#6504=ORIENTED_EDGE('',*,*,#4916,.F.);
#6505=ORIENTED_EDGE('',*,*,#4796,.F.);
#6506=ORIENTED_EDGE('',*,*,#4803,.F.);
#6507=ORIENTED_EDGE('',*,*,#4806,.F.);
#6508=ORIENTED_EDGE('',*,*,#4809,.F.);
#6509=ORIENTED_EDGE('',*,*,#4812,.F.);
#6510=ORIENTED_EDGE('',*,*,#4815,.F.);
#6511=ORIENTED_EDGE('',*,*,#4818,.F.);
#6512=ORIENTED_EDGE('',*,*,#4821,.F.);
#6513=ORIENTED_EDGE('',*,*,#4824,.F.);
#6514=ORIENTED_EDGE('',*,*,#4827,.F.);
#6515=ORIENTED_EDGE('',*,*,#4830,.F.);
#6516=ORIENTED_EDGE('',*,*,#4922,.F.);
#6517=ORIENTED_EDGE('',*,*,#4835,.F.);
#6518=ORIENTED_EDGE('',*,*,#4923,.F.);
#6519=ORIENTED_EDGE('',*,*,#4874,.T.);
#6520=ORIENTED_EDGE('',*,*,#4919,.T.);
#6521=ORIENTED_EDGE('',*,*,#4872,.T.);
#6522=ORIENTED_EDGE('',*,*,#4869,.T.);
#6523=ORIENTED_EDGE('',*,*,#4866,.T.);
#6524=ORIENTED_EDGE('',*,*,#4863,.T.);
#6525=ORIENTED_EDGE('',*,*,#4860,.T.);
#6526=ORIENTED_EDGE('',*,*,#4857,.T.);
#6527=ORIENTED_EDGE('',*,*,#4854,.T.);
#6528=ORIENTED_EDGE('',*,*,#4851,.T.);
#6529=ORIENTED_EDGE('',*,*,#4848,.T.);
#6530=ORIENTED_EDGE('',*,*,#4845,.T.);
#6531=ORIENTED_EDGE('',*,*,#4842,.T.);
#6532=ORIENTED_EDGE('',*,*,#4839,.T.);
#6533=ORIENTED_EDGE('',*,*,#4832,.T.);
#6534=ORIENTED_EDGE('',*,*,#4922,.T.);
#6535=ORIENTED_EDGE('',*,*,#4829,.F.);
#6536=ORIENTED_EDGE('',*,*,#4921,.T.);
#6537=ORIENTED_EDGE('',*,*,#4715,.F.);
#6538=ORIENTED_EDGE('',*,*,#4924,.T.);
#6539=ORIENTED_EDGE('',*,*,#4756,.T.);
#6540=ORIENTED_EDGE('',*,*,#4925,.T.);
#6541=ORIENTED_EDGE('',*,*,#4791,.T.);
#6542=ORIENTED_EDGE('',*,*,#4926,.T.);
#6543=ORIENTED_EDGE('',*,*,#4788,.F.);
#6544=ORIENTED_EDGE('',*,*,#4927,.F.);
#6545=ORIENTED_EDGE('',*,*,#4925,.F.);
#6546=ORIENTED_EDGE('',*,*,#4755,.F.);
#6547=ORIENTED_EDGE('',*,*,#4759,.F.);
#6548=ORIENTED_EDGE('',*,*,#4762,.F.);
#6549=ORIENTED_EDGE('',*,*,#4765,.F.);
#6550=ORIENTED_EDGE('',*,*,#4768,.F.);
#6551=ORIENTED_EDGE('',*,*,#4771,.F.);
#6552=ORIENTED_EDGE('',*,*,#4774,.F.);
#6553=ORIENTED_EDGE('',*,*,#4777,.F.);
#6554=ORIENTED_EDGE('',*,*,#4780,.F.);
#6555=ORIENTED_EDGE('',*,*,#4783,.F.);
#6556=ORIENTED_EDGE('',*,*,#4786,.F.);
#6557=ORIENTED_EDGE('',*,*,#4789,.F.);
#6558=ORIENTED_EDGE('',*,*,#4926,.F.);
#6559=ORIENTED_EDGE('',*,*,#4794,.F.);
#6560=ORIENTED_EDGE('',*,*,#4928,.F.);
#6561=ORIENTED_EDGE('',*,*,#4751,.F.);
#6562=ORIENTED_EDGE('',*,*,#4929,.F.);
#6563=ORIENTED_EDGE('',*,*,#4749,.F.);
#6564=ORIENTED_EDGE('',*,*,#4746,.F.);
#6565=ORIENTED_EDGE('',*,*,#4743,.F.);
#6566=ORIENTED_EDGE('',*,*,#4740,.F.);
#6567=ORIENTED_EDGE('',*,*,#4737,.F.);
#6568=ORIENTED_EDGE('',*,*,#4734,.F.);
#6569=ORIENTED_EDGE('',*,*,#4731,.F.);
#6570=ORIENTED_EDGE('',*,*,#4728,.F.);
#6571=ORIENTED_EDGE('',*,*,#4725,.F.);
#6572=ORIENTED_EDGE('',*,*,#4722,.F.);
#6573=ORIENTED_EDGE('',*,*,#4719,.F.);
#6574=ORIENTED_EDGE('',*,*,#4716,.F.);
#6575=ORIENTED_EDGE('',*,*,#4924,.F.);
#6576=ORIENTED_EDGE('',*,*,#4714,.F.);
#6577=ORIENTED_EDGE('',*,*,#4721,.F.);
#6578=ORIENTED_EDGE('',*,*,#4724,.F.);
#6579=ORIENTED_EDGE('',*,*,#4727,.F.);
#6580=ORIENTED_EDGE('',*,*,#4730,.F.);
#6581=ORIENTED_EDGE('',*,*,#4733,.F.);
#6582=ORIENTED_EDGE('',*,*,#4736,.F.);
#6583=ORIENTED_EDGE('',*,*,#4739,.F.);
#6584=ORIENTED_EDGE('',*,*,#4742,.F.);
#6585=ORIENTED_EDGE('',*,*,#4745,.F.);
#6586=ORIENTED_EDGE('',*,*,#4748,.F.);
#6587=ORIENTED_EDGE('',*,*,#4930,.F.);
#6588=ORIENTED_EDGE('',*,*,#4753,.F.);
#6589=ORIENTED_EDGE('',*,*,#4931,.F.);
#6590=ORIENTED_EDGE('',*,*,#4792,.T.);
#6591=ORIENTED_EDGE('',*,*,#4927,.T.);
#6592=ORIENTED_EDGE('',*,*,#4790,.T.);
#6593=ORIENTED_EDGE('',*,*,#4787,.T.);
#6594=ORIENTED_EDGE('',*,*,#4784,.T.);
#6595=ORIENTED_EDGE('',*,*,#4781,.T.);
#6596=ORIENTED_EDGE('',*,*,#4778,.T.);
#6597=ORIENTED_EDGE('',*,*,#4775,.T.);
#6598=ORIENTED_EDGE('',*,*,#4772,.T.);
#6599=ORIENTED_EDGE('',*,*,#4769,.T.);
#6600=ORIENTED_EDGE('',*,*,#4766,.T.);
#6601=ORIENTED_EDGE('',*,*,#4763,.T.);
#6602=ORIENTED_EDGE('',*,*,#4760,.T.);
#6603=ORIENTED_EDGE('',*,*,#4757,.T.);
#6604=ORIENTED_EDGE('',*,*,#4750,.T.);
#6605=ORIENTED_EDGE('',*,*,#4930,.T.);
#6606=ORIENTED_EDGE('',*,*,#4747,.F.);
#6607=ORIENTED_EDGE('',*,*,#4929,.T.);
#6608=ORIENTED_EDGE('',*,*,#4633,.F.);
#6609=ORIENTED_EDGE('',*,*,#4932,.T.);
#6610=ORIENTED_EDGE('',*,*,#4674,.T.);
#6611=ORIENTED_EDGE('',*,*,#4933,.T.);
#6612=ORIENTED_EDGE('',*,*,#4709,.T.);
#6613=ORIENTED_EDGE('',*,*,#4934,.T.);
#6614=ORIENTED_EDGE('',*,*,#4706,.F.);
#6615=ORIENTED_EDGE('',*,*,#4935,.F.);
#6616=ORIENTED_EDGE('',*,*,#4933,.F.);
#6617=ORIENTED_EDGE('',*,*,#4673,.F.);
#6618=ORIENTED_EDGE('',*,*,#4677,.F.);
#6619=ORIENTED_EDGE('',*,*,#4680,.F.);
#6620=ORIENTED_EDGE('',*,*,#4683,.F.);
#6621=ORIENTED_EDGE('',*,*,#4686,.F.);
#6622=ORIENTED_EDGE('',*,*,#4689,.F.);
#6623=ORIENTED_EDGE('',*,*,#4692,.F.);
#6624=ORIENTED_EDGE('',*,*,#4695,.F.);
#6625=ORIENTED_EDGE('',*,*,#4698,.F.);
#6626=ORIENTED_EDGE('',*,*,#4701,.F.);
#6627=ORIENTED_EDGE('',*,*,#4704,.F.);
#6628=ORIENTED_EDGE('',*,*,#4707,.F.);
#6629=ORIENTED_EDGE('',*,*,#4934,.F.);
#6630=ORIENTED_EDGE('',*,*,#4712,.F.);
#6631=ORIENTED_EDGE('',*,*,#4936,.F.);
#6632=ORIENTED_EDGE('',*,*,#4669,.F.);
#6633=ORIENTED_EDGE('',*,*,#4937,.F.);
#6634=ORIENTED_EDGE('',*,*,#4667,.F.);
#6635=ORIENTED_EDGE('',*,*,#4664,.F.);
#6636=ORIENTED_EDGE('',*,*,#4661,.F.);
#6637=ORIENTED_EDGE('',*,*,#4658,.F.);
#6638=ORIENTED_EDGE('',*,*,#4655,.F.);
#6639=ORIENTED_EDGE('',*,*,#4652,.F.);
#6640=ORIENTED_EDGE('',*,*,#4649,.F.);
#6641=ORIENTED_EDGE('',*,*,#4646,.F.);
#6642=ORIENTED_EDGE('',*,*,#4643,.F.);
#6643=ORIENTED_EDGE('',*,*,#4640,.F.);
#6644=ORIENTED_EDGE('',*,*,#4637,.F.);
#6645=ORIENTED_EDGE('',*,*,#4634,.F.);
#6646=ORIENTED_EDGE('',*,*,#4932,.F.);
#6647=ORIENTED_EDGE('',*,*,#4632,.F.);
#6648=ORIENTED_EDGE('',*,*,#4639,.F.);
#6649=ORIENTED_EDGE('',*,*,#4642,.F.);
#6650=ORIENTED_EDGE('',*,*,#4645,.F.);
#6651=ORIENTED_EDGE('',*,*,#4648,.F.);
#6652=ORIENTED_EDGE('',*,*,#4651,.F.);
#6653=ORIENTED_EDGE('',*,*,#4654,.F.);
#6654=ORIENTED_EDGE('',*,*,#4657,.F.);
#6655=ORIENTED_EDGE('',*,*,#4660,.F.);
#6656=ORIENTED_EDGE('',*,*,#4663,.F.);
#6657=ORIENTED_EDGE('',*,*,#4666,.F.);
#6658=ORIENTED_EDGE('',*,*,#4938,.F.);
#6659=ORIENTED_EDGE('',*,*,#4671,.F.);
#6660=ORIENTED_EDGE('',*,*,#4939,.F.);
#6661=ORIENTED_EDGE('',*,*,#4710,.T.);
#6662=ORIENTED_EDGE('',*,*,#4935,.T.);
#6663=ORIENTED_EDGE('',*,*,#4708,.T.);
#6664=ORIENTED_EDGE('',*,*,#4705,.T.);
#6665=ORIENTED_EDGE('',*,*,#4702,.T.);
#6666=ORIENTED_EDGE('',*,*,#4699,.T.);
#6667=ORIENTED_EDGE('',*,*,#4696,.T.);
#6668=ORIENTED_EDGE('',*,*,#4693,.T.);
#6669=ORIENTED_EDGE('',*,*,#4690,.T.);
#6670=ORIENTED_EDGE('',*,*,#4687,.T.);
#6671=ORIENTED_EDGE('',*,*,#4684,.T.);
#6672=ORIENTED_EDGE('',*,*,#4681,.T.);
#6673=ORIENTED_EDGE('',*,*,#4678,.T.);
#6674=ORIENTED_EDGE('',*,*,#4675,.T.);
#6675=ORIENTED_EDGE('',*,*,#4668,.T.);
#6676=ORIENTED_EDGE('',*,*,#4938,.T.);
#6677=ORIENTED_EDGE('',*,*,#4665,.F.);
#6678=ORIENTED_EDGE('',*,*,#4937,.T.);
#6679=ORIENTED_EDGE('',*,*,#4551,.F.);
#6680=ORIENTED_EDGE('',*,*,#4940,.T.);
#6681=ORIENTED_EDGE('',*,*,#4592,.T.);
#6682=ORIENTED_EDGE('',*,*,#4941,.T.);
#6683=ORIENTED_EDGE('',*,*,#4627,.T.);
#6684=ORIENTED_EDGE('',*,*,#4942,.T.);
#6685=ORIENTED_EDGE('',*,*,#4624,.F.);
#6686=ORIENTED_EDGE('',*,*,#4943,.F.);
#6687=ORIENTED_EDGE('',*,*,#4941,.F.);
#6688=ORIENTED_EDGE('',*,*,#4591,.F.);
#6689=ORIENTED_EDGE('',*,*,#4595,.F.);
#6690=ORIENTED_EDGE('',*,*,#4598,.F.);
#6691=ORIENTED_EDGE('',*,*,#4601,.F.);
#6692=ORIENTED_EDGE('',*,*,#4604,.F.);
#6693=ORIENTED_EDGE('',*,*,#4607,.F.);
#6694=ORIENTED_EDGE('',*,*,#4610,.F.);
#6695=ORIENTED_EDGE('',*,*,#4613,.F.);
#6696=ORIENTED_EDGE('',*,*,#4616,.F.);
#6697=ORIENTED_EDGE('',*,*,#4619,.F.);
#6698=ORIENTED_EDGE('',*,*,#4622,.F.);
#6699=ORIENTED_EDGE('',*,*,#4625,.F.);
#6700=ORIENTED_EDGE('',*,*,#4942,.F.);
#6701=ORIENTED_EDGE('',*,*,#4630,.F.);
#6702=ORIENTED_EDGE('',*,*,#4944,.F.);
#6703=ORIENTED_EDGE('',*,*,#4587,.F.);
#6704=ORIENTED_EDGE('',*,*,#4945,.F.);
#6705=ORIENTED_EDGE('',*,*,#4585,.F.);
#6706=ORIENTED_EDGE('',*,*,#4582,.F.);
#6707=ORIENTED_EDGE('',*,*,#4579,.F.);
#6708=ORIENTED_EDGE('',*,*,#4576,.F.);
#6709=ORIENTED_EDGE('',*,*,#4573,.F.);
#6710=ORIENTED_EDGE('',*,*,#4570,.F.);
#6711=ORIENTED_EDGE('',*,*,#4567,.F.);
#6712=ORIENTED_EDGE('',*,*,#4564,.F.);
#6713=ORIENTED_EDGE('',*,*,#4561,.F.);
#6714=ORIENTED_EDGE('',*,*,#4558,.F.);
#6715=ORIENTED_EDGE('',*,*,#4555,.F.);
#6716=ORIENTED_EDGE('',*,*,#4552,.F.);
#6717=ORIENTED_EDGE('',*,*,#4940,.F.);
#6718=ORIENTED_EDGE('',*,*,#4550,.F.);
#6719=ORIENTED_EDGE('',*,*,#4557,.F.);
#6720=ORIENTED_EDGE('',*,*,#4560,.F.);
#6721=ORIENTED_EDGE('',*,*,#4563,.F.);
#6722=ORIENTED_EDGE('',*,*,#4566,.F.);
#6723=ORIENTED_EDGE('',*,*,#4569,.F.);
#6724=ORIENTED_EDGE('',*,*,#4572,.F.);
#6725=ORIENTED_EDGE('',*,*,#4575,.F.);
#6726=ORIENTED_EDGE('',*,*,#4578,.F.);
#6727=ORIENTED_EDGE('',*,*,#4581,.F.);
#6728=ORIENTED_EDGE('',*,*,#4584,.F.);
#6729=ORIENTED_EDGE('',*,*,#4946,.F.);
#6730=ORIENTED_EDGE('',*,*,#4589,.F.);
#6731=ORIENTED_EDGE('',*,*,#4947,.F.);
#6732=ORIENTED_EDGE('',*,*,#4628,.T.);
#6733=ORIENTED_EDGE('',*,*,#4943,.T.);
#6734=ORIENTED_EDGE('',*,*,#4626,.T.);
#6735=ORIENTED_EDGE('',*,*,#4623,.T.);
#6736=ORIENTED_EDGE('',*,*,#4620,.T.);
#6737=ORIENTED_EDGE('',*,*,#4617,.T.);
#6738=ORIENTED_EDGE('',*,*,#4614,.T.);
#6739=ORIENTED_EDGE('',*,*,#4611,.T.);
#6740=ORIENTED_EDGE('',*,*,#4608,.T.);
#6741=ORIENTED_EDGE('',*,*,#4605,.T.);
#6742=ORIENTED_EDGE('',*,*,#4602,.T.);
#6743=ORIENTED_EDGE('',*,*,#4599,.T.);
#6744=ORIENTED_EDGE('',*,*,#4596,.T.);
#6745=ORIENTED_EDGE('',*,*,#4593,.T.);
#6746=ORIENTED_EDGE('',*,*,#4586,.T.);
#6747=ORIENTED_EDGE('',*,*,#4946,.T.);
#6748=ORIENTED_EDGE('',*,*,#4583,.F.);
#6749=ORIENTED_EDGE('',*,*,#4945,.T.);
#6750=ORIENTED_EDGE('',*,*,#4636,.F.);
#6751=ORIENTED_EDGE('',*,*,#4718,.F.);
#6752=ORIENTED_EDGE('',*,*,#4800,.F.);
#6753=ORIENTED_EDGE('',*,*,#4554,.F.);
#6754=ORIENTED_EDGE('',*,*,#4948,.F.);
#6755=ORIENTED_EDGE('',*,*,#4949,.T.);
#6756=ORIENTED_EDGE('',*,*,#4950,.F.);
#6757=ORIENTED_EDGE('',*,*,#4949,.F.);
#6758=ORIENTED_EDGE('',*,*,#4951,.F.);
#6759=ORIENTED_EDGE('',*,*,#4952,.T.);
#6760=ORIENTED_EDGE('',*,*,#4953,.F.);
#6761=ORIENTED_EDGE('',*,*,#4952,.F.);
#6762=ORIENTED_EDGE('',*,*,#4954,.T.);
#6763=ORIENTED_EDGE('',*,*,#4955,.F.);
#6764=ORIENTED_EDGE('',*,*,#4956,.F.);
#6765=ORIENTED_EDGE('',*,*,#4957,.F.);
#6766=ORIENTED_EDGE('',*,*,#4958,.T.);
#6767=ORIENTED_EDGE('',*,*,#4957,.T.);
#6768=ORIENTED_EDGE('',*,*,#4959,.F.);
#6769=ORIENTED_EDGE('',*,*,#4960,.F.);
#6770=ORIENTED_EDGE('',*,*,#4961,.T.);
#6771=ORIENTED_EDGE('',*,*,#4960,.T.);
#6772=ORIENTED_EDGE('',*,*,#4962,.F.);
#6773=ORIENTED_EDGE('',*,*,#4963,.F.);
#6774=ORIENTED_EDGE('',*,*,#4964,.F.);
#6775=ORIENTED_EDGE('',*,*,#4962,.T.);
#6776=ORIENTED_EDGE('',*,*,#4959,.T.);
#6777=ORIENTED_EDGE('',*,*,#4956,.T.);
#6778=ORIENTED_EDGE('',*,*,#4951,.T.);
#6779=ORIENTED_EDGE('',*,*,#4965,.T.);
#6780=ORIENTED_EDGE('',*,*,#4966,.T.);
#6781=ORIENTED_EDGE('',*,*,#4967,.F.);
#6782=ORIENTED_EDGE('',*,*,#4968,.F.);
#6783=ORIENTED_EDGE('',*,*,#4969,.T.);
#6784=ORIENTED_EDGE('',*,*,#4970,.F.);
#6785=ORIENTED_EDGE('',*,*,#4971,.F.);
#6786=ORIENTED_EDGE('',*,*,#4972,.F.);
#6787=ORIENTED_EDGE('',*,*,#4973,.T.);
#6788=ORIENTED_EDGE('',*,*,#4972,.T.);
#6789=ORIENTED_EDGE('',*,*,#4974,.F.);
#6790=ORIENTED_EDGE('',*,*,#4966,.F.);
#6791=ORIENTED_EDGE('',*,*,#4974,.T.);
#6792=ORIENTED_EDGE('',*,*,#4971,.T.);
#6793=ORIENTED_EDGE('',*,*,#4975,.F.);
#6794=ORIENTED_EDGE('',*,*,#4967,.T.);
#6795=ORIENTED_EDGE('',*,*,#4948,.T.);
#6796=ORIENTED_EDGE('',*,*,#4976,.F.);
#6797=ORIENTED_EDGE('',*,*,#4977,.T.);
#6798=ORIENTED_EDGE('',*,*,#4978,.F.);
#6799=ORIENTED_EDGE('',*,*,#4977,.F.);
#6800=ORIENTED_EDGE('',*,*,#4979,.F.);
#6801=ORIENTED_EDGE('',*,*,#4980,.T.);
#6802=ORIENTED_EDGE('',*,*,#4897,.F.);
#6803=ORIENTED_EDGE('',*,*,#4980,.F.);
#6804=ORIENTED_EDGE('',*,*,#4979,.T.);
#6805=ORIENTED_EDGE('',*,*,#4976,.T.);
#6806=ORIENTED_EDGE('',*,*,#4880,.F.);
#6807=ORIENTED_EDGE('',*,*,#4981,.F.);
#6808=ORIENTED_EDGE('',*,*,#4891,.F.);
#6809=ORIENTED_EDGE('',*,*,#4894,.T.);
#6810=ORIENTED_EDGE('',*,*,#4978,.T.);
#6811=ORIENTED_EDGE('',*,*,#4982,.T.);
#6812=ORIENTED_EDGE('',*,*,#4983,.T.);
#6813=ORIENTED_EDGE('',*,*,#4984,.F.);
#6814=ORIENTED_EDGE('',*,*,#4985,.F.);
#6815=ORIENTED_EDGE('',*,*,#4955,.T.);
#6816=ORIENTED_EDGE('',*,*,#4986,.T.);
#6817=ORIENTED_EDGE('',*,*,#4985,.T.);
#6818=ORIENTED_EDGE('',*,*,#4987,.F.);
#6819=ORIENTED_EDGE('',*,*,#4988,.F.);
#6820=ORIENTED_EDGE('',*,*,#4989,.T.);
#6821=ORIENTED_EDGE('',*,*,#4963,.T.);
#6822=ORIENTED_EDGE('',*,*,#4964,.T.);
#6823=ORIENTED_EDGE('',*,*,#4990,.T.);
#6824=ORIENTED_EDGE('',*,*,#4988,.T.);
#6825=ORIENTED_EDGE('',*,*,#4991,.F.);
#6826=ORIENTED_EDGE('',*,*,#4992,.F.);
#6827=ORIENTED_EDGE('',*,*,#4904,.T.);
#6828=ORIENTED_EDGE('',*,*,#4970,.T.);
#6829=ORIENTED_EDGE('',*,*,#4993,.T.);
#6830=ORIENTED_EDGE('',*,*,#4992,.T.);
#6831=ORIENTED_EDGE('',*,*,#4994,.F.);
#6832=ORIENTED_EDGE('',*,*,#4983,.F.);
#6833=ORIENTED_EDGE('',*,*,#4995,.T.);
#6834=ORIENTED_EDGE('',*,*,#4968,.T.);
#6835=ORIENTED_EDGE('',*,*,#4975,.T.);
#6836=ORIENTED_EDGE('',*,*,#4994,.T.);
#6837=ORIENTED_EDGE('',*,*,#4991,.T.);
#6838=ORIENTED_EDGE('',*,*,#4987,.T.);
#6839=ORIENTED_EDGE('',*,*,#4984,.T.);
#6840=ORIENTED_EDGE('',*,*,#4923,.T.);
#6841=ORIENTED_EDGE('',*,*,#4834,.T.);
#6842=ORIENTED_EDGE('',*,*,#4920,.T.);
#6843=ORIENTED_EDGE('',*,*,#4875,.T.);
#6844=ORIENTED_EDGE('',*,*,#4931,.T.);
#6845=ORIENTED_EDGE('',*,*,#4752,.T.);
#6846=ORIENTED_EDGE('',*,*,#4928,.T.);
#6847=ORIENTED_EDGE('',*,*,#4793,.T.);
#6848=ORIENTED_EDGE('',*,*,#4939,.T.);
#6849=ORIENTED_EDGE('',*,*,#4670,.T.);
#6850=ORIENTED_EDGE('',*,*,#4936,.T.);
#6851=ORIENTED_EDGE('',*,*,#4711,.T.);
#6852=ORIENTED_EDGE('',*,*,#4947,.T.);
#6853=ORIENTED_EDGE('',*,*,#4588,.T.);
#6854=ORIENTED_EDGE('',*,*,#4944,.T.);
#6855=ORIENTED_EDGE('',*,*,#4629,.T.);
#6856=ORIENTED_EDGE('',*,*,#4900,.T.);
#6857=ORIENTED_EDGE('',*,*,#4892,.F.);
#6858=ORIENTED_EDGE('',*,*,#4981,.T.);
#6859=ORIENTED_EDGE('',*,*,#4879,.F.);
#6860=ORIENTED_EDGE('',*,*,#4883,.T.);
#6861=ORIENTED_EDGE('',*,*,#4886,.F.);
#6862=ORIENTED_EDGE('',*,*,#4889,.T.);
#6863=ORIENTED_EDGE('',*,*,#4903,.F.);
#6864=ORIENTED_EDGE('',*,*,#4995,.F.);
#6865=ORIENTED_EDGE('',*,*,#4982,.F.);
#6866=ORIENTED_EDGE('',*,*,#4986,.F.);
#6867=ORIENTED_EDGE('',*,*,#4954,.F.);
#6868=ORIENTED_EDGE('',*,*,#4958,.F.);
#6869=ORIENTED_EDGE('',*,*,#4961,.F.);
#6870=ORIENTED_EDGE('',*,*,#4989,.F.);
#6871=ORIENTED_EDGE('',*,*,#4990,.F.);
#6872=ORIENTED_EDGE('',*,*,#4993,.F.);
#6873=ORIENTED_EDGE('',*,*,#4969,.F.);
#6874=ORIENTED_EDGE('',*,*,#4973,.F.);
#6875=ORIENTED_EDGE('',*,*,#4965,.F.);
#6876=ORIENTED_EDGE('',*,*,#4908,.T.);
#6877=ORIENTED_EDGE('',*,*,#4913,.T.);
#6878=ORIENTED_EDGE('',*,*,#4950,.T.);
#6879=ORIENTED_EDGE('',*,*,#4953,.T.);
#8860=CYLINDRICAL_SURFACE('',#9974,0.1666);
#8861=CYLINDRICAL_SURFACE('',#9977,0.1666);
#8862=CYLINDRICAL_SURFACE('',#9978,0.1666);
#8863=CYLINDRICAL_SURFACE('',#9979,0.1666);
#8864=CYLINDRICAL_SURFACE('',#9980,0.1666);
#8865=CYLINDRICAL_SURFACE('',#9981,0.1666);
#8866=CYLINDRICAL_SURFACE('',#9982,0.1666);
#8867=CYLINDRICAL_SURFACE('',#9983,0.1666);
#8868=CYLINDRICAL_SURFACE('',#9984,0.1666);
#8869=CYLINDRICAL_SURFACE('',#9985,0.1666);
#8870=CYLINDRICAL_SURFACE('',#9986,0.1666);
#8871=CYLINDRICAL_SURFACE('',#9987,0.1666);
#8872=CYLINDRICAL_SURFACE('',#9989,0.205475);
#8873=CYLINDRICAL_SURFACE('',#9991,0.205475);
#8874=CYLINDRICAL_SURFACE('',#9992,0.205475);
#8875=CYLINDRICAL_SURFACE('',#9993,0.205475);
#8876=CYLINDRICAL_SURFACE('',#9994,0.205475);
#8877=CYLINDRICAL_SURFACE('',#9995,0.205475);
#8878=CYLINDRICAL_SURFACE('',#9996,0.205475);
#8879=CYLINDRICAL_SURFACE('',#9997,0.205475);
#8880=CYLINDRICAL_SURFACE('',#9998,0.205475);
#8881=CYLINDRICAL_SURFACE('',#9999,0.205475);
#8882=CYLINDRICAL_SURFACE('',#10000,0.205475);
#8883=CYLINDRICAL_SURFACE('',#10001,0.205475);
#8884=CYLINDRICAL_SURFACE('',#10002,0.205475);
#8885=CYLINDRICAL_SURFACE('',#10004,0.1666);
#8886=CYLINDRICAL_SURFACE('',#10007,0.1666);
#8887=CYLINDRICAL_SURFACE('',#10008,0.1666);
#8888=CYLINDRICAL_SURFACE('',#10009,0.1666);
#8889=CYLINDRICAL_SURFACE('',#10010,0.1666);
#8890=CYLINDRICAL_SURFACE('',#10011,0.1666);
#8891=CYLINDRICAL_SURFACE('',#10012,0.1666);
#8892=CYLINDRICAL_SURFACE('',#10013,0.1666);
#8893=CYLINDRICAL_SURFACE('',#10014,0.1666);
#8894=CYLINDRICAL_SURFACE('',#10015,0.1666);
#8895=CYLINDRICAL_SURFACE('',#10016,0.1666);
#8896=CYLINDRICAL_SURFACE('',#10017,0.1666);
#8897=CYLINDRICAL_SURFACE('',#10019,0.205475000000001);
#8898=CYLINDRICAL_SURFACE('',#10021,0.205475000000001);
#8899=CYLINDRICAL_SURFACE('',#10022,0.205475000000001);
#8900=CYLINDRICAL_SURFACE('',#10023,0.205475000000001);
#8901=CYLINDRICAL_SURFACE('',#10024,0.205475000000001);
#8902=CYLINDRICAL_SURFACE('',#10025,0.205475000000001);
#8903=CYLINDRICAL_SURFACE('',#10026,0.205475000000001);
#8904=CYLINDRICAL_SURFACE('',#10027,0.205475000000001);
#8905=CYLINDRICAL_SURFACE('',#10028,0.205475000000001);
#8906=CYLINDRICAL_SURFACE('',#10029,0.205475000000001);
#8907=CYLINDRICAL_SURFACE('',#10030,0.205475000000001);
#8908=CYLINDRICAL_SURFACE('',#10031,0.205475000000001);
#8909=CYLINDRICAL_SURFACE('',#10032,0.205475000000001);
#8910=CYLINDRICAL_SURFACE('',#10034,0.1666);
#8911=CYLINDRICAL_SURFACE('',#10037,0.1666);
#8912=CYLINDRICAL_SURFACE('',#10038,0.1666);
#8913=CYLINDRICAL_SURFACE('',#10039,0.1666);
#8914=CYLINDRICAL_SURFACE('',#10040,0.1666);
#8915=CYLINDRICAL_SURFACE('',#10041,0.1666);
#8916=CYLINDRICAL_SURFACE('',#10042,0.1666);
#8917=CYLINDRICAL_SURFACE('',#10043,0.1666);
#8918=CYLINDRICAL_SURFACE('',#10044,0.1666);
#8919=CYLINDRICAL_SURFACE('',#10045,0.1666);
#8920=CYLINDRICAL_SURFACE('',#10046,0.1666);
#8921=CYLINDRICAL_SURFACE('',#10047,0.1666);
#8922=CYLINDRICAL_SURFACE('',#10049,0.205475000000001);
#8923=CYLINDRICAL_SURFACE('',#10051,0.205475000000001);
#8924=CYLINDRICAL_SURFACE('',#10052,0.205475000000001);
#8925=CYLINDRICAL_SURFACE('',#10053,0.205475000000001);
#8926=CYLINDRICAL_SURFACE('',#10054,0.205475000000001);
#8927=CYLINDRICAL_SURFACE('',#10055,0.205475000000001);
#8928=CYLINDRICAL_SURFACE('',#10056,0.205475000000001);
#8929=CYLINDRICAL_SURFACE('',#10057,0.205475000000001);
#8930=CYLINDRICAL_SURFACE('',#10058,0.205475000000001);
#8931=CYLINDRICAL_SURFACE('',#10059,0.205475000000001);
#8932=CYLINDRICAL_SURFACE('',#10060,0.205475000000001);
#8933=CYLINDRICAL_SURFACE('',#10061,0.205475000000001);
#8934=CYLINDRICAL_SURFACE('',#10062,0.205475000000001);
#8935=CYLINDRICAL_SURFACE('',#10064,0.1666);
#8936=CYLINDRICAL_SURFACE('',#10067,0.1666);
#8937=CYLINDRICAL_SURFACE('',#10068,0.1666);
#8938=CYLINDRICAL_SURFACE('',#10069,0.1666);
#8939=CYLINDRICAL_SURFACE('',#10070,0.1666);
#8940=CYLINDRICAL_SURFACE('',#10071,0.1666);
#8941=CYLINDRICAL_SURFACE('',#10072,0.1666);
#8942=CYLINDRICAL_SURFACE('',#10073,0.1666);
#8943=CYLINDRICAL_SURFACE('',#10074,0.1666);
#8944=CYLINDRICAL_SURFACE('',#10075,0.1666);
#8945=CYLINDRICAL_SURFACE('',#10076,0.1666);
#8946=CYLINDRICAL_SURFACE('',#10077,0.1666);
#8947=CYLINDRICAL_SURFACE('',#10079,0.205475);
#8948=CYLINDRICAL_SURFACE('',#10081,0.205475);
#8949=CYLINDRICAL_SURFACE('',#10082,0.205475);
#8950=CYLINDRICAL_SURFACE('',#10083,0.205475);
#8951=CYLINDRICAL_SURFACE('',#10084,0.205475);
#8952=CYLINDRICAL_SURFACE('',#10085,0.205475);
#8953=CYLINDRICAL_SURFACE('',#10086,0.205475);
#8954=CYLINDRICAL_SURFACE('',#10087,0.205475);
#8955=CYLINDRICAL_SURFACE('',#10088,0.205475);
#8956=CYLINDRICAL_SURFACE('',#10089,0.205475);
#8957=CYLINDRICAL_SURFACE('',#10090,0.205475);
#8958=CYLINDRICAL_SURFACE('',#10091,0.205475);
#8959=CYLINDRICAL_SURFACE('',#10092,0.205475);
#8960=CYLINDRICAL_SURFACE('',#10094,0.2);
#8961=CYLINDRICAL_SURFACE('',#10098,0.2);
#8962=CYLINDRICAL_SURFACE('',#10102,0.2);
#8963=CYLINDRICAL_SURFACE('',#10112,0.2);
#8964=CYLINDRICAL_SURFACE('',#10114,0.6);
#8965=CYLINDRICAL_SURFACE('',#10119,0.4);
#8966=CYLINDRICAL_SURFACE('',#10121,0.25);
#8967=CYLINDRICAL_SURFACE('',#10125,0.4);
#8968=CYLINDRICAL_SURFACE('',#10127,0.25);
#8969=CYLINDRICAL_SURFACE('',#10129,0.205475);
#8970=CYLINDRICAL_SURFACE('',#10130,0.1666);
#8971=CYLINDRICAL_SURFACE('',#10132,0.205475000000001);
#8972=CYLINDRICAL_SURFACE('',#10133,0.1666);
#8973=CYLINDRICAL_SURFACE('',#10135,0.205475000000001);
#8974=CYLINDRICAL_SURFACE('',#10136,0.1666);
#8975=CYLINDRICAL_SURFACE('',#10138,0.205475);
#8976=CYLINDRICAL_SURFACE('',#10139,0.1666);
#8977=CYLINDRICAL_SURFACE('',#10144,0.3);
#8978=CYLINDRICAL_SURFACE('',#10147,0.3);
#8979=CYLINDRICAL_SURFACE('',#10158,0.65);
#8980=CYLINDRICAL_SURFACE('',#10161,0.8);
#9229=ADVANCED_FACE('',(#439),#8860,.F.);
#9230=ADVANCED_FACE('',(#440),#8861,.F.);
#9231=ADVANCED_FACE('',(#441),#8862,.F.);
#9232=ADVANCED_FACE('',(#442),#8863,.F.);
#9233=ADVANCED_FACE('',(#443),#8864,.F.);
#9234=ADVANCED_FACE('',(#444),#8865,.F.);
#9235=ADVANCED_FACE('',(#445),#8866,.F.);
#9236=ADVANCED_FACE('',(#446),#8867,.F.);
#9237=ADVANCED_FACE('',(#447),#8868,.F.);
#9238=ADVANCED_FACE('',(#448),#8869,.F.);
#9239=ADVANCED_FACE('',(#449),#8870,.F.);
#9240=ADVANCED_FACE('',(#450),#8871,.F.);
#9241=ADVANCED_FACE('',(#451),#8872,.F.);
#9242=ADVANCED_FACE('',(#452),#8873,.F.);
#9243=ADVANCED_FACE('',(#453),#8874,.F.);
#9244=ADVANCED_FACE('',(#454),#8875,.F.);
#9245=ADVANCED_FACE('',(#455),#8876,.F.);
#9246=ADVANCED_FACE('',(#456),#8877,.F.);
#9247=ADVANCED_FACE('',(#457),#8878,.F.);
#9248=ADVANCED_FACE('',(#458),#8879,.F.);
#9249=ADVANCED_FACE('',(#459),#8880,.F.);
#9250=ADVANCED_FACE('',(#460),#8881,.F.);
#9251=ADVANCED_FACE('',(#461),#8882,.F.);
#9252=ADVANCED_FACE('',(#462),#8883,.F.);
#9253=ADVANCED_FACE('',(#463),#8884,.F.);
#9254=ADVANCED_FACE('',(#464),#8885,.F.);
#9255=ADVANCED_FACE('',(#465),#8886,.F.);
#9256=ADVANCED_FACE('',(#466),#8887,.F.);
#9257=ADVANCED_FACE('',(#467),#8888,.F.);
#9258=ADVANCED_FACE('',(#468),#8889,.F.);
#9259=ADVANCED_FACE('',(#469),#8890,.F.);
#9260=ADVANCED_FACE('',(#470),#8891,.F.);
#9261=ADVANCED_FACE('',(#471),#8892,.F.);
#9262=ADVANCED_FACE('',(#472),#8893,.F.);
#9263=ADVANCED_FACE('',(#473),#8894,.F.);
#9264=ADVANCED_FACE('',(#474),#8895,.F.);
#9265=ADVANCED_FACE('',(#475),#8896,.F.);
#9266=ADVANCED_FACE('',(#476),#8897,.F.);
#9267=ADVANCED_FACE('',(#477),#8898,.F.);
#9268=ADVANCED_FACE('',(#478),#8899,.F.);
#9269=ADVANCED_FACE('',(#479),#8900,.F.);
#9270=ADVANCED_FACE('',(#480),#8901,.F.);
#9271=ADVANCED_FACE('',(#481),#8902,.F.);
#9272=ADVANCED_FACE('',(#482),#8903,.F.);
#9273=ADVANCED_FACE('',(#483),#8904,.F.);
#9274=ADVANCED_FACE('',(#484),#8905,.F.);
#9275=ADVANCED_FACE('',(#485),#8906,.F.);
#9276=ADVANCED_FACE('',(#486),#8907,.F.);
#9277=ADVANCED_FACE('',(#487),#8908,.F.);
#9278=ADVANCED_FACE('',(#488),#8909,.F.);
#9279=ADVANCED_FACE('',(#489),#8910,.F.);
#9280=ADVANCED_FACE('',(#490),#8911,.F.);
#9281=ADVANCED_FACE('',(#491),#8912,.F.);
#9282=ADVANCED_FACE('',(#492),#8913,.F.);
#9283=ADVANCED_FACE('',(#493),#8914,.F.);
#9284=ADVANCED_FACE('',(#494),#8915,.F.);
#9285=ADVANCED_FACE('',(#495),#8916,.F.);
#9286=ADVANCED_FACE('',(#496),#8917,.F.);
#9287=ADVANCED_FACE('',(#497),#8918,.F.);
#9288=ADVANCED_FACE('',(#498),#8919,.F.);
#9289=ADVANCED_FACE('',(#499),#8920,.F.);
#9290=ADVANCED_FACE('',(#500),#8921,.F.);
#9291=ADVANCED_FACE('',(#501),#8922,.F.);
#9292=ADVANCED_FACE('',(#502),#8923,.F.);
#9293=ADVANCED_FACE('',(#503),#8924,.F.);
#9294=ADVANCED_FACE('',(#504),#8925,.F.);
#9295=ADVANCED_FACE('',(#505),#8926,.F.);
#9296=ADVANCED_FACE('',(#506),#8927,.F.);
#9297=ADVANCED_FACE('',(#507),#8928,.F.);
#9298=ADVANCED_FACE('',(#508),#8929,.F.);
#9299=ADVANCED_FACE('',(#509),#8930,.F.);
#9300=ADVANCED_FACE('',(#510),#8931,.F.);
#9301=ADVANCED_FACE('',(#511),#8932,.F.);
#9302=ADVANCED_FACE('',(#512),#8933,.F.);
#9303=ADVANCED_FACE('',(#513),#8934,.F.);
#9304=ADVANCED_FACE('',(#514),#8935,.F.);
#9305=ADVANCED_FACE('',(#515),#8936,.F.);
#9306=ADVANCED_FACE('',(#516),#8937,.F.);
#9307=ADVANCED_FACE('',(#517),#8938,.F.);
#9308=ADVANCED_FACE('',(#518),#8939,.F.);
#9309=ADVANCED_FACE('',(#519),#8940,.F.);
#9310=ADVANCED_FACE('',(#520),#8941,.F.);
#9311=ADVANCED_FACE('',(#521),#8942,.F.);
#9312=ADVANCED_FACE('',(#522),#8943,.F.);
#9313=ADVANCED_FACE('',(#523),#8944,.F.);
#9314=ADVANCED_FACE('',(#524),#8945,.F.);
#9315=ADVANCED_FACE('',(#525),#8946,.F.);
#9316=ADVANCED_FACE('',(#526),#8947,.F.);
#9317=ADVANCED_FACE('',(#527),#8948,.F.);
#9318=ADVANCED_FACE('',(#528),#8949,.F.);
#9319=ADVANCED_FACE('',(#529),#8950,.F.);
#9320=ADVANCED_FACE('',(#530),#8951,.F.);
#9321=ADVANCED_FACE('',(#531),#8952,.F.);
#9322=ADVANCED_FACE('',(#532),#8953,.F.);
#9323=ADVANCED_FACE('',(#533),#8954,.F.);
#9324=ADVANCED_FACE('',(#534),#8955,.F.);
#9325=ADVANCED_FACE('',(#535),#8956,.F.);
#9326=ADVANCED_FACE('',(#536),#8957,.F.);
#9327=ADVANCED_FACE('',(#537),#8958,.F.);
#9328=ADVANCED_FACE('',(#538),#8959,.F.);
#9329=ADVANCED_FACE('',(#539),#8960,.F.);
#9330=ADVANCED_FACE('',(#540),#302,.F.);
#9331=ADVANCED_FACE('',(#541),#8961,.F.);
#9332=ADVANCED_FACE('',(#542),#303,.F.);
#9333=ADVANCED_FACE('',(#543),#8962,.F.);
#9334=ADVANCED_FACE('',(#544,#235,#236,#237),#304,.F.);
#9335=ADVANCED_FACE('',(#545,#238),#305,.F.);
#9336=ADVANCED_FACE('',(#546),#8963,.F.);
#9337=ADVANCED_FACE('',(#547),#8964,.F.);
#9338=ADVANCED_FACE('',(#548,#239),#306,.F.);
#9339=ADVANCED_FACE('',(#549),#8965,.F.);
#9340=ADVANCED_FACE('',(#550),#8966,.F.);
#9341=ADVANCED_FACE('',(#551,#240),#307,.F.);
#9342=ADVANCED_FACE('',(#552),#8967,.F.);
#9343=ADVANCED_FACE('',(#553),#8968,.F.);
#9344=ADVANCED_FACE('',(#554),#308,.T.);
#9345=ADVANCED_FACE('',(#555),#8969,.F.);
#9346=ADVANCED_FACE('',(#556),#210,.F.);
#9347=ADVANCED_FACE('',(#557),#211,.F.);
#9348=ADVANCED_FACE('',(#558),#8970,.F.);
#9349=ADVANCED_FACE('',(#559),#309,.T.);
#9350=ADVANCED_FACE('',(#560),#8971,.F.);
#9351=ADVANCED_FACE('',(#561),#212,.F.);
#9352=ADVANCED_FACE('',(#562),#213,.F.);
#9353=ADVANCED_FACE('',(#563),#8972,.F.);
#9354=ADVANCED_FACE('',(#564),#310,.T.);
#9355=ADVANCED_FACE('',(#565),#8973,.F.);
#9356=ADVANCED_FACE('',(#566),#214,.F.);
#9357=ADVANCED_FACE('',(#567),#215,.F.);
#9358=ADVANCED_FACE('',(#568),#8974,.F.);
#9359=ADVANCED_FACE('',(#569),#311,.T.);
#9360=ADVANCED_FACE('',(#570),#8975,.F.);
#9361=ADVANCED_FACE('',(#571),#216,.F.);
#9362=ADVANCED_FACE('',(#572),#217,.F.);
#9363=ADVANCED_FACE('',(#573),#8976,.F.);
#9364=ADVANCED_FACE('',(#574),#312,.F.);
#9365=ADVANCED_FACE('',(#575),#313,.F.);
#9366=ADVANCED_FACE('',(#576),#314,.F.);
#9367=ADVANCED_FACE('',(#577),#315,.F.);
#9368=ADVANCED_FACE('',(#578),#8977,.F.);
#9369=ADVANCED_FACE('',(#579),#8978,.F.);
#9370=ADVANCED_FACE('',(#580),#316,.T.);
#9371=ADVANCED_FACE('',(#581),#317,.T.);
#9372=ADVANCED_FACE('',(#582),#318,.T.);
#9373=ADVANCED_FACE('',(#583,#241),#319,.T.);
#9374=ADVANCED_FACE('',(#584),#320,.T.);
#9375=ADVANCED_FACE('',(#585),#321,.T.);
#9376=ADVANCED_FACE('',(#586),#322,.T.);
#9377=ADVANCED_FACE('',(#587,#242),#323,.T.);
#9378=ADVANCED_FACE('',(#588),#8979,.F.);
#9379=ADVANCED_FACE('',(#589),#8980,.T.);
#9380=ADVANCED_FACE('',(#590,#243),#324,.T.);
#9381=ADVANCED_FACE('',(#591),#325,.F.);
#9382=ADVANCED_FACE('',(#592),#326,.F.);
#9383=ADVANCED_FACE('',(#593),#327,.T.);
#9384=ADVANCED_FACE('',(#594),#328,.T.);
#9385=ADVANCED_FACE('',(#595,#244),#329,.T.);
#9386=ADVANCED_FACE('',(#596),#330,.T.);
#9387=ADVANCED_FACE('',(#597,#245,#246,#247,#248,#249),#331,.T.);
#9388=ADVANCED_FACE('',(#598,#250,#251,#252,#253),#332,.F.);
#9767=CLOSED_SHELL('',(#9229,#9230,#9231,#9232,#9233,#9234,#9235,#9236,
#9237,#9238,#9239,#9240,#9241,#9242,#9243,#9244,#9245,#9246,#9247,#9248,
#9249,#9250,#9251,#9252,#9253,#9254,#9255,#9256,#9257,#9258,#9259,#9260,
#9261,#9262,#9263,#9264,#9265,#9266,#9267,#9268,#9269,#9270,#9271,#9272,
#9273,#9274,#9275,#9276,#9277,#9278,#9279,#9280,#9281,#9282,#9283,#9284,
#9285,#9286,#9287,#9288,#9289,#9290,#9291,#9292,#9293,#9294,#9295,#9296,
#9297,#9298,#9299,#9300,#9301,#9302,#9303,#9304,#9305,#9306,#9307,#9308,
#9309,#9310,#9311,#9312,#9313,#9314,#9315,#9316,#9317,#9318,#9319,#9320,
#9321,#9322,#9323,#9324,#9325,#9326,#9327,#9328,#9329,#9330,#9331,#9332,
#9333,#9334,#9335,#9336,#9337,#9338,#9339,#9340,#9341,#9342,#9343,#9344,
#9345,#9346,#9347,#9348,#9349,#9350,#9351,#9352,#9353,#9354,#9355,#9356,
#9357,#9358,#9359,#9360,#9361,#9362,#9363,#9364,#9365,#9366,#9367,#9368,
#9369,#9370,#9371,#9372,#9373,#9374,#9375,#9376,#9377,#9378,#9379,#9380,
#9381,#9382,#9383,#9384,#9385,#9386,#9387,#9388));
#9973=AXIS2_PLACEMENT_3D('',#12701,#10692,#10693);
#9974=AXIS2_PLACEMENT_3D('',#12702,#10694,#10695);
#9975=AXIS2_PLACEMENT_3D('',#12730,#10697,#10698);
#9976=AXIS2_PLACEMENT_3D('',#12741,#10700,#10701);
#9977=AXIS2_PLACEMENT_3D('',#12764,#10702,#10703);
#9978=AXIS2_PLACEMENT_3D('',#12815,#10705,#10706);
#9979=AXIS2_PLACEMENT_3D('',#12863,#10708,#10709);
#9980=AXIS2_PLACEMENT_3D('',#12911,#10711,#10712);
#9981=AXIS2_PLACEMENT_3D('',#12962,#10714,#10715);
#9982=AXIS2_PLACEMENT_3D('',#13010,#10717,#10718);
#9983=AXIS2_PLACEMENT_3D('',#13058,#10720,#10721);
#9984=AXIS2_PLACEMENT_3D('',#13109,#10723,#10724);
#9985=AXIS2_PLACEMENT_3D('',#13160,#10726,#10727);
#9986=AXIS2_PLACEMENT_3D('',#13208,#10729,#10730);
#9987=AXIS2_PLACEMENT_3D('',#13259,#10732,#10733);
#9988=AXIS2_PLACEMENT_3D('',#13278,#10735,#10736);
#9989=AXIS2_PLACEMENT_3D('',#13298,#10737,#10738);
#9990=AXIS2_PLACEMENT_3D('',#13311,#10740,#10741);
#9991=AXIS2_PLACEMENT_3D('',#13320,#10742,#10743);
#9992=AXIS2_PLACEMENT_3D('',#13344,#10745,#10746);
#9993=AXIS2_PLACEMENT_3D('',#13369,#10748,#10749);
#9994=AXIS2_PLACEMENT_3D('',#13394,#10751,#10752);
#9995=AXIS2_PLACEMENT_3D('',#13418,#10754,#10755);
#9996=AXIS2_PLACEMENT_3D('',#13443,#10757,#10758);
#9997=AXIS2_PLACEMENT_3D('',#13467,#10760,#10761);
#9998=AXIS2_PLACEMENT_3D('',#13492,#10763,#10764);
#9999=AXIS2_PLACEMENT_3D('',#13516,#10766,#10767);
#10000=AXIS2_PLACEMENT_3D('',#13541,#10769,#10770);
#10001=AXIS2_PLACEMENT_3D('',#13566,#10772,#10773);
#10002=AXIS2_PLACEMENT_3D('',#13590,#10775,#10776);
#10003=AXIS2_PLACEMENT_3D('',#13601,#10778,#10779);
#10004=AXIS2_PLACEMENT_3D('',#13607,#10780,#10781);
#10005=AXIS2_PLACEMENT_3D('',#13635,#10783,#10784);
#10006=AXIS2_PLACEMENT_3D('',#13646,#10786,#10787);
#10007=AXIS2_PLACEMENT_3D('',#13669,#10788,#10789);
#10008=AXIS2_PLACEMENT_3D('',#13720,#10791,#10792);
#10009=AXIS2_PLACEMENT_3D('',#13768,#10794,#10795);
#10010=AXIS2_PLACEMENT_3D('',#13816,#10797,#10798);
#10011=AXIS2_PLACEMENT_3D('',#13867,#10800,#10801);
#10012=AXIS2_PLACEMENT_3D('',#13915,#10803,#10804);
#10013=AXIS2_PLACEMENT_3D('',#13963,#10806,#10807);
#10014=AXIS2_PLACEMENT_3D('',#14014,#10809,#10810);
#10015=AXIS2_PLACEMENT_3D('',#14065,#10812,#10813);
#10016=AXIS2_PLACEMENT_3D('',#14113,#10815,#10816);
#10017=AXIS2_PLACEMENT_3D('',#14164,#10818,#10819);
#10018=AXIS2_PLACEMENT_3D('',#14183,#10821,#10822);
#10019=AXIS2_PLACEMENT_3D('',#14203,#10823,#10824);
#10020=AXIS2_PLACEMENT_3D('',#14216,#10826,#10827);
#10021=AXIS2_PLACEMENT_3D('',#14225,#10828,#10829);
#10022=AXIS2_PLACEMENT_3D('',#14249,#10831,#10832);
#10023=AXIS2_PLACEMENT_3D('',#14274,#10834,#10835);
#10024=AXIS2_PLACEMENT_3D('',#14299,#10837,#10838);
#10025=AXIS2_PLACEMENT_3D('',#14323,#10840,#10841);
#10026=AXIS2_PLACEMENT_3D('',#14348,#10843,#10844);
#10027=AXIS2_PLACEMENT_3D('',#14372,#10846,#10847);
#10028=AXIS2_PLACEMENT_3D('',#14397,#10849,#10850);
#10029=AXIS2_PLACEMENT_3D('',#14421,#10852,#10853);
#10030=AXIS2_PLACEMENT_3D('',#14446,#10855,#10856);
#10031=AXIS2_PLACEMENT_3D('',#14471,#10858,#10859);
#10032=AXIS2_PLACEMENT_3D('',#14495,#10861,#10862);
#10033=AXIS2_PLACEMENT_3D('',#14506,#10864,#10865);
#10034=AXIS2_PLACEMENT_3D('',#14512,#10866,#10867);
#10035=AXIS2_PLACEMENT_3D('',#14540,#10869,#10870);
#10036=AXIS2_PLACEMENT_3D('',#14551,#10872,#10873);
#10037=AXIS2_PLACEMENT_3D('',#14574,#10874,#10875);
#10038=AXIS2_PLACEMENT_3D('',#14625,#10877,#10878);
#10039=AXIS2_PLACEMENT_3D('',#14673,#10880,#10881);
#10040=AXIS2_PLACEMENT_3D('',#14721,#10883,#10884);
#10041=AXIS2_PLACEMENT_3D('',#14772,#10886,#10887);
#10042=AXIS2_PLACEMENT_3D('',#14820,#10889,#10890);
#10043=AXIS2_PLACEMENT_3D('',#14868,#10892,#10893);
#10044=AXIS2_PLACEMENT_3D('',#14919,#10895,#10896);
#10045=AXIS2_PLACEMENT_3D('',#14970,#10898,#10899);
#10046=AXIS2_PLACEMENT_3D('',#15018,#10901,#10902);
#10047=AXIS2_PLACEMENT_3D('',#15069,#10904,#10905);
#10048=AXIS2_PLACEMENT_3D('',#15088,#10907,#10908);
#10049=AXIS2_PLACEMENT_3D('',#15108,#10909,#10910);
#10050=AXIS2_PLACEMENT_3D('',#15121,#10912,#10913);
#10051=AXIS2_PLACEMENT_3D('',#15130,#10914,#10915);
#10052=AXIS2_PLACEMENT_3D('',#15154,#10917,#10918);
#10053=AXIS2_PLACEMENT_3D('',#15179,#10920,#10921);
#10054=AXIS2_PLACEMENT_3D('',#15204,#10923,#10924);
#10055=AXIS2_PLACEMENT_3D('',#15228,#10926,#10927);
#10056=AXIS2_PLACEMENT_3D('',#15253,#10929,#10930);
#10057=AXIS2_PLACEMENT_3D('',#15277,#10932,#10933);
#10058=AXIS2_PLACEMENT_3D('',#15302,#10935,#10936);
#10059=AXIS2_PLACEMENT_3D('',#15326,#10938,#10939);
#10060=AXIS2_PLACEMENT_3D('',#15351,#10941,#10942);
#10061=AXIS2_PLACEMENT_3D('',#15376,#10944,#10945);
#10062=AXIS2_PLACEMENT_3D('',#15400,#10947,#10948);
#10063=AXIS2_PLACEMENT_3D('',#15411,#10950,#10951);
#10064=AXIS2_PLACEMENT_3D('',#15417,#10952,#10953);
#10065=AXIS2_PLACEMENT_3D('',#15445,#10955,#10956);
#10066=AXIS2_PLACEMENT_3D('',#15456,#10958,#10959);
#10067=AXIS2_PLACEMENT_3D('',#15479,#10960,#10961);
#10068=AXIS2_PLACEMENT_3D('',#15530,#10963,#10964);
#10069=AXIS2_PLACEMENT_3D('',#15578,#10966,#10967);
#10070=AXIS2_PLACEMENT_3D('',#15626,#10969,#10970);
#10071=AXIS2_PLACEMENT_3D('',#15677,#10972,#10973);
#10072=AXIS2_PLACEMENT_3D('',#15725,#10975,#10976);
#10073=AXIS2_PLACEMENT_3D('',#15773,#10978,#10979);
#10074=AXIS2_PLACEMENT_3D('',#15824,#10981,#10982);
#10075=AXIS2_PLACEMENT_3D('',#15875,#10984,#10985);
#10076=AXIS2_PLACEMENT_3D('',#15923,#10987,#10988);
#10077=AXIS2_PLACEMENT_3D('',#15974,#10990,#10991);
#10078=AXIS2_PLACEMENT_3D('',#15993,#10993,#10994);
#10079=AXIS2_PLACEMENT_3D('',#16013,#10995,#10996);
#10080=AXIS2_PLACEMENT_3D('',#16026,#10998,#10999);
#10081=AXIS2_PLACEMENT_3D('',#16035,#11000,#11001);
#10082=AXIS2_PLACEMENT_3D('',#16059,#11003,#11004);
#10083=AXIS2_PLACEMENT_3D('',#16084,#11006,#11007);
#10084=AXIS2_PLACEMENT_3D('',#16109,#11009,#11010);
#10085=AXIS2_PLACEMENT_3D('',#16133,#11012,#11013);
#10086=AXIS2_PLACEMENT_3D('',#16158,#11015,#11016);
#10087=AXIS2_PLACEMENT_3D('',#16182,#11018,#11019);
#10088=AXIS2_PLACEMENT_3D('',#16207,#11021,#11022);
#10089=AXIS2_PLACEMENT_3D('',#16231,#11024,#11025);
#10090=AXIS2_PLACEMENT_3D('',#16256,#11027,#11028);
#10091=AXIS2_PLACEMENT_3D('',#16281,#11030,#11031);
#10092=AXIS2_PLACEMENT_3D('',#16305,#11033,#11034);
#10093=AXIS2_PLACEMENT_3D('',#16316,#11036,#11037);
#10094=AXIS2_PLACEMENT_3D('',#16322,#11038,#11039);
#10095=AXIS2_PLACEMENT_3D('',#16325,#11040,#11041);
#10096=AXIS2_PLACEMENT_3D('',#16329,#11043,#11044);
#10097=AXIS2_PLACEMENT_3D('',#16331,#11046,#11047);
#10098=AXIS2_PLACEMENT_3D('',#16337,#11051,#11052);
#10099=AXIS2_PLACEMENT_3D('',#16339,#11053,#11054);
#10100=AXIS2_PLACEMENT_3D('',#16342,#11056,#11057);
#10101=AXIS2_PLACEMENT_3D('',#16343,#11058,#11059);
#10102=AXIS2_PLACEMENT_3D('',#16349,#11063,#11064);
#10103=AXIS2_PLACEMENT_3D('',#16352,#11065,#11066);
#10104=AXIS2_PLACEMENT_3D('',#16356,#11068,#11069);
#10105=AXIS2_PLACEMENT_3D('',#16358,#11071,#11072);
#10106=AXIS2_PLACEMENT_3D('',#16362,#11075,#11076);
#10107=AXIS2_PLACEMENT_3D('',#16364,#11077,#11078);
#10108=AXIS2_PLACEMENT_3D('',#16366,#11079,#11080);
#10109=AXIS2_PLACEMENT_3D('',#16368,#11081,#11082);
#10110=AXIS2_PLACEMENT_3D('',#16369,#11083,#11084);
#10111=AXIS2_PLACEMENT_3D('',#16374,#11087,#11088);
#10112=AXIS2_PLACEMENT_3D('',#16375,#11089,#11090);
#10113=AXIS2_PLACEMENT_3D('',#16376,#11091,#11092);
#10114=AXIS2_PLACEMENT_3D('',#16377,#11093,#11094);
#10115=AXIS2_PLACEMENT_3D('',#16379,#11095,#11096);
#10116=AXIS2_PLACEMENT_3D('',#16381,#11098,#11099);
#10117=AXIS2_PLACEMENT_3D('',#16383,#11100,#11101);
#10118=AXIS2_PLACEMENT_3D('',#16385,#11102,#11103);
#10119=AXIS2_PLACEMENT_3D('',#16386,#11104,#11105);
#10120=AXIS2_PLACEMENT_3D('',#16388,#11106,#11107);
#10121=AXIS2_PLACEMENT_3D('',#16390,#11109,#11110);
#10122=AXIS2_PLACEMENT_3D('',#16392,#11112,#11113);
#10123=AXIS2_PLACEMENT_3D('',#16394,#11114,#11115);
#10124=AXIS2_PLACEMENT_3D('',#16396,#11116,#11117);
#10125=AXIS2_PLACEMENT_3D('',#16397,#11118,#11119);
#10126=AXIS2_PLACEMENT_3D('',#16399,#11120,#11121);
#10127=AXIS2_PLACEMENT_3D('',#16401,#11123,#11124);
#10128=AXIS2_PLACEMENT_3D('',#16403,#11126,#11127);
#10129=AXIS2_PLACEMENT_3D('',#16514,#11128,#11129);
#10130=AXIS2_PLACEMENT_3D('',#17375,#11130,#11131);
#10131=AXIS2_PLACEMENT_3D('',#17376,#11132,#11133);
#10132=AXIS2_PLACEMENT_3D('',#17487,#11134,#11135);
#10133=AXIS2_PLACEMENT_3D('',#18348,#11136,#11137);
#10134=AXIS2_PLACEMENT_3D('',#18349,#11138,#11139);
#10135=AXIS2_PLACEMENT_3D('',#18460,#11140,#11141);
#10136=AXIS2_PLACEMENT_3D('',#19321,#11142,#11143);
#10137=AXIS2_PLACEMENT_3D('',#19322,#11144,#11145);
#10138=AXIS2_PLACEMENT_3D('',#19433,#11146,#11147);
#10139=AXIS2_PLACEMENT_3D('',#20294,#11148,#11149);
#10140=AXIS2_PLACEMENT_3D('',#20295,#11150,#11151);
#10141=AXIS2_PLACEMENT_3D('',#20296,#11152,#11153);
#10142=AXIS2_PLACEMENT_3D('',#20297,#11154,#11155);
#10143=AXIS2_PLACEMENT_3D('',#20298,#11156,#11157);
#10144=AXIS2_PLACEMENT_3D('',#20299,#11158,#11159);
#10145=AXIS2_PLACEMENT_3D('',#20301,#11160,#11161);
#10146=AXIS2_PLACEMENT_3D('',#20304,#11163,#11164);
#10147=AXIS2_PLACEMENT_3D('',#20305,#11165,#11166);
#10148=AXIS2_PLACEMENT_3D('',#20307,#11167,#11168);
#10149=AXIS2_PLACEMENT_3D('',#20310,#11170,#11171);
#10150=AXIS2_PLACEMENT_3D('',#20311,#11172,#11173);
#10151=AXIS2_PLACEMENT_3D('',#20320,#11178,#11179);
#10152=AXIS2_PLACEMENT_3D('',#20326,#11183,#11184);
#10153=AXIS2_PLACEMENT_3D('',#20332,#11188,#11189);
#10154=AXIS2_PLACEMENT_3D('',#20334,#11191,#11192);
#10155=AXIS2_PLACEMENT_3D('',#20343,#11197,#11198);
#10156=AXIS2_PLACEMENT_3D('',#20352,#11203,#11204);
#10157=AXIS2_PLACEMENT_3D('',#20355,#11207,#11208);
#10158=AXIS2_PLACEMENT_3D('',#20357,#11210,#11211);
#10159=AXIS2_PLACEMENT_3D('',#20359,#11212,#11213);
#10160=AXIS2_PLACEMENT_3D('',#20362,#11215,#11216);
#10161=AXIS2_PLACEMENT_3D('',#20363,#11217,#11218);
#10162=AXIS2_PLACEMENT_3D('',#20365,#11219,#11220);
#10163=AXIS2_PLACEMENT_3D('',#20367,#11222,#11223);
#10164=AXIS2_PLACEMENT_3D('',#20368,#11224,#11225);
#10165=AXIS2_PLACEMENT_3D('',#20370,#11227,#11228);
#10166=AXIS2_PLACEMENT_3D('',#20371,#11229,#11230);
#10167=AXIS2_PLACEMENT_3D('',#20380,#11235,#11236);
#10168=AXIS2_PLACEMENT_3D('',#20387,#11241,#11242);
#10169=AXIS2_PLACEMENT_3D('',#20393,#11246,#11247);
#10170=AXIS2_PLACEMENT_3D('',#20397,#11251,#11252);
#10171=AXIS2_PLACEMENT_3D('',#20398,#11253,#11254);
#10692=DIRECTION('axis',(0.,0.,1.));
#10693=DIRECTION('refdir',(1.,0.,0.));
#10694=DIRECTION('center_axis',(0.,0.,-1.));
#10695=DIRECTION('ref_axis',(1.,0.,0.));
#10696=DIRECTION('',(0.,0.,-1.));
#10697=DIRECTION('center_axis',(0.,0.,1.));
#10698=DIRECTION('ref_axis',(1.,0.,0.));
#10699=DIRECTION('',(0.,0.,-1.));
#10700=DIRECTION('center_axis',(0.,0.,1.));
#10701=DIRECTION('ref_axis',(1.,0.,0.));
#10702=DIRECTION('center_axis',(0.,0.,-1.));
#10703=DIRECTION('ref_axis',(1.,0.,0.));
#10704=DIRECTION('',(0.,0.,-1.));
#10705=DIRECTION('center_axis',(0.,0.,-1.));
#10706=DIRECTION('ref_axis',(1.,0.,0.));
#10707=DIRECTION('',(0.,0.,-1.));
#10708=DIRECTION('center_axis',(0.,0.,-1.));
#10709=DIRECTION('ref_axis',(1.,0.,0.));
#10710=DIRECTION('',(0.,0.,-1.));
#10711=DIRECTION('center_axis',(0.,0.,-1.));
#10712=DIRECTION('ref_axis',(1.,0.,0.));
#10713=DIRECTION('',(0.,0.,-1.));
#10714=DIRECTION('center_axis',(0.,0.,-1.));
#10715=DIRECTION('ref_axis',(1.,0.,0.));
#10716=DIRECTION('',(0.,0.,-1.));
#10717=DIRECTION('center_axis',(0.,0.,-1.));
#10718=DIRECTION('ref_axis',(1.,0.,0.));
#10719=DIRECTION('',(0.,0.,-1.));
#10720=DIRECTION('center_axis',(0.,0.,-1.));
#10721=DIRECTION('ref_axis',(1.,0.,0.));
#10722=DIRECTION('',(0.,0.,-1.));
#10723=DIRECTION('center_axis',(0.,0.,-1.));
#10724=DIRECTION('ref_axis',(1.,0.,0.));
#10725=DIRECTION('',(0.,0.,-1.));
#10726=DIRECTION('center_axis',(0.,0.,-1.));
#10727=DIRECTION('ref_axis',(1.,0.,0.));
#10728=DIRECTION('',(0.,0.,-1.));
#10729=DIRECTION('center_axis',(0.,0.,-1.));
#10730=DIRECTION('ref_axis',(1.,0.,0.));
#10731=DIRECTION('',(0.,0.,-1.));
#10732=DIRECTION('center_axis',(0.,0.,-1.));
#10733=DIRECTION('ref_axis',(0.938438601292299,-0.345446076261625,0.));
#10734=DIRECTION('',(0.,0.,-1.));
#10735=DIRECTION('center_axis',(0.,0.,-1.));
#10736=DIRECTION('ref_axis',(1.,0.,0.));
#10737=DIRECTION('center_axis',(0.,0.,-1.));
#10738=DIRECTION('ref_axis',(0.450153040552508,0.892951420896642,0.));
#10739=DIRECTION('',(1.22464679914735E-16,-7.42605394171526E-30,-1.));
#10740=DIRECTION('center_axis',(0.,0.,1.));
#10741=DIRECTION('ref_axis',(1.,-6.05158675060312E-14,0.));
#10742=DIRECTION('center_axis',(0.,0.,-1.));
#10743=DIRECTION('ref_axis',(1.,-6.05158675060312E-14,0.));
#10744=DIRECTION('',(1.22464679914735E-16,-7.42605394171526E-30,-1.));
#10745=DIRECTION('center_axis',(0.,0.,-1.));
#10746=DIRECTION('ref_axis',(1.,-6.05158675060312E-14,0.));
#10747=DIRECTION('',(1.22464679914735E-16,-7.42605394171526E-30,-1.));
#10748=DIRECTION('center_axis',(0.,0.,-1.));
#10749=DIRECTION('ref_axis',(1.,-6.05158675060312E-14,0.));
#10750=DIRECTION('',(1.22464679914735E-16,-7.42605394171526E-30,-1.));
#10751=DIRECTION('center_axis',(0.,0.,-1.));
#10752=DIRECTION('ref_axis',(1.,-6.05158675060312E-14,0.));
#10753=DIRECTION('',(1.22464679914735E-16,-7.42605394171526E-30,-1.));
#10754=DIRECTION('center_axis',(0.,0.,-1.));
#10755=DIRECTION('ref_axis',(1.,-6.05158675060312E-14,0.));
#10756=DIRECTION('',(1.22464679914735E-16,-7.42605394171526E-30,-1.));
#10757=DIRECTION('center_axis',(0.,0.,-1.));
#10758=DIRECTION('ref_axis',(1.,-6.05158675060312E-14,0.));
#10759=DIRECTION('',(1.22464679914735E-16,-7.42605394171526E-30,-1.));
#10760=DIRECTION('center_axis',(0.,0.,-1.));
#10761=DIRECTION('ref_axis',(1.,-6.05158675060312E-14,0.));
#10762=DIRECTION('',(1.22464679914735E-16,-7.42605394171526E-30,-1.));
#10763=DIRECTION('center_axis',(0.,0.,-1.));
#10764=DIRECTION('ref_axis',(1.,-6.05158675060312E-14,0.));
#10765=DIRECTION('',(1.22464679914735E-16,-7.42605394171526E-30,-1.));
#10766=DIRECTION('center_axis',(0.,0.,-1.));
#10767=DIRECTION('ref_axis',(1.,-6.05158675060312E-14,0.));
#10768=DIRECTION('',(1.22464679914735E-16,-7.42605394171526E-30,-1.));
#10769=DIRECTION('center_axis',(0.,0.,-1.));
#10770=DIRECTION('ref_axis',(1.,-6.05158675060312E-14,0.));
#10771=DIRECTION('',(1.22464679914735E-16,-7.42605394171526E-30,-1.));
#10772=DIRECTION('center_axis',(0.,0.,-1.));
#10773=DIRECTION('ref_axis',(1.,-6.05158675060312E-14,0.));
#10774=DIRECTION('',(1.22464679914735E-16,-7.42605394171526E-30,-1.));
#10775=DIRECTION('center_axis',(0.,0.,-1.));
#10776=DIRECTION('ref_axis',(-0.609341503082739,-0.792907896682123,0.));
#10777=DIRECTION('',(1.22464679914735E-16,-7.42605394171526E-30,-1.));
#10778=DIRECTION('center_axis',(0.,0.,-1.));
#10779=DIRECTION('ref_axis',(1.,-6.05158675060312E-14,0.));
#10780=DIRECTION('center_axis',(0.,0.,-1.));
#10781=DIRECTION('ref_axis',(1.,0.,0.));
#10782=DIRECTION('',(0.,0.,-1.));
#10783=DIRECTION('center_axis',(0.,0.,1.));
#10784=DIRECTION('ref_axis',(1.,0.,0.));
#10785=DIRECTION('',(0.,0.,-1.));
#10786=DIRECTION('center_axis',(0.,0.,1.));
#10787=DIRECTION('ref_axis',(1.,0.,0.));
#10788=DIRECTION('center_axis',(0.,0.,-1.));
#10789=DIRECTION('ref_axis',(1.,0.,0.));
#10790=DIRECTION('',(0.,0.,-1.));
#10791=DIRECTION('center_axis',(0.,0.,-1.));
#10792=DIRECTION('ref_axis',(1.,0.,0.));
#10793=DIRECTION('',(0.,0.,-1.));
#10794=DIRECTION('center_axis',(0.,0.,-1.));
#10795=DIRECTION('ref_axis',(1.,0.,0.));
#10796=DIRECTION('',(0.,0.,-1.));
#10797=DIRECTION('center_axis',(0.,0.,-1.));
#10798=DIRECTION('ref_axis',(1.,0.,0.));
#10799=DIRECTION('',(0.,0.,-1.));
#10800=DIRECTION('center_axis',(0.,0.,-1.));
#10801=DIRECTION('ref_axis',(1.,0.,0.));
#10802=DIRECTION('',(0.,0.,-1.));
#10803=DIRECTION('center_axis',(0.,0.,-1.));
#10804=DIRECTION('ref_axis',(1.,0.,0.));
#10805=DIRECTION('',(0.,0.,-1.));
#10806=DIRECTION('center_axis',(0.,0.,-1.));
#10807=DIRECTION('ref_axis',(1.,0.,0.));
#10808=DIRECTION('',(0.,0.,-1.));
#10809=DIRECTION('center_axis',(0.,0.,-1.));
#10810=DIRECTION('ref_axis',(1.,0.,0.));
#10811=DIRECTION('',(0.,0.,-1.));
#10812=DIRECTION('center_axis',(0.,0.,-1.));
#10813=DIRECTION('ref_axis',(1.,0.,0.));
#10814=DIRECTION('',(0.,0.,-1.));
#10815=DIRECTION('center_axis',(0.,0.,-1.));
#10816=DIRECTION('ref_axis',(1.,0.,0.));
#10817=DIRECTION('',(0.,0.,-1.));
#10818=DIRECTION('center_axis',(0.,0.,-1.));
#10819=DIRECTION('ref_axis',(0.938438595705222,-0.345446091439475,0.));
#10820=DIRECTION('',(0.,0.,-1.));
#10821=DIRECTION('center_axis',(0.,0.,-1.));
#10822=DIRECTION('ref_axis',(1.,0.,0.));
#10823=DIRECTION('center_axis',(0.,0.,-1.));
#10824=DIRECTION('ref_axis',(0.450153019553355,0.892951431482697,0.));
#10825=DIRECTION('',(1.22464679914735E-16,-6.89669277429462E-30,-1.));
#10826=DIRECTION('center_axis',(0.,0.,1.));
#10827=DIRECTION('ref_axis',(1.,-5.61933055413145E-14,0.));
#10828=DIRECTION('center_axis',(0.,0.,-1.));
#10829=DIRECTION('ref_axis',(1.,-5.61933055413145E-14,0.));
#10830=DIRECTION('',(1.22464679914735E-16,-6.89669277429462E-30,-1.));
#10831=DIRECTION('center_axis',(0.,0.,-1.));
#10832=DIRECTION('ref_axis',(1.,-5.61933055413145E-14,0.));
#10833=DIRECTION('',(1.22464679914735E-16,-6.89669277429462E-30,-1.));
#10834=DIRECTION('center_axis',(0.,0.,-1.));
#10835=DIRECTION('ref_axis',(1.,-5.61933055413145E-14,0.));
#10836=DIRECTION('',(1.22464679914735E-16,-6.89669277429462E-30,-1.));
#10837=DIRECTION('center_axis',(0.,0.,-1.));
#10838=DIRECTION('ref_axis',(1.,-5.61933055413145E-14,0.));
#10839=DIRECTION('',(1.22464679914735E-16,-6.89669277429462E-30,-1.));
#10840=DIRECTION('center_axis',(0.,0.,-1.));
#10841=DIRECTION('ref_axis',(1.,-5.61933055413145E-14,0.));
#10842=DIRECTION('',(1.22464679914735E-16,-6.89669277429462E-30,-1.));
#10843=DIRECTION('center_axis',(0.,0.,-1.));
#10844=DIRECTION('ref_axis',(1.,-5.61933055413145E-14,0.));
#10845=DIRECTION('',(1.22464679914735E-16,-6.89669277429462E-30,-1.));
#10846=DIRECTION('center_axis',(0.,0.,-1.));
#10847=DIRECTION('ref_axis',(1.,-5.61933055413145E-14,0.));
#10848=DIRECTION('',(1.22464679914735E-16,-6.89669277429462E-30,-1.));
#10849=DIRECTION('center_axis',(0.,0.,-1.));
#10850=DIRECTION('ref_axis',(1.,-5.61933055413145E-14,0.));
#10851=DIRECTION('',(1.22464679914735E-16,-6.89669277429462E-30,-1.));
#10852=DIRECTION('center_axis',(0.,0.,-1.));
#10853=DIRECTION('ref_axis',(1.,-5.61933055413145E-14,0.));
#10854=DIRECTION('',(1.22464679914735E-16,-6.89669277429462E-30,-1.));
#10855=DIRECTION('center_axis',(0.,0.,-1.));
#10856=DIRECTION('ref_axis',(1.,-5.61933055413145E-14,0.));
#10857=DIRECTION('',(1.22464679914735E-16,-6.89669277429462E-30,-1.));
#10858=DIRECTION('center_axis',(0.,0.,-1.));
#10859=DIRECTION('ref_axis',(1.,-5.61933055413145E-14,0.));
#10860=DIRECTION('',(1.22464679914735E-16,-6.89669277429462E-30,-1.));
#10861=DIRECTION('center_axis',(0.,0.,-1.));
#10862=DIRECTION('ref_axis',(-0.609341511570002,-0.792907890159749,0.));
#10863=DIRECTION('',(1.22464679914735E-16,-6.89669277429462E-30,-1.));
#10864=DIRECTION('center_axis',(0.,0.,-1.));
#10865=DIRECTION('ref_axis',(1.,-5.61933055413145E-14,0.));
#10866=DIRECTION('center_axis',(0.,0.,-1.));
#10867=DIRECTION('ref_axis',(1.,0.,0.));
#10868=DIRECTION('',(0.,0.,-1.));
#10869=DIRECTION('center_axis',(0.,0.,1.));
#10870=DIRECTION('ref_axis',(1.,0.,0.));
#10871=DIRECTION('',(0.,0.,-1.));
#10872=DIRECTION('center_axis',(0.,0.,1.));
#10873=DIRECTION('ref_axis',(1.,0.,0.));
#10874=DIRECTION('center_axis',(0.,0.,-1.));
#10875=DIRECTION('ref_axis',(1.,0.,0.));
#10876=DIRECTION('',(0.,0.,-1.));
#10877=DIRECTION('center_axis',(0.,0.,-1.));
#10878=DIRECTION('ref_axis',(1.,0.,0.));
#10879=DIRECTION('',(0.,0.,-1.));
#10880=DIRECTION('center_axis',(0.,0.,-1.));
#10881=DIRECTION('ref_axis',(1.,0.,0.));
#10882=DIRECTION('',(0.,0.,-1.));
#10883=DIRECTION('center_axis',(0.,0.,-1.));
#10884=DIRECTION('ref_axis',(1.,0.,0.));
#10885=DIRECTION('',(0.,0.,-1.));
#10886=DIRECTION('center_axis',(0.,0.,-1.));
#10887=DIRECTION('ref_axis',(1.,0.,0.));
#10888=DIRECTION('',(0.,0.,-1.));
#10889=DIRECTION('center_axis',(0.,0.,-1.));
#10890=DIRECTION('ref_axis',(1.,0.,0.));
#10891=DIRECTION('',(0.,0.,-1.));
#10892=DIRECTION('center_axis',(0.,0.,-1.));
#10893=DIRECTION('ref_axis',(1.,0.,0.));
#10894=DIRECTION('',(0.,0.,-1.));
#10895=DIRECTION('center_axis',(0.,0.,-1.));
#10896=DIRECTION('ref_axis',(1.,0.,0.));
#10897=DIRECTION('',(0.,0.,-1.));
#10898=DIRECTION('center_axis',(0.,0.,-1.));
#10899=DIRECTION('ref_axis',(1.,0.,0.));
#10900=DIRECTION('',(0.,0.,-1.));
#10901=DIRECTION('center_axis',(0.,0.,-1.));
#10902=DIRECTION('ref_axis',(1.,0.,0.));
#10903=DIRECTION('',(0.,0.,-1.));
#10904=DIRECTION('center_axis',(0.,0.,-1.));
#10905=DIRECTION('ref_axis',(0.938438617144983,-0.345446033196231,0.));
#10906=DIRECTION('',(0.,0.,-1.));
#10907=DIRECTION('center_axis',(0.,0.,-1.));
#10908=DIRECTION('ref_axis',(1.,0.,0.));
#10909=DIRECTION('center_axis',(0.,0.,-1.));
#10910=DIRECTION('ref_axis',(0.450153067737633,0.892951407192126,0.));
#10911=DIRECTION('',(1.22464679914735E-16,-6.89669277429462E-30,-1.));
#10912=DIRECTION('center_axis',(0.,0.,1.));
#10913=DIRECTION('ref_axis',(1.,-5.61933055413145E-14,0.));
#10914=DIRECTION('center_axis',(0.,0.,-1.));
#10915=DIRECTION('ref_axis',(1.,-5.61933055413145E-14,0.));
#10916=DIRECTION('',(1.22464679914735E-16,-6.89669277429462E-30,-1.));
#10917=DIRECTION('center_axis',(0.,0.,-1.));
#10918=DIRECTION('ref_axis',(1.,-5.61933055413145E-14,0.));
#10919=DIRECTION('',(1.22464679914735E-16,-6.89669277429462E-30,-1.));
#10920=DIRECTION('center_axis',(0.,0.,-1.));
#10921=DIRECTION('ref_axis',(1.,-5.61933055413145E-14,0.));
#10922=DIRECTION('',(1.22464679914735E-16,-6.89669277429462E-30,-1.));
#10923=DIRECTION('center_axis',(0.,0.,-1.));
#10924=DIRECTION('ref_axis',(1.,-5.61933055413145E-14,0.));
#10925=DIRECTION('',(1.22464679914735E-16,-6.89669277429462E-30,-1.));
#10926=DIRECTION('center_axis',(0.,0.,-1.));
#10927=DIRECTION('ref_axis',(1.,-5.61933055413145E-14,0.));
#10928=DIRECTION('',(1.22464679914735E-16,-6.89669277429462E-30,-1.));
#10929=DIRECTION('center_axis',(0.,0.,-1.));
#10930=DIRECTION('ref_axis',(1.,-5.61933055413145E-14,0.));
#10931=DIRECTION('',(1.22464679914735E-16,-6.89669277429462E-30,-1.));
#10932=DIRECTION('center_axis',(0.,0.,-1.));
#10933=DIRECTION('ref_axis',(1.,-5.61933055413145E-14,0.));
#10934=DIRECTION('',(1.22464679914735E-16,-6.89669277429462E-30,-1.));
#10935=DIRECTION('center_axis',(0.,0.,-1.));
#10936=DIRECTION('ref_axis',(1.,-5.61933055413145E-14,0.));
#10937=DIRECTION('',(1.22464679914735E-16,-6.89669277429462E-30,-1.));
#10938=DIRECTION('center_axis',(0.,0.,-1.));
#10939=DIRECTION('ref_axis',(1.,-5.61933055413145E-14,0.));
#10940=DIRECTION('',(1.22464679914735E-16,-6.89669277429462E-30,-1.));
#10941=DIRECTION('center_axis',(0.,0.,-1.));
#10942=DIRECTION('ref_axis',(1.,-5.61933055413145E-14,0.));
#10943=DIRECTION('',(1.22464679914735E-16,-6.89669277429462E-30,-1.));
#10944=DIRECTION('center_axis',(0.,0.,-1.));
#10945=DIRECTION('ref_axis',(1.,-5.61933055413145E-14,0.));
#10946=DIRECTION('',(1.22464679914735E-16,-6.89669277429462E-30,-1.));
#10947=DIRECTION('center_axis',(0.,0.,-1.));
#10948=DIRECTION('ref_axis',(-0.609341520949359,-0.79290788295181,0.));
#10949=DIRECTION('',(1.22464679914735E-16,-6.89669277429462E-30,-1.));
#10950=DIRECTION('center_axis',(0.,0.,-1.));
#10951=DIRECTION('ref_axis',(1.,-5.61933055413145E-14,0.));
#10952=DIRECTION('center_axis',(0.,0.,-1.));
#10953=DIRECTION('ref_axis',(1.,0.,0.));
#10954=DIRECTION('',(0.,0.,-1.));
#10955=DIRECTION('center_axis',(0.,0.,1.));
#10956=DIRECTION('ref_axis',(1.,0.,0.));
#10957=DIRECTION('',(0.,0.,-1.));
#10958=DIRECTION('center_axis',(0.,0.,1.));
#10959=DIRECTION('ref_axis',(1.,0.,0.));
#10960=DIRECTION('center_axis',(0.,0.,-1.));
#10961=DIRECTION('ref_axis',(1.,0.,0.));
#10962=DIRECTION('',(0.,0.,-1.));
#10963=DIRECTION('center_axis',(0.,0.,-1.));
#10964=DIRECTION('ref_axis',(1.,0.,0.));
#10965=DIRECTION('',(0.,0.,-1.));
#10966=DIRECTION('center_axis',(0.,0.,-1.));
#10967=DIRECTION('ref_axis',(1.,0.,0.));
#10968=DIRECTION('',(0.,0.,-1.));
#10969=DIRECTION('center_axis',(0.,0.,-1.));
#10970=DIRECTION('ref_axis',(1.,0.,0.));
#10971=DIRECTION('',(0.,0.,-1.));
#10972=DIRECTION('center_axis',(0.,0.,-1.));
#10973=DIRECTION('ref_axis',(1.,0.,0.));
#10974=DIRECTION('',(0.,0.,-1.));
#10975=DIRECTION('center_axis',(0.,0.,-1.));
#10976=DIRECTION('ref_axis',(1.,0.,0.));
#10977=DIRECTION('',(0.,0.,-1.));
#10978=DIRECTION('center_axis',(0.,0.,-1.));
#10979=DIRECTION('ref_axis',(1.,0.,0.));
#10980=DIRECTION('',(0.,0.,-1.));
#10981=DIRECTION('center_axis',(0.,0.,-1.));
#10982=DIRECTION('ref_axis',(1.,0.,0.));
#10983=DIRECTION('',(0.,0.,-1.));
#10984=DIRECTION('center_axis',(0.,0.,-1.));
#10985=DIRECTION('ref_axis',(1.,0.,0.));
#10986=DIRECTION('',(0.,0.,-1.));
#10987=DIRECTION('center_axis',(0.,0.,-1.));
#10988=DIRECTION('ref_axis',(1.,0.,0.));
#10989=DIRECTION('',(0.,0.,-1.));
#10990=DIRECTION('center_axis',(0.,0.,-1.));
#10991=DIRECTION('ref_axis',(0.938438612980319,-0.345446044509957,0.));
#10992=DIRECTION('',(0.,0.,-1.));
#10993=DIRECTION('center_axis',(0.,0.,-1.));
#10994=DIRECTION('ref_axis',(1.,0.,0.));
#10995=DIRECTION('center_axis',(0.,0.,-1.));
#10996=DIRECTION('ref_axis',(0.450153049056661,0.892951416609544,0.));
#10997=DIRECTION('',(1.22464679914735E-16,-7.42605394171526E-30,-1.));
#10998=DIRECTION('center_axis',(0.,0.,1.));
#10999=DIRECTION('ref_axis',(1.,-6.05158675060312E-14,0.));
#11000=DIRECTION('center_axis',(0.,0.,-1.));
#11001=DIRECTION('ref_axis',(1.,-6.05158675060312E-14,0.));
#11002=DIRECTION('',(1.22464679914735E-16,-7.42605394171526E-30,-1.));
#11003=DIRECTION('center_axis',(0.,0.,-1.));
#11004=DIRECTION('ref_axis',(1.,-6.05158675060312E-14,0.));
#11005=DIRECTION('',(1.22464679914735E-16,-7.42605394171526E-30,-1.));
#11006=DIRECTION('center_axis',(0.,0.,-1.));
#11007=DIRECTION('ref_axis',(1.,-6.05158675060312E-14,0.));
#11008=DIRECTION('',(1.22464679914735E-16,-7.42605394171526E-30,-1.));
#11009=DIRECTION('center_axis',(0.,0.,-1.));
#11010=DIRECTION('ref_axis',(1.,-6.05158675060312E-14,0.));
#11011=DIRECTION('',(1.22464679914735E-16,-7.42605394171526E-30,-1.));
#11012=DIRECTION('center_axis',(0.,0.,-1.));
#11013=DIRECTION('ref_axis',(1.,-6.05158675060312E-14,0.));
#11014=DIRECTION('',(1.22464679914735E-16,-7.42605394171526E-30,-1.));
#11015=DIRECTION('center_axis',(0.,0.,-1.));
#11016=DIRECTION('ref_axis',(1.,-6.05158675060312E-14,0.));
#11017=DIRECTION('',(1.22464679914735E-16,-7.42605394171526E-30,-1.));
#11018=DIRECTION('center_axis',(0.,0.,-1.));
#11019=DIRECTION('ref_axis',(1.,-6.05158675060312E-14,0.));
#11020=DIRECTION('',(1.22464679914735E-16,-7.42605394171526E-30,-1.));
#11021=DIRECTION('center_axis',(0.,0.,-1.));
#11022=DIRECTION('ref_axis',(1.,-6.05158675060312E-14,0.));
#11023=DIRECTION('',(1.22464679914735E-16,-7.42605394171526E-30,-1.));
#11024=DIRECTION('center_axis',(0.,0.,-1.));
#11025=DIRECTION('ref_axis',(1.,-6.05158675060312E-14,0.));
#11026=DIRECTION('',(1.22464679914735E-16,-7.42605394171526E-30,-1.));
#11027=DIRECTION('center_axis',(0.,0.,-1.));
#11028=DIRECTION('ref_axis',(1.,-6.05158675060312E-14,0.));
#11029=DIRECTION('',(1.22464679914735E-16,-7.42605394171526E-30,-1.));
#11030=DIRECTION('center_axis',(0.,0.,-1.));
#11031=DIRECTION('ref_axis',(1.,-6.05158675060312E-14,0.));
#11032=DIRECTION('',(1.22464679914735E-16,-7.42605394171526E-30,-1.));
#11033=DIRECTION('center_axis',(0.,0.,-1.));
#11034=DIRECTION('ref_axis',(-0.609341531225801,-0.792907875054471,0.));
#11035=DIRECTION('',(1.22464679914735E-16,-7.42605394171526E-30,-1.));
#11036=DIRECTION('center_axis',(0.,0.,-1.));
#11037=DIRECTION('ref_axis',(1.,-6.05158675060312E-14,0.));
#11038=DIRECTION('center_axis',(0.,0.,-1.));
#11039=DIRECTION('ref_axis',(-0.707106781186547,0.707106781186547,0.));
#11040=DIRECTION('center_axis',(0.,0.,1.));
#11041=DIRECTION('ref_axis',(-0.707106781186547,0.707106781186547,0.));
#11042=DIRECTION('',(0.,0.,1.));
#11043=DIRECTION('center_axis',(0.,0.,1.));
#11044=DIRECTION('ref_axis',(-0.707106781186547,0.707106781186547,0.));
#11045=DIRECTION('',(0.,0.,-1.));
#11046=DIRECTION('center_axis',(0.,1.,0.));
#11047=DIRECTION('ref_axis',(1.,0.,0.));
#11048=DIRECTION('',(1.,0.,0.));
#11049=DIRECTION('',(0.,0.,-1.));
#11050=DIRECTION('',(1.,0.,0.));
#11051=DIRECTION('center_axis',(0.,0.,-1.));
#11052=DIRECTION('ref_axis',(0.707106781186548,0.707106781186547,0.));
#11053=DIRECTION('center_axis',(0.,0.,1.));
#11054=DIRECTION('ref_axis',(0.707106781186548,0.707106781186547,0.));
#11055=DIRECTION('',(0.,0.,1.));
#11056=DIRECTION('center_axis',(0.,0.,1.));
#11057=DIRECTION('ref_axis',(0.707106781186548,0.707106781186547,0.));
#11058=DIRECTION('center_axis',(1.,0.,0.));
#11059=DIRECTION('ref_axis',(0.,-1.,0.));
#11060=DIRECTION('',(0.,-1.,0.));
#11061=DIRECTION('',(0.,0.,-1.));
#11062=DIRECTION('',(0.,-1.,0.));
#11063=DIRECTION('center_axis',(0.,0.,-1.));
#11064=DIRECTION('ref_axis',(-0.707106781186548,-0.707106781186547,0.));
#11065=DIRECTION('center_axis',(0.,0.,1.));
#11066=DIRECTION('ref_axis',(-0.707106781186548,-0.707106781186547,0.));
#11067=DIRECTION('',(0.,0.,1.));
#11068=DIRECTION('center_axis',(0.,0.,1.));
#11069=DIRECTION('ref_axis',(-0.707106781186548,-0.707106781186547,0.));
#11070=DIRECTION('',(0.,0.,-1.));
#11071=DIRECTION('center_axis',(0.,0.,-1.));
#11072=DIRECTION('ref_axis',(-1.,0.,0.));
#11073=DIRECTION('',(0.,1.,0.));
#11074=DIRECTION('',(-1.,0.,0.));
#11075=DIRECTION('center_axis',(0.,0.,1.));
#11076=DIRECTION('ref_axis',(0.707106781186547,-0.707106781186547,0.));
#11077=DIRECTION('center_axis',(0.,0.,-1.));
#11078=DIRECTION('ref_axis',(1.,0.,0.));
#11079=DIRECTION('center_axis',(0.,0.,-1.));
#11080=DIRECTION('ref_axis',(-1.,0.,0.));
#11081=DIRECTION('center_axis',(0.,0.,-1.));
#11082=DIRECTION('ref_axis',(-1.,0.,0.));
#11083=DIRECTION('center_axis',(0.,-1.,0.));
#11084=DIRECTION('ref_axis',(-1.,0.,0.));
#11085=DIRECTION('',(-1.,0.,0.));
#11086=DIRECTION('',(0.,0.,1.));
#11087=DIRECTION('center_axis',(0.,-1.,0.));
#11088=DIRECTION('ref_axis',(0.,0.,-1.));
#11089=DIRECTION('center_axis',(0.,0.,-1.));
#11090=DIRECTION('ref_axis',(0.707106781186547,-0.707106781186547,0.));
#11091=DIRECTION('center_axis',(0.,0.,1.));
#11092=DIRECTION('ref_axis',(0.707106781186547,-0.707106781186547,0.));
#11093=DIRECTION('center_axis',(0.,1.,0.));
#11094=DIRECTION('ref_axis',(0.,0.,-1.));
#11095=DIRECTION('center_axis',(0.,1.,0.));
#11096=DIRECTION('ref_axis',(0.,0.,-1.));
#11097=DIRECTION('',(0.,1.,0.));
#11098=DIRECTION('center_axis',(0.,0.,1.));
#11099=DIRECTION('ref_axis',(-1.,0.,0.));
#11100=DIRECTION('center_axis',(0.,0.,1.));
#11101=DIRECTION('ref_axis',(-1.,0.,0.));
#11102=DIRECTION('center_axis',(0.,0.,1.));
#11103=DIRECTION('ref_axis',(-1.,0.,0.));
#11104=DIRECTION('center_axis',(0.,0.,1.));
#11105=DIRECTION('ref_axis',(-1.,0.,0.));
#11106=DIRECTION('center_axis',(0.,0.,1.));
#11107=DIRECTION('ref_axis',(-1.,0.,0.));
#11108=DIRECTION('',(0.,0.,1.));
#11109=DIRECTION('center_axis',(0.,0.,1.));
#11110=DIRECTION('ref_axis',(-1.,0.,0.));
#11111=DIRECTION('',(0.,0.,1.));
#11112=DIRECTION('center_axis',(0.,0.,1.));
#11113=DIRECTION('ref_axis',(-1.,0.,0.));
#11114=DIRECTION('center_axis',(0.,0.,1.));
#11115=DIRECTION('ref_axis',(-1.,0.,0.));
#11116=DIRECTION('center_axis',(0.,0.,1.));
#11117=DIRECTION('ref_axis',(-1.,0.,0.));
#11118=DIRECTION('center_axis',(0.,0.,1.));
#11119=DIRECTION('ref_axis',(-1.,0.,0.));
#11120=DIRECTION('center_axis',(0.,0.,1.));
#11121=DIRECTION('ref_axis',(-1.,0.,0.));
#11122=DIRECTION('',(0.,0.,1.));
#11123=DIRECTION('center_axis',(0.,0.,1.));
#11124=DIRECTION('ref_axis',(-1.,0.,0.));
#11125=DIRECTION('',(0.,0.,1.));
#11126=DIRECTION('center_axis',(0.,0.,1.));
#11127=DIRECTION('ref_axis',(1.,0.,0.));
#11128=DIRECTION('center_axis',(0.,0.,-1.));
#11129=DIRECTION('ref_axis',(1.,-6.05158675060312E-14,0.));
#11130=DIRECTION('center_axis',(0.,0.,-1.));
#11131=DIRECTION('ref_axis',(1.,0.,0.));
#11132=DIRECTION('center_axis',(0.,0.,1.));
#11133=DIRECTION('ref_axis',(1.,0.,0.));
#11134=DIRECTION('center_axis',(0.,0.,-1.));
#11135=DIRECTION('ref_axis',(1.,-5.61933055413145E-14,0.));
#11136=DIRECTION('center_axis',(0.,0.,-1.));
#11137=DIRECTION('ref_axis',(1.,0.,0.));
#11138=DIRECTION('center_axis',(0.,0.,1.));
#11139=DIRECTION('ref_axis',(1.,0.,0.));
#11140=DIRECTION('center_axis',(0.,0.,-1.));
#11141=DIRECTION('ref_axis',(1.,-5.61933055413145E-14,0.));
#11142=DIRECTION('center_axis',(0.,0.,-1.));
#11143=DIRECTION('ref_axis',(1.,0.,0.));
#11144=DIRECTION('center_axis',(0.,0.,1.));
#11145=DIRECTION('ref_axis',(1.,0.,0.));
#11146=DIRECTION('center_axis',(0.,0.,-1.));
#11147=DIRECTION('ref_axis',(1.,-6.05158675060312E-14,0.));
#11148=DIRECTION('center_axis',(0.,0.,-1.));
#11149=DIRECTION('ref_axis',(1.,0.,0.));
#11150=DIRECTION('center_axis',(0.,0.,-1.));
#11151=DIRECTION('ref_axis',(1.,0.,0.));
#11152=DIRECTION('center_axis',(0.,0.,-1.));
#11153=DIRECTION('ref_axis',(1.,0.,0.));
#11154=DIRECTION('center_axis',(0.,0.,-1.));
#11155=DIRECTION('ref_axis',(1.,0.,0.));
#11156=DIRECTION('center_axis',(0.,0.,-1.));
#11157=DIRECTION('ref_axis',(1.,0.,0.));
#11158=DIRECTION('center_axis',(0.,0.,-1.));
#11159=DIRECTION('ref_axis',(1.,0.,0.));
#11160=DIRECTION('center_axis',(0.,0.,-1.));
#11161=DIRECTION('ref_axis',(1.,0.,0.));
#11162=DIRECTION('',(0.,0.,-1.));
#11163=DIRECTION('center_axis',(0.,0.,1.));
#11164=DIRECTION('ref_axis',(1.,0.,0.));
#11165=DIRECTION('center_axis',(0.,0.,-1.));
#11166=DIRECTION('ref_axis',(1.,0.,0.));
#11167=DIRECTION('center_axis',(0.,0.,-1.));
#11168=DIRECTION('ref_axis',(1.,0.,0.));
#11169=DIRECTION('',(0.,0.,-1.));
#11170=DIRECTION('center_axis',(0.,0.,1.));
#11171=DIRECTION('ref_axis',(1.,0.,0.));
#11172=DIRECTION('center_axis',(0.,1.,0.));
#11173=DIRECTION('ref_axis',(-1.,0.,0.));
#11174=DIRECTION('',(-1.,0.,0.));
#11175=DIRECTION('',(0.,0.,-1.));
#11176=DIRECTION('',(-1.,0.,0.));
#11177=DIRECTION('',(0.,0.,1.));
#11178=DIRECTION('center_axis',(1.,0.,0.));
#11179=DIRECTION('ref_axis',(0.,1.,0.));
#11180=DIRECTION('',(0.,1.,0.));
#11181=DIRECTION('',(0.,1.,0.));
#11182=DIRECTION('',(0.,0.,1.));
#11183=DIRECTION('center_axis',(0.,-1.,0.));
#11184=DIRECTION('ref_axis',(1.,0.,0.));
#11185=DIRECTION('',(1.,0.,0.));
#11186=DIRECTION('',(1.,0.,0.));
#11187=DIRECTION('',(0.,0.,1.));
#11188=DIRECTION('center_axis',(0.,0.,1.));
#11189=DIRECTION('ref_axis',(1.,0.,0.));
#11190=DIRECTION('',(0.,1.,0.));
#11191=DIRECTION('center_axis',(0.,1.,0.));
#11192=DIRECTION('ref_axis',(-1.,0.,0.));
#11193=DIRECTION('',(-1.,0.,0.));
#11194=DIRECTION('',(0.,0.,1.));
#11195=DIRECTION('',(-1.,0.,0.));
#11196=DIRECTION('',(0.,0.,1.));
#11197=DIRECTION('center_axis',(0.,-1.,0.));
#11198=DIRECTION('ref_axis',(1.,0.,0.));
#11199=DIRECTION('',(1.,0.,0.));
#11200=DIRECTION('',(0.,0.,-1.));
#11201=DIRECTION('',(1.,0.,0.));
#11202=DIRECTION('',(0.,0.,1.));
#11203=DIRECTION('center_axis',(-1.,0.,0.));
#11204=DIRECTION('ref_axis',(0.,-1.,0.));
#11205=DIRECTION('',(0.,-1.,0.));
#11206=DIRECTION('',(0.,-1.,0.));
#11207=DIRECTION('center_axis',(0.,0.,1.));
#11208=DIRECTION('ref_axis',(1.,0.,0.));
#11209=DIRECTION('',(0.,-1.,0.));
#11210=DIRECTION('center_axis',(0.,0.,1.));
#11211=DIRECTION('ref_axis',(1.,0.,0.));
#11212=DIRECTION('center_axis',(0.,0.,-1.));
#11213=DIRECTION('ref_axis',(1.,0.,0.));
#11214=DIRECTION('',(0.,0.,-1.));
#11215=DIRECTION('center_axis',(0.,0.,1.));
#11216=DIRECTION('ref_axis',(1.,0.,0.));
#11217=DIRECTION('center_axis',(0.,0.,1.));
#11218=DIRECTION('ref_axis',(1.,0.,0.));
#11219=DIRECTION('center_axis',(0.,0.,1.));
#11220=DIRECTION('ref_axis',(1.,0.,0.));
#11221=DIRECTION('',(0.,0.,-1.));
#11222=DIRECTION('center_axis',(0.,0.,1.));
#11223=DIRECTION('ref_axis',(1.,0.,0.));
#11224=DIRECTION('center_axis',(-1.,0.,0.));
#11225=DIRECTION('ref_axis',(0.,1.,0.));
#11226=DIRECTION('',(0.,1.,0.));
#11227=DIRECTION('center_axis',(0.,0.,-1.));
#11228=DIRECTION('ref_axis',(-1.,0.,0.));
#11229=DIRECTION('center_axis',(0.,1.,0.));
#11230=DIRECTION('ref_axis',(-1.,0.,0.));
#11231=DIRECTION('',(-1.,0.,0.));
#11232=DIRECTION('',(0.,0.,1.));
#11233=DIRECTION('',(-1.,0.,0.));
#11234=DIRECTION('',(0.,0.,1.));
#11235=DIRECTION('center_axis',(1.,0.,0.));
#11236=DIRECTION('ref_axis',(0.,1.,0.));
#11237=DIRECTION('',(0.,1.,0.));
#11238=DIRECTION('',(0.,1.,0.));
#11239=DIRECTION('',(0.,0.,1.));
#11240=DIRECTION('',(0.,1.,0.));
#11241=DIRECTION('center_axis',(0.,-1.,0.));
#11242=DIRECTION('ref_axis',(1.,0.,0.));
#11243=DIRECTION('',(1.,0.,0.));
#11244=DIRECTION('',(1.,0.,0.));
#11245=DIRECTION('',(0.,0.,1.));
#11246=DIRECTION('center_axis',(-1.,0.,0.));
#11247=DIRECTION('ref_axis',(0.,-1.,0.));
#11248=DIRECTION('',(0.,-1.,0.));
#11249=DIRECTION('',(0.,-1.,0.));
#11250=DIRECTION('',(0.,-1.,0.));
#11251=DIRECTION('center_axis',(0.,0.,1.));
#11252=DIRECTION('ref_axis',(1.,0.,0.));
#11253=DIRECTION('center_axis',(0.,0.,1.));
#11254=DIRECTION('ref_axis',(1.,0.,0.));
#12701=CARTESIAN_POINT('',(0.,0.,0.));
#12702=CARTESIAN_POINT('Origin',(3.6,2.4,4.7));
#12703=CARTESIAN_POINT('',(3.43324411482341,2.39987855685961,4.38714803633902));
#12704=CARTESIAN_POINT('',(3.43319917606922,2.4000969362753,4.36785196366098));
#12705=CARTESIAN_POINT('',(3.4334,2.4,4.7));
#12706=CARTESIAN_POINT('',(3.43648706727485,2.36807695453719,4.3));
#12707=CARTESIAN_POINT('Ctrl Pts',(3.43319917606922,2.4000969362753,4.36785196366098));
#12708=CARTESIAN_POINT('Ctrl Pts',(3.43315841823699,2.40590556741068,4.36746222055426));
#12709=CARTESIAN_POINT('Ctrl Pts',(3.43343543893775,2.41171030674387,4.36707247744754));
#12710=CARTESIAN_POINT('Ctrl Pts',(3.43404307301465,2.41748025740019,4.36668273434083));
#12711=CARTESIAN_POINT('Ctrl Pts',(3.43981877230484,2.47232494300381,4.36297813798856));
#12712=CARTESIAN_POINT('Ctrl Pts',(3.475465166407,2.52402649519299,4.35927354163629));
#12713=CARTESIAN_POINT('Ctrl Pts',(3.52467802575654,2.54891438715568,4.35556894528402));
#12714=CARTESIAN_POINT('Ctrl Pts',(3.57389088510608,2.57380227911837,4.35186434893175));
#12715=CARTESIAN_POINT('Ctrl Pts',(3.636670209703,2.57187651085455,4.34815975257948));
#12716=CARTESIAN_POINT('Ctrl Pts',(3.68426556342447,2.54403648109996,4.34445515622722));
#12717=CARTESIAN_POINT('Ctrl Pts',(3.73186091714595,2.51619645134536,4.34075055987495));
#12718=CARTESIAN_POINT('Ctrl Pts',(3.76427229999197,2.46244216009999,4.33704596352268));
#12719=CARTESIAN_POINT('Ctrl Pts',(3.76670490932883,2.40733835348838,4.33334136717041));
#12720=CARTESIAN_POINT('Ctrl Pts',(3.76913751866569,2.35223454687676,4.32963677081814));
#12721=CARTESIAN_POINT('Ctrl Pts',(3.74159135449339,2.29578122489891,4.32593217446588));
#12722=CARTESIAN_POINT('Ctrl Pts',(3.69659413605431,2.26388777656513,4.32222757811361));
#12723=CARTESIAN_POINT('Ctrl Pts',(3.65159691761524,2.23199432823136,4.31852298176134));
#12724=CARTESIAN_POINT('Ctrl Pts',(3.5891486449094,2.22466075354166,4.31481838540907));
#12725=CARTESIAN_POINT('Ctrl Pts',(3.53802497534865,2.24508842505152,4.3111137890568));
#12726=CARTESIAN_POINT('Ctrl Pts',(3.4869013057879,2.26551609656139,4.30740919270454));
#12727=CARTESIAN_POINT('Ctrl Pts',(3.44710223937223,2.31370501427082,4.30370459635227));
#12728=CARTESIAN_POINT('Ctrl Pts',(3.43648706727485,2.36807695453719,4.3));
#12729=CARTESIAN_POINT('',(3.5947433343941,2.5668198697629,4.3));
#12730=CARTESIAN_POINT('Origin',(3.6,2.4,4.3));
#12731=CARTESIAN_POINT('',(3.43365448824955,2.39993503013922,4.31714803633902));
#12732=CARTESIAN_POINT('Ctrl Pts',(3.59474333802771,2.56682006235004,4.3));
#12733=CARTESIAN_POINT('Ctrl Pts',(3.54069368762274,2.56504680898901,4.30363229181856));
#12734=CARTESIAN_POINT('Ctrl Pts',(3.48748281235487,2.53457817870515,4.30726458363711));
#12735=CARTESIAN_POINT('Ctrl Pts',(3.45871386452964,2.48878411340601,4.31089687545566));
#12736=CARTESIAN_POINT('Ctrl Pts',(3.44221011333674,2.46251364065879,4.31298059575012));
#12737=CARTESIAN_POINT('Ctrl Pts',(3.43375000591375,2.43119968923457,4.31506431604457));
#12738=CARTESIAN_POINT('Ctrl Pts',(3.43365448824955,2.39993503013922,4.31714803633902));
#12739=CARTESIAN_POINT('',(3.4334,2.4,4.2));
#12740=CARTESIAN_POINT('',(3.4334,2.4,4.7));
#12741=CARTESIAN_POINT('Origin',(3.6,2.4,4.2));
#12742=CARTESIAN_POINT('Ctrl Pts',(3.43365448824955,2.39993503013922,4.31714803633902));
#12743=CARTESIAN_POINT('Ctrl Pts',(3.4335801873487,2.37561500142982,4.31876891239684));
#12744=CARTESIAN_POINT('Ctrl Pts',(3.43856722533918,2.35132479907035,4.32038978845465));
#12745=CARTESIAN_POINT('Ctrl Pts',(3.44876666696164,2.32946151839122,4.32201066451247));
#12746=CARTESIAN_POINT('Ctrl Pts',(3.47207802013238,2.27949185571287,4.32571526086474));
#12747=CARTESIAN_POINT('Ctrl Pts',(3.52261765366037,2.24219981905568,4.32941985721701));
#12748=CARTESIAN_POINT('Ctrl Pts',(3.57725038766107,2.23467802743392,4.33312445356927));
#12749=CARTESIAN_POINT('Ctrl Pts',(3.63188312166177,2.22715623581217,4.33682904992154));
#12750=CARTESIAN_POINT('Ctrl Pts',(3.69060895613519,2.24940468922586,4.34053364627381));
#12751=CARTESIAN_POINT('Ctrl Pts',(3.72655438764877,2.29122842499976,4.34423824262608));
#12752=CARTESIAN_POINT('Ctrl Pts',(3.76249981916235,2.33305216077365,4.34794283897835));
#12753=CARTESIAN_POINT('Ctrl Pts',(3.77566484771609,2.39445117890775,4.35164743533062));
#12754=CARTESIAN_POINT('Ctrl Pts',(3.76002307153489,2.44733227776831,4.35535203168288));
#12755=CARTESIAN_POINT('Ctrl Pts',(3.7443812953537,2.50021337662887,4.35905662803515));
#12756=CARTESIAN_POINT('Ctrl Pts',(3.69993271443756,2.5445765562159,4.36276122438742));
#12757=CARTESIAN_POINT('Ctrl Pts',(3.64702014888419,2.56011555645441,4.36646582073968));
#12758=CARTESIAN_POINT('Ctrl Pts',(3.59410758333083,2.57565455669293,4.37017041709195));
#12759=CARTESIAN_POINT('Ctrl Pts',(3.53273103314024,2.56236937758293,4.37387501344422));
#12760=CARTESIAN_POINT('Ctrl Pts',(3.49097948747713,2.52634165427837,4.37757960979649));
#12761=CARTESIAN_POINT('Ctrl Pts',(3.45503345721934,2.49532355395523,4.38076908531067));
#12762=CARTESIAN_POINT('Ctrl Pts',(3.43363419524109,2.44744785138174,4.38395856082484));
#12763=CARTESIAN_POINT('Ctrl Pts',(3.43324411482341,2.39987855685961,4.38714803633902));
#12764=CARTESIAN_POINT('Origin',(3.6,2.4,4.7));
#12765=CARTESIAN_POINT('',(3.43327529856389,2.40013247750357,4.45714803633902));
#12766=CARTESIAN_POINT('',(3.43362892985438,2.40008323250784,4.43785196366098));
#12767=CARTESIAN_POINT('',(3.4334,2.4,4.7));
#12768=CARTESIAN_POINT('Ctrl Pts',(3.43362892985438,2.40008323250784,4.43785196366098));
#12769=CARTESIAN_POINT('Ctrl Pts',(3.43352744619908,2.42251958229607,4.43635646533454));
#12770=CARTESIAN_POINT('Ctrl Pts',(3.43774838281902,2.44491933756368,4.43486096700809));
#12771=CARTESIAN_POINT('Ctrl Pts',(3.44647310901037,2.4654005396039,4.43336546868165));
#12772=CARTESIAN_POINT('Ctrl Pts',(3.46808569676891,2.5161358597488,4.42966087232938));
#12773=CARTESIAN_POINT('Ctrl Pts',(3.51733510120548,2.55509827110394,4.42595627597712));
#12774=CARTESIAN_POINT('Ctrl Pts',(3.57168220127168,2.56445626518835,4.42225167962485));
#12775=CARTESIAN_POINT('Ctrl Pts',(3.62602930133789,2.57381425927275,4.41854708327258));
#12776=CARTESIAN_POINT('Ctrl Pts',(3.68547409703373,2.55356783608644,4.41484248692031));
#12777=CARTESIAN_POINT('Ctrl Pts',(3.7228110439026,2.51298316629394,4.41113789056804));
#12778=CARTESIAN_POINT('Ctrl Pts',(3.76014799077148,2.47239849650144,4.40743329421577));
#12779=CARTESIAN_POINT('Ctrl Pts',(3.77537708881339,2.41147558010275,4.4037286978635));
#12780=CARTESIAN_POINT('Ctrl Pts',(3.76152924886074,2.35809557405986,4.40002410151124));
#12781=CARTESIAN_POINT('Ctrl Pts',(3.74768140890809,2.30471556801697,4.39631950515897));
#12782=CARTESIAN_POINT('Ctrl Pts',(3.70475663096088,2.25887847232986,4.3926149088067));
#12783=CARTESIAN_POINT('Ctrl Pts',(3.65239849394634,2.24156301733926,4.38891031245443));
#12784=CARTESIAN_POINT('Ctrl Pts',(3.6000403569318,2.22424756234866,4.38520571610217));
#12785=CARTESIAN_POINT('Ctrl Pts',(3.53824886084993,2.23545374805455,4.3815011197499));
#12786=CARTESIAN_POINT('Ctrl Pts',(3.49530561504809,2.27005075041653,4.37779652339763));
#12787=CARTESIAN_POINT('Ctrl Pts',(3.45688022556308,2.30100796536268,4.37448167015208));
#12788=CARTESIAN_POINT('Ctrl Pts',(3.43354583064794,2.35069321510765,4.37116681690653));
#12789=CARTESIAN_POINT('Ctrl Pts',(3.43319917606922,2.4000969362753,4.36785196366098));
#12790=CARTESIAN_POINT('Ctrl Pts',(3.43324411482341,2.39987855685961,4.38714803633902));
#12791=CARTESIAN_POINT('Ctrl Pts',(3.43318111432356,2.39219580941329,4.38766315717711));
#12792=CARTESIAN_POINT('Ctrl Pts',(3.4336661242569,2.38452105441581,4.3881782780152));
#12793=CARTESIAN_POINT('Ctrl Pts',(3.43472636939645,2.37692660019285,4.38869339885329));
#12794=CARTESIAN_POINT('Ctrl Pts',(3.44235133811452,2.32230953691099,4.39239799520556));
#12795=CARTESIAN_POINT('Ctrl Pts',(3.47972781668628,2.27184567784637,4.39610259155783));
#12796=CARTESIAN_POINT('Ctrl Pts',(3.52975016370933,2.24863049260891,4.3998071879101));
#12797=CARTESIAN_POINT('Ctrl Pts',(3.57977251073239,2.22541530737146,4.40351178426237));
#12798=CARTESIAN_POINT('Ctrl Pts',(3.64244072620675,2.22944879596115,4.40721638061463));
#12799=CARTESIAN_POINT('Ctrl Pts',(3.6890743879353,2.25888481053352,4.4109209769669));
#12800=CARTESIAN_POINT('Ctrl Pts',(3.73570804966386,2.28832082510588,4.41462557331917));
#12801=CARTESIAN_POINT('Ctrl Pts',(3.76630715764661,2.34315936566092,4.41833016967144));
#12802=CARTESIAN_POINT('Ctrl Pts',(3.76686783565003,2.39830336248822,4.4220347660237));
#12803=CARTESIAN_POINT('Ctrl Pts',(3.76742851365345,2.45344735931552,4.42573936237597));
#12804=CARTESIAN_POINT('Ctrl Pts',(3.73795076167754,2.5088968124151,4.42944395872824));
#12805=CARTESIAN_POINT('Ctrl Pts',(3.69192525052887,2.53927491555576,4.43314855508051));
#12806=CARTESIAN_POINT('Ctrl Pts',(3.6458997393802,2.56965301869642,4.43685315143278));
#12807=CARTESIAN_POINT('Ctrl Pts',(3.58332646905877,2.57495977187817,4.44055774778505));
#12808=CARTESIAN_POINT('Ctrl Pts',(3.5328424463163,2.55276653418389,4.44426234413732));
#12809=CARTESIAN_POINT('Ctrl Pts',(3.48235842357382,2.53057329648961,4.44796694048958));
#12810=CARTESIAN_POINT('Ctrl Pts',(3.4439636484103,2.4808800679193,4.45167153684185));
#12811=CARTESIAN_POINT('Ctrl Pts',(3.43522971000183,2.42642922394017,4.45537613319412));
#12812=CARTESIAN_POINT('Ctrl Pts',(3.43383723324577,2.41774797030146,4.45596676757575));
#12813=CARTESIAN_POINT('Ctrl Pts',(3.43319870043454,2.40894578361697,4.45655740195739));
#12814=CARTESIAN_POINT('Ctrl Pts',(3.43327529856389,2.40013247750357,4.45714803633902));
#12815=CARTESIAN_POINT('Origin',(3.6,2.4,4.7));
#12816=CARTESIAN_POINT('',(3.43366207255012,2.4000380247868,4.52714803633902));
#12817=CARTESIAN_POINT('',(3.43350143198867,2.39985687063426,4.50785196366098));
#12818=CARTESIAN_POINT('',(3.4334,2.4,4.7));
#12819=CARTESIAN_POINT('Ctrl Pts',(3.43350143198867,2.39985687063426,4.50785196366098));
#12820=CARTESIAN_POINT('Ctrl Pts',(3.43382054827219,2.43880728393095,4.50525071011481));
#12821=CARTESIAN_POINT('Ctrl Pts',(3.44745633991989,2.47795898515992,4.50264945656865));
#12822=CARTESIAN_POINT('Ctrl Pts',(3.47241574712106,2.50756395301054,4.50004820302248));
#12823=CARTESIAN_POINT('Ctrl Pts',(3.50796188948324,2.54972610827987,4.49634360667021));
#12824=CARTESIAN_POINT('Ctrl Pts',(3.56647488720154,2.57252532742787,4.49263901031794));
#12825=CARTESIAN_POINT('Ctrl Pts',(3.62117593737884,2.56552741635789,4.48893441396567));
#12826=CARTESIAN_POINT('Ctrl Pts',(3.67587698755613,2.55852950528791,4.4852298176134));
#12827=CARTESIAN_POINT('Ctrl Pts',(3.72676609019243,2.52173446399995,4.48152522126113));
#12828=CARTESIAN_POINT('Ctrl Pts',(3.75055355430056,2.47198175613265,4.47782062490887));
#12829=CARTESIAN_POINT('Ctrl Pts',(3.77434101840868,2.42222904826535,4.4741160285566));
#12830=CARTESIAN_POINT('Ctrl Pts',(3.77102684398863,2.3595186738187,4.47041143220433));
#12831=CARTESIAN_POINT('Ctrl Pts',(3.74212779097605,2.31255038253853,4.46670683585206));
#12832=CARTESIAN_POINT('Ctrl Pts',(3.71322873796346,2.26558209125837,4.4630022394998));
#12833=CARTESIAN_POINT('Ctrl Pts',(3.65874480635833,2.23435588314469,4.45929764314753));
#12834=CARTESIAN_POINT('Ctrl Pts',(3.60361085794536,2.23316262684763,4.45559304679526));
#12835=CARTESIAN_POINT('Ctrl Pts',(3.54847690953239,2.23196937055057,4.45188845044299));
#12836=CARTESIAN_POINT('Ctrl Pts',(3.49269294431159,2.26080906607012,4.44818385409072));
#12837=CARTESIAN_POINT('Ctrl Pts',(3.46178884724144,2.30648302829723,4.44447925773845));
#12838=CARTESIAN_POINT('Ctrl Pts',(3.44336034023669,2.33371899416048,4.44227015971263));
#12839=CARTESIAN_POINT('Ctrl Pts',(3.43377883797438,2.36694103826561,4.44006106168681));
#12840=CARTESIAN_POINT('Ctrl Pts',(3.43362892985438,2.40008323250784,4.43785196366098));
#12841=CARTESIAN_POINT('Ctrl Pts',(3.43327529856389,2.40013247750357,4.45714803633902));
#12842=CARTESIAN_POINT('Ctrl Pts',(3.43367914173529,2.35366667577227,4.46026199830965));
#12843=CARTESIAN_POINT('Ctrl Pts',(3.45396107839716,2.3068917935147,4.46337596028029));
#12844=CARTESIAN_POINT('Ctrl Pts',(3.48843309004669,2.27590093912579,4.46648992225093));
#12845=CARTESIAN_POINT('Ctrl Pts',(3.52944351015346,2.23903195767851,4.47019451860319));
#12846=CARTESIAN_POINT('Ctrl Pts',(3.59053745202041,2.22450245417194,4.47389911495546));
#12847=CARTESIAN_POINT('Ctrl Pts',(3.64375492737657,2.23896193518984,4.47760371130773));
#12848=CARTESIAN_POINT('Ctrl Pts',(3.69697240273272,2.25342141620775,4.48130830765999));
#12849=CARTESIAN_POINT('Ctrl Pts',(3.74231341157808,2.29686988175014,4.48501290401227));
#12850=CARTESIAN_POINT('Ctrl Pts',(3.75902738378866,2.34942289673192,4.48871750036453));
#12851=CARTESIAN_POINT('Ctrl Pts',(3.77574135599923,2.40197591171369,4.4924220967168));
#12852=CARTESIAN_POINT('Ctrl Pts',(3.76382829157503,2.46363347613485,4.49612669306907));
#12853=CARTESIAN_POINT('Ctrl Pts',(3.7287402721637,2.50617765524692,4.49983128942134));
#12854=CARTESIAN_POINT('Ctrl Pts',(3.69365225275236,2.54872183435899,4.5035358857736));
#12855=CARTESIAN_POINT('Ctrl Pts',(3.63538927835389,2.57215262816197,4.50724048212587));
#12856=CARTESIAN_POINT('Ctrl Pts',(3.58061572949426,2.56574680139426,4.51094507847814));
#12857=CARTESIAN_POINT('Ctrl Pts',(3.52584218063463,2.55934097462656,4.51464967483041));
#12858=CARTESIAN_POINT('Ctrl Pts',(3.47455805731385,2.52309852728818,4.51835427118268));
#12859=CARTESIAN_POINT('Ctrl Pts',(3.45023382941089,2.47360602072044,4.52205886753494));
#12860=CARTESIAN_POINT('Ctrl Pts',(3.43909540477512,2.45094266808951,4.5237552571363));
#12861=CARTESIAN_POINT('Ctrl Pts',(3.43361009249165,2.42550096367579,4.52545164673766));
#12862=CARTESIAN_POINT('Ctrl Pts',(3.43366207255012,2.4000380247868,4.52714803633902));
#12863=CARTESIAN_POINT('Origin',(3.6,2.4,4.7));
#12864=CARTESIAN_POINT('',(3.43341474631901,2.39984765669014,4.59714803633902));
#12865=CARTESIAN_POINT('',(3.43312356359968,2.40000067112034,4.57785196366098));
#12866=CARTESIAN_POINT('',(3.4334,2.4,4.7));
#12867=CARTESIAN_POINT('Ctrl Pts',(3.43312356496403,2.40000067111703,4.57785196366098));
#12868=CARTESIAN_POINT('Ctrl Pts',(3.43312026903532,2.45518344011976,4.57414495489509));
#12869=CARTESIAN_POINT('Ctrl Pts',(3.46320502523792,2.51036311996034,4.5704379461292));
#12870=CARTESIAN_POINT('Ctrl Pts',(3.50958660620738,2.54026105638185,4.5667309373633));
#12871=CARTESIAN_POINT('Ctrl Pts',(3.55593800339121,2.57013953609479,4.56302634101103));
#12872=CARTESIAN_POINT('Ctrl Pts',(3.6185650095987,2.57476916693782,4.55932174465876));
#12873=CARTESIAN_POINT('Ctrl Pts',(3.66880602035543,2.55203117207009,4.55561714830649));
#12874=CARTESIAN_POINT('Ctrl Pts',(3.71904703111215,2.52929317720236,4.55191255195423));
#12875=CARTESIAN_POINT('Ctrl Pts',(3.7569020464181,2.47918755662387,4.54820795560196));
#12876=CARTESIAN_POINT('Ctrl Pts',(3.76504650379449,2.42464543177811,4.54450335924969));
#12877=CARTESIAN_POINT('Ctrl Pts',(3.77319096117088,2.37010330693235,4.54079876289743));
#12878=CARTESIAN_POINT('Ctrl Pts',(3.75162486061771,2.31112467781931,4.53709416654516));
#12879=CARTESIAN_POINT('Ctrl Pts',(3.71021805048437,2.27470144834891,4.53338957019289));
#12880=CARTESIAN_POINT('Ctrl Pts',(3.66881124035102,2.23827821887852,4.52968497384062));
#12881=CARTESIAN_POINT('Ctrl Pts',(3.60756372063751,2.22441038905077,4.52598037748835));
#12882=CARTESIAN_POINT('Ctrl Pts',(3.55450576575121,2.23944465009304,4.52227578113609));
#12883=CARTESIAN_POINT('Ctrl Pts',(3.50144781086492,2.25447891113532,4.51857118478382));
#12884=CARTESIAN_POINT('Ctrl Pts',(3.45657942080584,2.29841526304761,4.51486658843155));
#12885=CARTESIAN_POINT('Ctrl Pts',(3.44043486927933,2.35114598469909,4.51116199207928));
#12886=CARTESIAN_POINT('Ctrl Pts',(3.43562652497117,2.36685081644385,4.51005864927318));
#12887=CARTESIAN_POINT('Ctrl Pts',(3.43336607622673,2.38333573667221,4.50895530646708));
#12888=CARTESIAN_POINT('Ctrl Pts',(3.43350143198867,2.39985687063426,4.50785196366098));
#12889=CARTESIAN_POINT('Ctrl Pts',(3.43366207255012,2.4000380247868,4.52714803633902));
#12890=CARTESIAN_POINT('Ctrl Pts',(3.43372360717887,2.36989468640869,4.52915624308993));
#12891=CARTESIAN_POINT('Ctrl Pts',(3.44154516635149,2.33972158979514,4.53116444984084));
#12892=CARTESIAN_POINT('Ctrl Pts',(3.45693460375181,2.31409281443648,4.53317265659175));
#12893=CARTESIAN_POINT('Ctrl Pts',(3.48532393848085,2.26681468051736,4.53687725294402));
#12894=CARTESIAN_POINT('Ctrl Pts',(3.53946694042407,2.23500097847622,4.54058184929629));
#12895=CARTESIAN_POINT('Ctrl Pts',(3.59458475774056,2.23321142940033,4.54428644564855));
#12896=CARTESIAN_POINT('Ctrl Pts',(3.64970257505705,2.23142188032444,4.54799104200082));
#12897=CARTESIAN_POINT('Ctrl Pts',(3.7057952077468,2.25965648421381,4.55169563835309));
#12898=CARTESIAN_POINT('Ctrl Pts',(3.73719154438744,2.30499351452124,4.55540023470536));
#12899=CARTESIAN_POINT('Ctrl Pts',(3.76858788102808,2.35033054482868,4.55910483105763));
#12900=CARTESIAN_POINT('Ctrl Pts',(3.77528792161962,2.41277000155418,4.56280942740989));
#12901=CARTESIAN_POINT('Ctrl Pts',(3.75422535459604,2.4637361132596,4.56651402376216));
#12902=CARTESIAN_POINT('Ctrl Pts',(3.73316278757246,2.51470222496502,4.57021862011443));
#12903=CARTESIAN_POINT('Ctrl Pts',(3.68433761293377,2.55419499165036,4.5739232164667));
#12904=CARTESIAN_POINT('Ctrl Pts',(3.63009494870967,2.56414032470881,4.57762781281897));
#12905=CARTESIAN_POINT('Ctrl Pts',(3.57585228448556,2.57408565776726,4.58133240917124));
#12906=CARTESIAN_POINT('Ctrl Pts',(3.51619213067606,2.55448355719882,4.5850370055235));
#12907=CARTESIAN_POINT('Ctrl Pts',(3.47841829496877,2.51430503547713,4.58874160187577));
#12908=CARTESIAN_POINT('Ctrl Pts',(3.44984628656769,2.48391413027303,4.59154374669685));
#12909=CARTESIAN_POINT('Ctrl Pts',(3.43379623122065,2.44175071136891,4.59434589151794));
#12910=CARTESIAN_POINT('Ctrl Pts',(3.43341474631901,2.39984765669014,4.59714803633902));
#12911=CARTESIAN_POINT('Origin',(3.6,2.4,4.7));
#12912=CARTESIAN_POINT('',(3.43314571939013,2.4000550352968,4.66714803633902));
#12913=CARTESIAN_POINT('',(3.43350338992805,2.40014270746267,4.64785196366098));
#12914=CARTESIAN_POINT('',(3.4334,2.4,4.7));
#12915=CARTESIAN_POINT('Ctrl Pts',(3.43350338992805,2.40014270746267,4.64785196366098));
#12916=CARTESIAN_POINT('Ctrl Pts',(3.43336795942281,2.41673658085083,4.64674379602763));
#12917=CARTESIAN_POINT('Ctrl Pts',(3.43564861639563,2.43329406542932,4.64563562839428));
#12918=CARTESIAN_POINT('Ctrl Pts',(3.44049847652216,2.44906128539828,4.64452746076093));
#12919=CARTESIAN_POINT('Ctrl Pts',(3.45671152371201,2.5017709872742,4.64082286440866));
#12920=CARTESIAN_POINT('Ctrl Pts',(3.5016369588364,2.54564900761994,4.63711826805639));
#12921=CARTESIAN_POINT('Ctrl Pts',(3.55471440176584,2.56061432161925,4.63341367170412));
#12922=CARTESIAN_POINT('Ctrl Pts',(3.60779184469527,2.57557963561855,4.62970907535186));
#12923=CARTESIAN_POINT('Ctrl Pts',(3.66902129542974,2.56163224327142,4.62600447899959));
#12924=CARTESIAN_POINT('Ctrl Pts',(3.71038074864658,2.52515524777208,4.62229988264732));
#12925=CARTESIAN_POINT('Ctrl Pts',(3.75174020186341,2.48867825227274,4.61859528629505));
#12926=CARTESIAN_POINT('Ctrl Pts',(3.77322965756262,2.42967165362121,4.61489068994278));
#12927=CARTESIAN_POINT('Ctrl Pts',(3.76501434448883,2.37514015628156,4.61118609359052));
#12928=CARTESIAN_POINT('Ctrl Pts',(3.75679903141505,2.32060865894192,4.60748149723825));
#12929=CARTESIAN_POINT('Ctrl Pts',(3.71887894956827,2.27055226291416,4.60377690088598));
#12930=CARTESIAN_POINT('Ctrl Pts',(3.6686084394294,2.24787956167738,4.60007230453371));
#12931=CARTESIAN_POINT('Ctrl Pts',(3.61833792929053,2.22520686044059,4.59636770818145));
#12932=CARTESIAN_POINT('Ctrl Pts',(3.55571699085956,2.22991785399477,4.59266311182918));
#12933=CARTESIAN_POINT('Ctrl Pts',(3.50940445168984,2.2598565294309,4.58895851547691));
#12934=CARTESIAN_POINT('Ctrl Pts',(3.46312207100161,2.28977570895933,4.58525633153827));
#12935=CARTESIAN_POINT('Ctrl Pts',(3.43312685660295,2.34488972480058,4.58155414759962));
#12936=CARTESIAN_POINT('Ctrl Pts',(3.43312356496403,2.40000067111703,4.57785196366098));
#12937=CARTESIAN_POINT('Ctrl Pts',(3.43341474631901,2.39984765669014,4.59714803633902));
#12938=CARTESIAN_POINT('Ctrl Pts',(3.43329188627587,2.38635246701557,4.59805048787021));
#12939=CARTESIAN_POINT('Ctrl Pts',(3.43479418574107,2.37288428257405,4.59895293940139));
#12940=CARTESIAN_POINT('Ctrl Pts',(3.43802675467359,2.35984505096448,4.59985539093258));
#12941=CARTESIAN_POINT('Ctrl Pts',(3.45129656769075,2.30631853104845,4.60355998728484));
#12942=CARTESIAN_POINT('Ctrl Pts',(3.49372371133013,2.26002043409134,4.60726458363711));
#12943=CARTESIAN_POINT('Ctrl Pts',(3.54589116272705,2.24213934669288,4.61096917998938));
#12944=CARTESIAN_POINT('Ctrl Pts',(3.59805861412397,2.22425825929442,4.61467377634164));
#12945=CARTESIAN_POINT('Ctrl Pts',(3.65996637327845,2.23479418145462,4.61837837269391));
#12946=CARTESIAN_POINT('Ctrl Pts',(3.70328200317247,2.26892528865449,4.62208296904618));
#12947=CARTESIAN_POINT('Ctrl Pts',(3.7465976330665,2.30305639585435,4.62578756539845));
#12948=CARTESIAN_POINT('Ctrl Pts',(3.77132113370008,2.3607826880939,4.62949216175072));
#12949=CARTESIAN_POINT('Ctrl Pts',(3.76613765481651,2.41568540039916,4.63319675810299));
#12950=CARTESIAN_POINT('Ctrl Pts',(3.76095417593294,2.47058811270442,4.63690135445526));
#12951=CARTESIAN_POINT('Ctrl Pts',(3.72586371753223,2.5226672450754,4.64060595080753));
#12952=CARTESIAN_POINT('Ctrl Pts',(3.67692562687786,2.54808848727385,4.64431054715979));
#12953=CARTESIAN_POINT('Ctrl Pts',(3.6279875362235,2.5735097294723,4.64801514351206));
#12954=CARTESIAN_POINT('Ctrl Pts',(3.56520181331549,2.57227308149821,4.65171973986433));
#12955=CARTESIAN_POINT('Ctrl Pts',(3.51730270026196,2.54494450230916,4.65542433621659));
#12956=CARTESIAN_POINT('Ctrl Pts',(3.46940358720842,2.51761592312011,4.65912893256886));
#12957=CARTESIAN_POINT('Ctrl Pts',(3.43639108400936,2.46419541271609,4.66283352892113));
#12958=CARTESIAN_POINT('Ctrl Pts',(3.43337354994745,2.40913117059842,4.6665381252734));
#12959=CARTESIAN_POINT('Ctrl Pts',(3.43320795139183,2.40610931275893,4.66674142896194));
#12960=CARTESIAN_POINT('Ctrl Pts',(3.43313268806444,2.40308250452664,4.66694473265048));
#12961=CARTESIAN_POINT('Ctrl Pts',(3.43314571939013,2.4000550352968,4.66714803633902));
#12962=CARTESIAN_POINT('Origin',(3.6,2.4,4.7));
#12963=CARTESIAN_POINT('',(3.43357722762007,2.40011764662452,4.73714803633902));
#12964=CARTESIAN_POINT('',(3.43362781118013,2.39991574862771,4.71785196366098));
#12965=CARTESIAN_POINT('',(3.4334,2.4,4.7));
#12966=CARTESIAN_POINT('Ctrl Pts',(3.43362781118013,2.39991574862771,4.71785196366098));
#12967=CARTESIAN_POINT('Ctrl Pts',(3.4337799165104,2.43312978761853,4.71563804080791));
#12968=CARTESIAN_POINT('Ctrl Pts',(3.44340626416077,2.46642503117871,4.71342411795483));
#12969=CARTESIAN_POINT('Ctrl Pts',(3.46191047388993,2.49369647002616,4.71121019510175));
#12970=CARTESIAN_POINT('Ctrl Pts',(3.49287389602047,2.5393302520412,4.70750559874949));
#12971=CARTESIAN_POINT('Ctrl Pts',(3.54869526280824,2.56809742778931,4.70380100239722));
#12972=CARTESIAN_POINT('Ctrl Pts',(3.60382760921412,2.56683253616837,4.70009640604495));
#12973=CARTESIAN_POINT('Ctrl Pts',(3.65895995562,2.56556764454744,4.69639180969268));
#12974=CARTESIAN_POINT('Ctrl Pts',(3.71340328164399,2.53427068555747,4.69268721334041));
#12975=CARTESIAN_POINT('Ctrl Pts',(3.74224129041658,2.48726488994604,4.68898261698815));
#12976=CARTESIAN_POINT('Ctrl Pts',(3.77107929918916,2.44025909433461,4.68527802063588));
#12977=CARTESIAN_POINT('Ctrl Pts',(3.77431199071034,2.37754446210172,4.68157342428361));
#12978=CARTESIAN_POINT('Ctrl Pts',(3.75045990537481,2.32782270030492,4.67786882793134));
#12979=CARTESIAN_POINT('Ctrl Pts',(3.72660782003928,2.27810093850813,4.67416423157907));
#12980=CARTESIAN_POINT('Ctrl Pts',(3.67567095784705,2.24137204714742,4.6704596352268));
#12981=CARTESIAN_POINT('Ctrl Pts',(3.62096086261208,2.23444521162098,4.66675503887454));
#12982=CARTESIAN_POINT('Ctrl Pts',(3.56625076737711,2.22751837609454,4.66305044252227));
#12983=CARTESIAN_POINT('Ctrl Pts',(3.5077674390994,2.25039359640236,4.65934584617));
#12984=CARTESIAN_POINT('Ctrl Pts',(3.4722761045882,2.29260189825932,4.65564124981774));
#12985=CARTESIAN_POINT('Ctrl Pts',(3.44740140531328,2.32218429717603,4.65304482109882));
#12986=CARTESIAN_POINT('Ctrl Pts',(3.43382070261849,2.36126338259659,4.6504483923799));
#12987=CARTESIAN_POINT('Ctrl Pts',(3.43350338992805,2.40014270746267,4.64785196366098));
#12988=CARTESIAN_POINT('Ctrl Pts',(3.43314571939013,2.4000550352968,4.66714803633902));
#12989=CARTESIAN_POINT('Ctrl Pts',(3.43337014465933,2.34791601174949,4.67064932900275));
#12990=CARTESIAN_POINT('Ctrl Pts',(3.45978247246013,2.29558093851357,4.67415062166648));
#12991=CARTESIAN_POINT('Ctrl Pts',(3.50195947903851,2.26495997488444,4.67765191433021));
#12992=CARTESIAN_POINT('Ctrl Pts',(3.54658550711625,2.23256099511944,4.68135651068247));
#12993=CARTESIAN_POINT('Ctrl Pts',(3.60886012819649,2.22447100942077,4.68506110703474));
#12994=CARTESIAN_POINT('Ctrl Pts',(3.66028300882075,2.24439244561677,4.68876570338701));
#12995=CARTESIAN_POINT('Ctrl Pts',(3.71170588944501,2.26431388181277,4.69247029973928));
#12996=CARTESIAN_POINT('Ctrl Pts',(3.75227702961328,2.31224673990343,4.69617489609154));
#12997=CARTESIAN_POINT('Ctrl Pts',(3.76342881697354,2.36625427558577,4.69987949244381));
#12998=CARTESIAN_POINT('Ctrl Pts',(3.7745806043338,2.42026181126811,4.70358408879608));
#12999=CARTESIAN_POINT('Ctrl Pts',(3.75631303888606,2.48034402454213,4.70728868514835));
#13000=CARTESIAN_POINT('Ctrl Pts',(3.71698637554161,2.51900394981365,4.71099328150062));
#13001=CARTESIAN_POINT('Ctrl Pts',(3.67765971219715,2.55766387508518,4.71469787785288));
#13002=CARTESIAN_POINT('Ctrl Pts',(3.617273950956,2.57490151235421,4.71840247420515));
#13003=CARTESIAN_POINT('Ctrl Pts',(3.5634649778607,2.56282795918052,4.72210707055742));
#13004=CARTESIAN_POINT('Ctrl Pts',(3.50965600476541,2.55075440600683,4.72581166690969));
#13005=CARTESIAN_POINT('Ctrl Pts',(3.46242381981598,2.50936966239043,4.72951626326196));
#13006=CARTESIAN_POINT('Ctrl Pts',(3.44338450027923,2.45761369091481,4.73322085961423));
#13007=CARTESIAN_POINT('Ctrl Pts',(3.43665675223952,2.43932516253718,4.73452991852249));
#13008=CARTESIAN_POINT('Ctrl Pts',(3.43344927286167,2.41974164310833,4.73583897743076));
#13009=CARTESIAN_POINT('Ctrl Pts',(3.43357722762007,2.40011764662452,4.73714803633902));
#13010=CARTESIAN_POINT('Origin',(3.6,2.4,4.7));
#13011=CARTESIAN_POINT('',(3.4335708769619,2.39987935507417,4.80714803633902));
#13012=CARTESIAN_POINT('',(3.43319592025803,2.39990252619761,4.78785196366098));
#13013=CARTESIAN_POINT('',(3.4334,2.4,4.7));
#13014=CARTESIAN_POINT('Ctrl Pts',(3.43319592025803,2.39990252619761,4.78785196366098));
#13015=CARTESIAN_POINT('Ctrl Pts',(3.43353981667182,2.44937640878962,4.78453228558818));
#13016=CARTESIAN_POINT('Ctrl Pts',(3.45695303934336,2.49913297337583,4.78121260751538));
#13017=CARTESIAN_POINT('Ctrl Pts',(3.495475201044,2.5300857875399,4.77789292944258));
#13018=CARTESIAN_POINT('Ctrl Pts',(3.5384640260409,2.56462759548935,4.77418833309031));
#13019=CARTESIAN_POINT('Ctrl Pts',(3.60026870000874,2.57575223778946,4.77048373673805));
#13020=CARTESIAN_POINT('Ctrl Pts',(3.6526039634498,2.55836845881058,4.76677914038578));
#13021=CARTESIAN_POINT('Ctrl Pts',(3.70493922689085,2.54098467983171,4.76307454403351));
#13022=CARTESIAN_POINT('Ctrl Pts',(3.74780507980512,2.49509247957384,4.75936994768124));
#13023=CARTESIAN_POINT('Ctrl Pts',(3.76158372154047,2.44169468371147,4.75566535132897));
#13024=CARTESIAN_POINT('Ctrl Pts',(3.77536236327582,2.38829688784909,4.7519607549767));
#13025=CARTESIAN_POINT('Ctrl Pts',(3.76005379383226,2.32739349638222,4.74825615862444));
#13026=CARTESIAN_POINT('Ctrl Pts',(3.72266406682112,2.28685729176137,4.74455156227217));
#13027=CARTESIAN_POINT('Ctrl Pts',(3.68527433980998,2.24632108714052,4.7408469659199));
#13028=CARTESIAN_POINT('Ctrl Pts',(3.62580345523126,2.22615206936571,4.73714236956763));
#13029=CARTESIAN_POINT('Ctrl Pts',(3.57146860063526,2.23558070378767,4.73343777321536));
#13030=CARTESIAN_POINT('Ctrl Pts',(3.51713374603927,2.24500933820964,4.72973317686309));
#13031=CARTESIAN_POINT('Ctrl Pts',(3.467934921426,2.28403562482839,4.72602858051083));
#13032=CARTESIAN_POINT('Ctrl Pts',(3.44638824785603,2.33479896227876,4.72232398415856));
#13033=CARTESIAN_POINT('Ctrl Pts',(3.43771819254303,2.35522536091232,4.72083331065937));
#13034=CARTESIAN_POINT('Ctrl Pts',(3.43352539596517,2.37755214744982,4.71934263716017));
#13035=CARTESIAN_POINT('Ctrl Pts',(3.43362781118013,2.39991574862771,4.71785196366098));
#13036=CARTESIAN_POINT('Ctrl Pts',(3.43357722762007,2.40011764662452,4.73714803633902));
#13037=CARTESIAN_POINT('Ctrl Pts',(3.4338113808831,2.36420633806453,4.73954357378302));
#13038=CARTESIAN_POINT('Ctrl Pts',(3.44521519316665,2.32815948046248,4.74193911122703));
#13039=CARTESIAN_POINT('Ctrl Pts',(3.46665596573275,2.29966495797107,4.74433464867103));
#13040=CARTESIAN_POINT('Ctrl Pts',(3.49981320484709,2.25559939583779,4.7480392450233));
#13041=CARTESIAN_POINT('Ctrl Pts',(3.55697413719987,2.22959547090607,4.75174384137556));
#13042=CARTESIAN_POINT('Ctrl Pts',(3.61197873797528,2.23355402687319,4.75544843772783));
#13043=CARTESIAN_POINT('Ctrl Pts',(3.6669833387507,2.2375125828403,4.7591530340801));
#13044=CARTESIAN_POINT('Ctrl Pts',(3.71983160794876,2.27143361970626,4.76285763043237));
#13045=CARTESIAN_POINT('Ctrl Pts',(3.74633723550091,2.31979298260399,4.76656222678464));
#13046=CARTESIAN_POINT('Ctrl Pts',(3.77284286305306,2.36815234550172,4.7702668231369));
#13047=CARTESIAN_POINT('Ctrl Pts',(3.77300584895929,2.43095003443123,4.77397141948917));
#13048=CARTESIAN_POINT('Ctrl Pts',(3.74675160179543,2.47944633096681,4.77767601584144));
#13049=CARTESIAN_POINT('Ctrl Pts',(3.72049735463157,2.52794262750239,4.78138061219371));
#13050=CARTESIAN_POINT('Ctrl Pts',(3.66782587439761,2.56213753164403,4.78508520854598));
#13051=CARTESIAN_POINT('Ctrl Pts',(3.61284256269023,2.56638155161303,4.78878980489825));
#13052=CARTESIAN_POINT('Ctrl Pts',(3.55785925098286,2.57062557158203,4.79249440125052));
#13053=CARTESIAN_POINT('Ctrl Pts',(3.50056410780207,2.54491870737838,4.79619899760278));
#13054=CARTESIAN_POINT('Ctrl Pts',(3.4671785803101,2.50102585117272,4.79990359395505));
#13055=CARTESIAN_POINT('Ctrl Pts',(3.44541646757448,2.47241461280706,4.80231840808304));
#13056=CARTESIAN_POINT('Ctrl Pts',(3.43381352470784,2.43607616609189,4.80473322221103));
#13057=CARTESIAN_POINT('Ctrl Pts',(3.4335708769619,2.39987935507417,4.80714803633902));
#13058=CARTESIAN_POINT('Origin',(3.6,2.4,4.7));
#13059=CARTESIAN_POINT('',(3.43314188794433,2.3999499425809,4.87714803633902));
#13060=CARTESIAN_POINT('',(3.43333250203974,2.40014587505553,4.85785196366098));
#13061=CARTESIAN_POINT('',(3.4334,2.4,4.7));
#13062=CARTESIAN_POINT('Ctrl Pts',(3.43333250203974,2.40014587505553,4.85785196366098));
#13063=CARTESIAN_POINT('Ctrl Pts',(3.43323383740233,2.41091157669441,4.85713112672073));
#13064=CARTESIAN_POINT('Ctrl Pts',(3.43418764294185,2.42165986991066,4.85641028978047));
#13065=CARTESIAN_POINT('Ctrl Pts',(3.43625743346387,2.43218878097762,4.85568945284021));
#13066=CARTESIAN_POINT('Ctrl Pts',(3.44689470520955,2.48629999996998,4.85198485648794));
#13067=CARTESIAN_POINT('Ctrl Pts',(3.48700780884227,2.53461681182183,4.84828026013567));
#13068=CARTESIAN_POINT('Ctrl Pts',(3.53823875502779,2.55502675361418,4.8445756637834));
#13069=CARTESIAN_POINT('Ctrl Pts',(3.58946970121331,2.57543669540653,4.84087106743113));
#13070=CARTESIAN_POINT('Ctrl Pts',(3.65181848995162,2.56793976713939,4.83716647107887));
#13071=CARTESIAN_POINT('Ctrl Pts',(3.69675084453495,2.5359669805447,4.8334618747266));
#13072=CARTESIAN_POINT('Ctrl Pts',(3.74168319911827,2.50399419395,4.82975727837433));
#13073=CARTESIAN_POINT('Ctrl Pts',(3.7691991195466,2.44754554902777,4.82605268202206));
#13074=CARTESIAN_POINT('Ctrl Pts',(3.76670578881005,2.39245508821223,4.8223480856698));
#13075=CARTESIAN_POINT('Ctrl Pts',(3.7642124580735,2.33736462739668,4.81864348931753));
#13076=CARTESIAN_POINT('Ctrl Pts',(3.73170987617206,2.28363235068783,4.81493889296526));
#13077=CARTESIAN_POINT('Ctrl Pts',(3.68407303401509,2.25584913920422,4.811234296613));
#13078=CARTESIAN_POINT('Ctrl Pts',(3.63643619185813,2.2280659277206,4.80752970026073));
#13079=CARTESIAN_POINT('Ctrl Pts',(3.57366508944564,2.22623178146222,4.80382510390846));
#13080=CARTESIAN_POINT('Ctrl Pts',(3.52448727773306,2.25118610786454,4.80012050755619));
#13081=CARTESIAN_POINT('Ctrl Pts',(3.47530946602049,2.27614043426686,4.79641591120392));
#13082=CARTESIAN_POINT('Ctrl Pts',(3.43972494500783,2.32788323332987,4.79271131485165));
#13083=CARTESIAN_POINT('Ctrl Pts',(3.43401917251448,2.38273411966077,4.78900671849938));
#13084=CARTESIAN_POINT('Ctrl Pts',(3.43342632624397,2.38843328545001,4.78862180021992));
#13085=CARTESIAN_POINT('Ctrl Pts',(3.43315604530238,2.39416600556269,4.78823688194045));
#13086=CARTESIAN_POINT('Ctrl Pts',(3.43319592025803,2.39990252619761,4.78785196366098));
#13087=CARTESIAN_POINT('Ctrl Pts',(3.4335708769619,2.39987935507417,4.80714803633902));
#13088=CARTESIAN_POINT('Ctrl Pts',(3.43344127578645,2.38054618864739,4.8084378185633));
#13089=CARTESIAN_POINT('Ctrl Pts',(3.43655249507166,2.36125342749717,4.80972760078758));
#13090=CARTESIAN_POINT('Ctrl Pts',(3.44308754966948,2.34320004344294,4.81101738301185));
#13091=CARTESIAN_POINT('Ctrl Pts',(3.46185795832395,2.2913459401265,4.81472197936412));
#13092=CARTESIAN_POINT('Ctrl Pts',(3.50887468743604,2.24971658170129,4.81842657571639));
#13093=CARTESIAN_POINT('Ctrl Pts',(3.5626202643246,2.23736388010515,4.82213117206866));
#13094=CARTESIAN_POINT('Ctrl Pts',(3.61636584121316,2.22501117850901,4.82583576842092));
#13095=CARTESIAN_POINT('Ctrl Pts',(3.6768402658782,2.24193513374194,4.82954036477319));
#13096=CARTESIAN_POINT('Ctrl Pts',(3.71636707495845,2.28039040172619,4.83324496112546));
#13097=CARTESIAN_POINT('Ctrl Pts',(3.7558938840387,2.31884566971043,4.83694955747773));
#13098=CARTESIAN_POINT('Ctrl Pts',(3.77447307753417,2.378832250446,4.84065415383));
#13099=CARTESIAN_POINT('Ctrl Pts',(3.76360178219044,2.4328969451123,4.84435875018227));
#13100=CARTESIAN_POINT('Ctrl Pts',(3.75273048684672,2.4869616397786,4.84806334653454));
#13101=CARTESIAN_POINT('Ctrl Pts',(3.71240870266382,2.53510444837563,4.8517679428868));
#13102=CARTESIAN_POINT('Ctrl Pts',(3.66108992281312,2.55529254156049,4.85547253923907));
#13103=CARTESIAN_POINT('Ctrl Pts',(3.60977114296242,2.57548063474534,4.85917713559134));
#13104=CARTESIAN_POINT('Ctrl Pts',(3.54745536744392,2.56771401251802,4.86288173194361));
#13105=CARTESIAN_POINT('Ctrl Pts',(3.50266176427811,2.53554711358097,4.86658632829587));
#13106=CARTESIAN_POINT('Ctrl Pts',(3.46009329762648,2.50497811560107,4.87010689764359));
#13107=CARTESIAN_POINT('Ctrl Pts',(3.43334940270065,2.45237281292388,4.87362746699131));
#13108=CARTESIAN_POINT('Ctrl Pts',(3.43314188794433,2.3999499425809,4.87714803633902));
#13109=CARTESIAN_POINT('Origin',(3.6,2.4,4.7));
#13110=CARTESIAN_POINT('',(3.43342338863395,2.40015219044389,4.94714803633902));
#13111=CARTESIAN_POINT('',(3.4336698690944,2.40000633253548,4.92785196366098));
#13112=CARTESIAN_POINT('',(3.4334,2.4,4.7));
#13113=CARTESIAN_POINT('Ctrl Pts',(3.4336698690944,2.40000633253548,4.92785196366098));
#13114=CARTESIAN_POINT('Ctrl Pts',(3.43366057242126,2.42742681740845,4.926025371501));
#13115=CARTESIAN_POINT('Ctrl Pts',(3.44006468394764,2.45484321422969,4.92419877934102));
#13116=CARTESIAN_POINT('Ctrl Pts',(3.4529060499396,2.47881063108511,4.92237218718104));
#13117=CARTESIAN_POINT('Ctrl Pts',(3.47895022041959,2.52742006180595,4.91866759082877));
#13118=CARTESIAN_POINT('Ctrl Pts',(3.53147325119262,2.5618425345377,4.9149629944765));
#13119=CARTESIAN_POINT('Ctrl Pts',(3.58643767940152,2.56632440944362,4.91125839812423));
#13120=CARTESIAN_POINT('Ctrl Pts',(3.64140210761043,2.57080628434953,4.90755380177196));
#13121=CARTESIAN_POINT('Ctrl Pts',(3.6988079332552,2.54534756142961,4.90384920541969));
#13122=CARTESIAN_POINT('Ctrl Pts',(3.73238305471537,2.50159956959011,4.90014460906743));
#13123=CARTESIAN_POINT('Ctrl Pts',(3.76595817617555,2.45785157775061,4.89644001271516));
#13124=CARTESIAN_POINT('Ctrl Pts',(3.77570259345112,2.39581431699153,4.89273541636289));
#13125=CARTESIAN_POINT('Ctrl Pts',(3.75715671872181,2.34387949147388,4.88903082001062));
#13126=CARTESIAN_POINT('Ctrl Pts',(3.7386108439925,2.29194466595622,4.88532622365836));
#13127=CARTESIAN_POINT('Ctrl Pts',(3.6917746772583,2.25011227567998,4.88162162730609));
#13128=CARTESIAN_POINT('Ctrl Pts',(3.638083055804,2.23752715126117,4.87791703095382));
#13129=CARTESIAN_POINT('Ctrl Pts',(3.58439143434971,2.22494202684235,4.87421243460155));
#13130=CARTESIAN_POINT('Ctrl Pts',(3.52384435817533,2.24160416828095,4.87050783824928));
#13131=CARTESIAN_POINT('Ctrl Pts',(3.48415154001745,2.27988805206668,4.86680324189701));
#13132=CARTESIAN_POINT('Ctrl Pts',(3.45218211379499,2.3107226930672,4.863819482485));
#13133=CARTESIAN_POINT('Ctrl Pts',(3.43374090444541,2.35558342022287,4.86083572307299));
#13134=CARTESIAN_POINT('Ctrl Pts',(3.43333250203974,2.40014587505553,4.85785196366098));
#13135=CARTESIAN_POINT('Ctrl Pts',(3.43314188794433,2.3999499425809,4.87714803633902));
#13136=CARTESIAN_POINT('Ctrl Pts',(3.43313104074456,2.39720969722669,4.87733206334358));
#13137=CARTESIAN_POINT('Ctrl Pts',(3.43319270038641,2.39446995034259,4.87751609034813));
#13138=CARTESIAN_POINT('Ctrl Pts',(3.43332839678999,2.39173387533235,4.87770011735268));
#13139=CARTESIAN_POINT('Ctrl Pts',(3.43606006328079,2.33665471166754,4.88140471370495));
#13140=CARTESIAN_POINT('Ctrl Pts',(3.4687948270755,2.28306355998471,4.88510931005722));
#13141=CARTESIAN_POINT('Ctrl Pts',(3.5165514379046,2.2554867147355,4.88881390640948));
#13142=CARTESIAN_POINT('Ctrl Pts',(3.5643080487337,2.2279098694863,4.89251850276175));
#13143=CARTESIAN_POINT('Ctrl Pts',(3.6270865065972,2.22634733067072,4.89622309911402));
#13144=CARTESIAN_POINT('Ctrl Pts',(3.67615589427605,2.25151420303488,4.89992769546629));
#13145=CARTESIAN_POINT('Ctrl Pts',(3.72522528195491,2.27668107539905,4.90363229181856));
#13146=CARTESIAN_POINT('Ctrl Pts',(3.76058559944912,2.32857735894297,4.90733688817082));
#13147=CARTESIAN_POINT('Ctrl Pts',(3.76605399695032,2.38345242523688,4.91104148452309));
#13148=CARTESIAN_POINT('Ctrl Pts',(3.77152239445151,2.43832749153079,4.91474608087536));
#13149=CARTESIAN_POINT('Ctrl Pts',(3.74709887195967,2.4961813405747,4.91845067722763));
#13150=CARTESIAN_POINT('Ctrl Pts',(3.70396099303503,2.53053683028788,4.9221552735799));
#13151=CARTESIAN_POINT('Ctrl Pts',(3.66082311411038,2.56489232000106,4.92585986993216));
#13152=CARTESIAN_POINT('Ctrl Pts',(3.59897087875293,2.57574945038351,4.92956446628443));
#13153=CARTESIAN_POINT('Ctrl Pts',(3.54671131319796,2.55813939417591,4.9332690626367));
#13154=CARTESIAN_POINT('Ctrl Pts',(3.494451747643,2.5405293379683,4.93697365898897));
#13155=CARTESIAN_POINT('Ctrl Pts',(3.45178485189053,2.49445209517064,4.94067825534124));
#13156=CARTESIAN_POINT('Ctrl Pts',(3.43823737272355,2.44099517717631,4.94438285169351));
#13157=CARTESIAN_POINT('Ctrl Pts',(3.43486666978988,2.42769474038747,4.94530457990868));
#13158=CARTESIAN_POINT('Ctrl Pts',(3.43329859706143,2.41393746665015,4.94622630812385));
#13159=CARTESIAN_POINT('Ctrl Pts',(3.43342338863395,2.40015219044389,4.94714803633902));
#13160=CARTESIAN_POINT('Origin',(3.6,2.4,4.7));
#13161=CARTESIAN_POINT('',(3.43365998372879,2.39995738785189,5.01714803633902));
#13162=CARTESIAN_POINT('',(3.43335574706359,2.39985083704977,4.99785196366098));
#13163=CARTESIAN_POINT('',(3.4334,2.4,4.7));
#13164=CARTESIAN_POINT('Ctrl Pts',(3.43335574706359,2.39985083704977,4.99785196366098));
#13165=CARTESIAN_POINT('Ctrl Pts',(3.43376006251615,2.44366117078388,4.99491961628127));
#13166=CARTESIAN_POINT('Ctrl Pts',(3.45150379085869,2.48776127159334,4.99198726890157));
#13167=CARTESIAN_POINT('Ctrl Pts',(3.48249984106631,2.5184966596533,4.98905492152186));
#13168=CARTESIAN_POINT('Ctrl Pts',(3.52165886271855,2.55732637242214,4.98535032516959));
#13169=CARTESIAN_POINT('Ctrl Pts',(3.58196946998821,2.57482511625956,4.98164572881732));
#13170=CARTESIAN_POINT('Ctrl Pts',(3.63583017159909,2.56298449167174,4.97794113246505));
#13171=CARTESIAN_POINT('Ctrl Pts',(3.68969087320997,2.55114386708391,4.97423653611278));
#13172=CARTESIAN_POINT('Ctrl Pts',(3.73710166916209,2.50996387407084,4.97053193976052));
#13173=CARTESIAN_POINT('Ctrl Pts',(3.75636473978792,2.45829077001732,4.96682734340825));
#13174=CARTESIAN_POINT('Ctrl Pts',(3.77562781041376,2.4066176659638,4.96312274705598));
#13175=CARTESIAN_POINT('Ctrl Pts',(3.76674315571332,2.34445145086982,4.95941815070371));
#13176=CARTESIAN_POINT('Ctrl Pts',(3.73377688832091,2.30024284554165,4.95571355435145));
#13177=CARTESIAN_POINT('Ctrl Pts',(3.70081062092849,2.25603424021347,4.95200895799918));
#13178=CARTESIAN_POINT('Ctrl Pts',(3.64376274084411,2.2297832446511,4.94830436164691));
#13179=CARTESIAN_POINT('Ctrl Pts',(3.58874153385625,2.23350377584586,4.94459976529464));
#13180=CARTESIAN_POINT('Ctrl Pts',(3.5337203268684,2.23722430704061,4.94089516894238));
#13181=CARTESIAN_POINT('Ctrl Pts',(3.48072579297707,2.2709163649925,4.93719057259011));
#13182=CARTESIAN_POINT('Ctrl Pts',(3.45401118112487,2.31916058832341,4.93348597623784));
#13183=CARTESIAN_POINT('Ctrl Pts',(3.44046850379027,2.34361746433734,4.93160797204555));
#13184=CARTESIAN_POINT('Ctrl Pts',(3.43367942743562,2.37181405914562,4.92972996785326));
#13185=CARTESIAN_POINT('Ctrl Pts',(3.4336698690944,2.40000633253548,4.92785196366098));
#13186=CARTESIAN_POINT('Ctrl Pts',(3.43342338863395,2.40015219044389,4.94714803633902));
#13187=CARTESIAN_POINT('Ctrl Pts',(3.43380015749623,2.35853188927053,4.94993090447612));
#13188=CARTESIAN_POINT('Ctrl Pts',(3.44960819526551,2.31665633218087,4.95271377261321));
#13189=CARTESIAN_POINT('Ctrl Pts',(3.47782659951237,2.28632760954166,4.95549664075031));
#13190=CARTESIAN_POINT('Ctrl Pts',(3.51539136804964,2.24595355309232,4.95920123710258));
#13191=CARTESIAN_POINT('Ctrl Pts',(3.57494896770565,2.22604203338462,4.96290583345485));
#13192=CARTESIAN_POINT('Ctrl Pts',(3.62924252529985,2.23570567012353,4.96661042980711));
#13193=CARTESIAN_POINT('Ctrl Pts',(3.68353608289404,2.24536930686244,4.97031502615938));
#13194=CARTESIAN_POINT('Ctrl Pts',(3.73256559842641,2.28460810004796,4.97401962251165));
#13195=CARTESIAN_POINT('Ctrl Pts',(3.75389243606413,2.33546419387067,4.97772421886392));
#13196=CARTESIAN_POINT('Ctrl Pts',(3.77521927370186,2.38632028769338,4.98142881521618));
#13197=CARTESIAN_POINT('Ctrl Pts',(3.76884343344493,2.44879368215328,4.98513341156845));
#13198=CARTESIAN_POINT('Ctrl Pts',(3.73768285480685,2.49429307324449,4.98883800792072));
#13199=CARTESIAN_POINT('Ctrl Pts',(3.70652227616876,2.5397924643357,4.99254260427299));
#13200=CARTESIAN_POINT('Ctrl Pts',(3.65057695914952,2.5683178520582,4.99624720062526));
#13201=CARTESIAN_POINT('Ctrl Pts',(3.59545059518146,2.56681443253905,4.99995179697753));
#13202=CARTESIAN_POINT('Ctrl Pts',(3.54032423121339,2.5653110130199,5.00365639332979));
#13203=CARTESIAN_POINT('Ctrl Pts',(3.4860168202965,2.5337787862591,5.00736098968206));
#13204=CARTESIAN_POINT('Ctrl Pts',(3.45738245724731,2.48664865149311,5.01106558603433));
#13205=CARTESIAN_POINT('Ctrl Pts',(3.44171119613527,2.4608548649544,5.01309306946923));
#13206=CARTESIAN_POINT('Ctrl Pts',(3.43372965048622,2.43038911757193,5.01512055290412));
#13207=CARTESIAN_POINT('Ctrl Pts',(3.43365998372879,2.39995738785189,5.01714803633902));
#13208=CARTESIAN_POINT('Origin',(3.6,2.4,4.7));
#13209=CARTESIAN_POINT('',(3.43326717741735,2.39986996798437,5.08714803633902));
#13210=CARTESIAN_POINT('',(3.43317938608394,2.40008640134203,5.06785196366098));
#13211=CARTESIAN_POINT('',(3.4334,2.4,4.7));
#13212=CARTESIAN_POINT('Ctrl Pts',(3.43317938608394,2.40008640134203,5.06785196366098));
#13213=CARTESIAN_POINT('Ctrl Pts',(3.43314802172115,2.40505542046622,5.06751845741382));
#13214=CARTESIAN_POINT('Ctrl Pts',(3.4333507965104,2.41002184414099,5.06718495116665));
#13215=CARTESIAN_POINT('Ctrl Pts',(3.43379604919982,2.41496643290483,5.06685144491949));
#13216=CARTESIAN_POINT('Ctrl Pts',(3.4387419280344,2.46989105771691,5.06314684856722));
#13217=CARTESIAN_POINT('Ctrl Pts',(3.47360673324676,2.52212151084356,5.05944225221496));
#13218=CARTESIAN_POINT('Ctrl Pts',(3.52243437289015,2.54775424884904,5.05573765586269));
#13219=CARTESIAN_POINT('Ctrl Pts',(3.57126201253354,2.57338698685451,5.05203305951042));
#13220=CARTESIAN_POINT('Ctrl Pts',(3.63405248660798,2.57242200973882,5.04832846315815));
#13221=CARTESIAN_POINT('Ctrl Pts',(3.68206938667054,2.54530093495911,5.04462386680588));
#13222=CARTESIAN_POINT('Ctrl Pts',(3.7300862867331,2.51817986017941,5.04091927045361));
#13223=CARTESIAN_POINT('Ctrl Pts',(3.7633296127838,2.4649026877357,5.03721467410135));
#13224=CARTESIAN_POINT('Ctrl Pts',(3.76658536412569,2.40985202258946,5.03351007774908));
#13225=CARTESIAN_POINT('Ctrl Pts',(3.76984111546757,2.35480135744323,5.02980548139681));
#13226=CARTESIAN_POINT('Ctrl Pts',(3.74310929210064,2.29797719959448,5.02610088504454));
#13227=CARTESIAN_POINT('Ctrl Pts',(3.69862386658003,2.26538544465498,5.02239628869227));
#13228=CARTESIAN_POINT('Ctrl Pts',(3.65413844105941,2.23279368971548,5.01869169234));
#13229=CARTESIAN_POINT('Ctrl Pts',(3.59189941338511,2.22443433768522,5.01498709598774));
#13230=CARTESIAN_POINT('Ctrl Pts',(3.54039082648689,2.24413309464159,5.01128249963547));
#13231=CARTESIAN_POINT('Ctrl Pts',(3.48888223958867,2.26383185159795,5.0075779032832));
#13232=CARTESIAN_POINT('Ctrl Pts',(3.44810409346653,2.31158871754094,5.00387330693093));
#13233=CARTESIAN_POINT('Ctrl Pts',(3.43671873842288,2.36554749136257,5.00016871057866));
#13234=CARTESIAN_POINT('Ctrl Pts',(3.43434538167935,2.37679557446855,4.9993964616061));
#13235=CARTESIAN_POINT('Ctrl Pts',(3.43324926848095,2.38831315722103,4.99862421263354));
#13236=CARTESIAN_POINT('Ctrl Pts',(3.43335574706359,2.39985083704977,4.99785196366098));
#13237=CARTESIAN_POINT('Ctrl Pts',(3.43365998372879,2.39995738785189,5.01714803633902));
#13238=CARTESIAN_POINT('Ctrl Pts',(3.43360235612169,2.37478458193251,5.01882514925639));
#13239=CARTESIAN_POINT('Ctrl Pts',(3.43895837147105,2.34963505233992,5.02050226217376));
#13240=CARTESIAN_POINT('Ctrl Pts',(3.44985377385385,2.32717237393524,5.02217937509113));
#13241=CARTESIAN_POINT('Ctrl Pts',(3.47392076869108,2.2775542739145,5.0258839714434));
#13242=CARTESIAN_POINT('Ctrl Pts',(3.52501607354704,2.24104611664418,5.02958856779567));
#13243=CARTESIAN_POINT('Ctrl Pts',(3.57975563349286,2.23435605471958,5.03329316414794));
#13244=CARTESIAN_POINT('Ctrl Pts',(3.63449519343869,2.22766599279499,5.03699776050021));
#13245=CARTESIAN_POINT('Ctrl Pts',(3.69287900847437,2.25079402621613,5.04070235685247));
#13246=CARTESIAN_POINT('Ctrl Pts',(3.72818739245021,2.2931555045654,5.04440695320474));
#13247=CARTESIAN_POINT('Ctrl Pts',(3.76349577642604,2.33551698291468,5.04811154955701));
#13248=CARTESIAN_POINT('Ctrl Pts',(3.77572872934203,2.39711190619209,5.05181614590928));
#13249=CARTESIAN_POINT('Ctrl Pts',(3.75928777521595,2.44975095798197,5.05552074226155));
#13250=CARTESIAN_POINT('Ctrl Pts',(3.74284682108988,2.50239000977184,5.05922533861381));
#13251=CARTESIAN_POINT('Ctrl Pts',(3.69773195992176,2.54607319007419,5.06292993496608));
#13252=CARTESIAN_POINT('Ctrl Pts',(3.64459025516192,2.56080874487665,5.06663453131835));
#13253=CARTESIAN_POINT('Ctrl Pts',(3.59144855040209,2.57554429967911,5.07033912767062));
#13254=CARTESIAN_POINT('Ctrl Pts',(3.53028000205055,2.5613322289817,5.07404372402289));
#13255=CARTESIAN_POINT('Ctrl Pts',(3.48907876029587,2.52467656495583,5.07774832037516));
#13256=CARTESIAN_POINT('Ctrl Pts',(3.45423196161424,2.49367428224656,5.08088155902978));
#13257=CARTESIAN_POINT('Ctrl Pts',(3.43366833435756,2.44661747113372,5.0840147976844));
#13258=CARTESIAN_POINT('Ctrl Pts',(3.43326717741735,2.39986996798437,5.08714803633902));
#13259=CARTESIAN_POINT('Origin',(3.6,2.4,4.7));
#13260=CARTESIAN_POINT('',(3.43325215340634,2.40012157034435,5.15714803633902));
#13261=CARTESIAN_POINT('',(3.43361558566414,2.40009421455432,5.13785196366098));
#13262=CARTESIAN_POINT('',(3.4334,2.4,4.7));
#13263=CARTESIAN_POINT('',(3.72690708798524,2.50793586530485,5.2));
#13264=CARTESIAN_POINT('Ctrl Pts',(3.43325215340634,2.40012157034435,5.15714803633902));
#13265=CARTESIAN_POINT('Ctrl Pts',(3.43364568326786,2.35284438105766,5.16031823516921));
#13266=CARTESIAN_POINT('Ctrl Pts',(3.45475449837728,2.3052683699281,5.1634884339994));
#13267=CARTESIAN_POINT('Ctrl Pts',(3.49032381108024,2.27424021130156,5.16665863282959));
#13268=CARTESIAN_POINT('Ctrl Pts',(3.53188901034701,2.23798166430732,5.17036322918186));
#13269=CARTESIAN_POINT('Ctrl Pts',(3.59320079576331,2.22432009870508,5.17406782553412));
#13270=CARTESIAN_POINT('Ctrl Pts',(3.64619138280368,2.2396150803554,5.17777242188639));
#13271=CARTESIAN_POINT('Ctrl Pts',(3.69918196984405,2.25491006200572,5.18147701823866));
#13272=CARTESIAN_POINT('Ctrl Pts',(3.74385135850849,2.2991615909086,5.18518161459093));
#13273=CARTESIAN_POINT('Ctrl Pts',(3.75975544882264,2.35186813523316,5.1888862109432));
#13274=CARTESIAN_POINT('Ctrl Pts',(3.7756595391368,2.40457467955771,5.19259080729547));
#13275=CARTESIAN_POINT('Ctrl Pts',(3.76279833110066,2.46573623930395,5.19629540364773));
#13276=CARTESIAN_POINT('Ctrl Pts',(3.72690708798524,2.50793586530485,5.2));
#13277=CARTESIAN_POINT('',(3.47285246768952,2.50812032770478,5.2));
#13278=CARTESIAN_POINT('Origin',(3.6,2.4,5.2));
#13279=CARTESIAN_POINT('Ctrl Pts',(3.47285231527688,2.50812044463164,5.2));
#13280=CARTESIAN_POINT('Ctrl Pts',(3.50793811173714,2.54927258268021,5.19636770818145));
#13281=CARTESIAN_POINT('Ctrl Pts',(3.56493587106976,2.57187757629771,5.19273541636289));
#13282=CARTESIAN_POINT('Ctrl Pts',(3.6186762488644,2.56581789998251,5.18910312454433));
#13283=CARTESIAN_POINT('Ctrl Pts',(3.67348638458382,2.55963759952907,5.18539852819207));
#13284=CARTESIAN_POINT('Ctrl Pts',(3.72490816491496,2.52364007082416,5.1816939318398));
#13285=CARTESIAN_POINT('Ctrl Pts',(3.74944162746499,2.4742589593754,5.17798933548753));
#13286=CARTESIAN_POINT('Ctrl Pts',(3.77397509001502,2.42487784792664,5.17428473913527));
#13287=CARTESIAN_POINT('Ctrl Pts',(3.77162023478396,2.36211315373403,5.17058014278299));
#13288=CARTESIAN_POINT('Ctrl Pts',(3.74343805908691,2.31470980295916,5.16687554643072));
#13289=CARTESIAN_POINT('Ctrl Pts',(3.71525588338986,2.2673064521843,5.16317095007846));
#13290=CARTESIAN_POINT('Ctrl Pts',(3.66124638722683,2.23526444482719,5.15946635372619));
#13291=CARTESIAN_POINT('Ctrl Pts',(3.60613566997566,2.23323785031625,5.15576175737392));
#13292=CARTESIAN_POINT('Ctrl Pts',(3.55102495272448,2.23121125580531,5.15205716102166));
#13293=CARTESIAN_POINT('Ctrl Pts',(3.49481301438516,2.25920007414054,5.14835256466939));
#13294=CARTESIAN_POINT('Ctrl Pts',(3.46322139831185,2.30440012642267,5.14464796831712));
#13295=CARTESIAN_POINT('Ctrl Pts',(3.44390334496103,2.33203964380033,5.14238263343174));
#13296=CARTESIAN_POINT('Ctrl Pts',(3.43379141454156,2.36611485011022,5.14011729854636));
#13297=CARTESIAN_POINT('Ctrl Pts',(3.43361558566414,2.40009421455432,5.13785196366098));
#13298=CARTESIAN_POINT('Origin',(3.6,2.4,5.35459252805377));
#13299=CARTESIAN_POINT('',(3.39427731514299,2.4001195557093,4.34540747194623));
#13300=CARTESIAN_POINT('',(3.39483887138702,2.39991986985508,4.33959252805377));
#13301=CARTESIAN_POINT('',(3.394525,2.40000000000001,5.35459252805377));
#13302=CARTESIAN_POINT('',(3.78826275096636,2.31767678198967,4.3));
#13303=CARTESIAN_POINT('Ctrl Pts',(3.39483887138702,2.39991986985508,4.33959252805377));
#13304=CARTESIAN_POINT('Ctrl Pts',(3.39495667746176,2.43847992884438,4.33750880775932));
#13305=CARTESIAN_POINT('Ctrl Pts',(3.42394163903792,2.54576387140554,4.3317204911126));
#13306=CARTESIAN_POINT('Ctrl Pts',(3.59702533363695,2.64299053446886,4.32222757811361));
#13307=CARTESIAN_POINT('Ctrl Pts',(3.80250223745458,2.5338839434383,4.3111137890568));
#13308=CARTESIAN_POINT('Ctrl Pts',(3.81563717950601,2.38027862564402,4.30370459635227));
#13309=CARTESIAN_POINT('Ctrl Pts',(3.78826275096636,2.31767678198967,4.3));
#13310=CARTESIAN_POINT('',(3.72235838409899,2.2344646706273,4.3));
#13311=CARTESIAN_POINT('Origin',(3.6,2.4,4.3));
#13312=CARTESIAN_POINT('Ctrl Pts',(3.394277315143,2.4001195557093,4.34540747194623));
#13313=CARTESIAN_POINT('Ctrl Pts',(3.39422704674216,2.40728359221916,4.34501772883951));
#13314=CARTESIAN_POINT('Ctrl Pts',(3.39781627947545,2.48249299124839,4.34092338938053));
#13315=CARTESIAN_POINT('Ctrl Pts',(3.49037003538787,2.61673301642169,4.33312445356927));
#13316=CARTESIAN_POINT('Ctrl Pts',(3.72265542052987,2.60960761604941,4.32201066451248));
#13317=CARTESIAN_POINT('Ctrl Pts',(3.84179830935629,2.41200908789601,4.31096917998937));
#13318=CARTESIAN_POINT('Ctrl Pts',(3.77594284069862,2.27417970060314,4.30363229181856));
#13319=CARTESIAN_POINT('Ctrl Pts',(3.72235851517117,2.23446447326397,4.3));
#13320=CARTESIAN_POINT('Origin',(3.6,2.4,5.35459252805377));
#13321=CARTESIAN_POINT('',(3.39480734911062,2.40010265425899,4.41540747194623));
#13322=CARTESIAN_POINT('',(3.39433274005607,2.39985021891194,4.40959252805377));
#13323=CARTESIAN_POINT('',(3.394525,2.40000000000001,5.35459252805377));
#13324=CARTESIAN_POINT('Ctrl Pts',(3.39433274005607,2.39985021891194,4.40959252805377));
#13325=CARTESIAN_POINT('Ctrl Pts',(3.39481384314024,2.45851949137253,4.40640305253959));
#13326=CARTESIAN_POINT('Ctrl Pts',(3.45186169840294,2.58615034863243,4.39950898067315));
#13327=CARTESIAN_POINT('Ctrl Pts',(3.66843098640644,2.63302756431036,4.38891031245443));
#13328=CARTESIAN_POINT('Ctrl Pts',(3.83289206978718,2.4688824684104,4.37779652339763));
#13329=CARTESIAN_POINT('Ctrl Pts',(3.78418106902943,2.24170425860662,4.36668273434082));
#13330=CARTESIAN_POINT('Ctrl Pts',(3.56689371899776,2.15938431325527,4.35556894528402));
#13331=CARTESIAN_POINT('Ctrl Pts',(3.41495577575702,2.27149583748734,4.34653887652167));
#13332=CARTESIAN_POINT('Ctrl Pts',(3.39474723286599,2.36992492448255,4.34121340411158));
#13333=CARTESIAN_POINT('Ctrl Pts',(3.39483887138702,2.39991986985508,4.33959252805377));
#13334=CARTESIAN_POINT('Ctrl Pts',(3.39480734911062,2.40010265425899,4.41540747194623));
#13335=CARTESIAN_POINT('Ctrl Pts',(3.3946821849205,2.42777437678442,4.41391197361979));
#13336=CARTESIAN_POINT('Ctrl Pts',(3.41278383405305,2.52383658927861,4.40871187894108));
#13337=CARTESIAN_POINT('Ctrl Pts',(3.55878722266986,2.63934344974957,4.3998071879101));
#13338=CARTESIAN_POINT('Ctrl Pts',(3.77873475080197,2.56443107632444,4.38869339885329));
#13339=CARTESIAN_POINT('Ctrl Pts',(3.8350828706128,2.33901445723046,4.37757960979649));
#13340=CARTESIAN_POINT('Ctrl Pts',(3.67625990394949,2.16941582752504,4.36646582073968));
#13341=CARTESIAN_POINT('Ctrl Pts',(3.45564722223464,2.20942500090864,4.3557417747896));
#13342=CARTESIAN_POINT('Ctrl Pts',(3.394704859258,2.33918780536763,4.34872232519178));
#13343=CARTESIAN_POINT('Ctrl Pts',(3.394277315143,2.4001195557093,4.34540747194623));
#13344=CARTESIAN_POINT('Origin',(3.6,2.4,5.35459252805377));
#13345=CARTESIAN_POINT('',(3.39465010046741,2.39982347235041,4.48540747194623));
#13346=CARTESIAN_POINT('',(3.39437120031462,2.40016339024638,4.47959252805377));
#13347=CARTESIAN_POINT('',(3.394525,2.40000000000001,5.35459252805377));
#13348=CARTESIAN_POINT('Ctrl Pts',(3.39437120031462,2.40016339024638,4.47959252805377));
#13349=CARTESIAN_POINT('Ctrl Pts',(3.39427672852213,2.41103322262123,4.47900189367213));
#13350=CARTESIAN_POINT('Ctrl Pts',(3.40000383140382,2.48998144241434,4.47470666293823));
#13351=CARTESIAN_POINT('Ctrl Pts',(3.5022614856576,2.62233051762717,4.46670683585207));
#13352=CARTESIAN_POINT('Ctrl Pts',(3.73378446379617,2.60269537158839,4.45559304679526));
#13353=CARTESIAN_POINT('Ctrl Pts',(3.84285303079348,2.39753073097072,4.44447925773845));
#13354=CARTESIAN_POINT('Ctrl Pts',(3.72963541291671,2.19462648510256,4.43336546868165));
#13355=CARTESIAN_POINT('Ctrl Pts',(3.49776113486282,2.17970245626759,4.42225167962485));
#13356=CARTESIAN_POINT('Ctrl Pts',(3.39915518291127,2.31283529949844,4.41432736608222));
#13357=CARTESIAN_POINT('Ctrl Pts',(3.39425503880932,2.39037475353659,4.41010764889186));
#13358=CARTESIAN_POINT('Ctrl Pts',(3.39433274005607,2.39985021891194,4.40959252805377));
#13359=CARTESIAN_POINT('Ctrl Pts',(3.39465010046741,2.39982347235041,4.48540747194623));
#13360=CARTESIAN_POINT('Ctrl Pts',(3.39504368040953,2.44786270507631,4.48280621840007));
#13361=CARTESIAN_POINT('Ctrl Pts',(3.43581223293462,2.56491921556266,4.47650036850162));
#13362=CARTESIAN_POINT('Ctrl Pts',(3.63081864137997,2.64090222813732,4.46648992225093));
#13363=CARTESIAN_POINT('Ctrl Pts',(3.81910984841827,2.50475947107891,4.45537613319412));
#13364=CARTESIAN_POINT('Ctrl Pts',(3.80684730359907,2.27272920356226,4.44426234413732));
#13365=CARTESIAN_POINT('Ctrl Pts',(3.60525512148808,2.15719129638054,4.43314855508051));
#13366=CARTESIAN_POINT('Ctrl Pts',(3.42662677463403,2.24954018398722,4.42353026435015));
#13367=CARTESIAN_POINT('Ctrl Pts',(3.39499223729164,2.35922694980568,4.41761656997206));
#13368=CARTESIAN_POINT('Ctrl Pts',(3.39480734911062,2.40010265425899,4.41540747194623));
#13369=CARTESIAN_POINT('Origin',(3.6,2.4,5.35459252805377));
#13370=CARTESIAN_POINT('',(3.39418405900746,2.40000082772182,4.55540747194623));
#13371=CARTESIAN_POINT('',(3.39484822543359,2.40004689761745,4.54959252805377));
#13372=CARTESIAN_POINT('',(3.394525,2.40000000000001,5.35459252805377));
#13373=CARTESIAN_POINT('Ctrl Pts',(3.39484822543359,2.40004689761745,4.54959252805377));
#13374=CARTESIAN_POINT('Ctrl Pts',(3.3947841161748,2.43145144364515,4.54789613845241));
#13375=CARTESIAN_POINT('Ctrl Pts',(3.41632347620735,2.53135423912678,4.54249515249878));
#13376=CARTESIAN_POINT('Ctrl Pts',(3.57178887938318,2.64122151037363,4.5333895701929));
#13377=CARTESIAN_POINT('Ctrl Pts',(3.78736363324621,2.55452687009752,4.52227578113608));
#13378=CARTESIAN_POINT('Ctrl Pts',(3.83144232915068,2.3263920312721,4.51116199207928));
#13379=CARTESIAN_POINT('Ctrl Pts',(3.66367923564831,2.1656314047897,4.50004820302247));
#13380=CARTESIAN_POINT('Ctrl Pts',(3.44964305208187,2.21653398832958,4.48952504834731));
#13381=CARTESIAN_POINT('Ctrl Pts',(3.39486927759939,2.34285510326715,4.4827064900244));
#13382=CARTESIAN_POINT('Ctrl Pts',(3.39437120031462,2.40016339024638,4.47959252805377));
#13383=CARTESIAN_POINT('Ctrl Pts',(3.39418406069018,2.40000082771773,4.55540747194623));
#13384=CARTESIAN_POINT('Ctrl Pts',(3.39418405804479,2.40004511873352,4.55540505953261));
#13385=CARTESIAN_POINT('Ctrl Pts',(3.39420412805525,2.46810441674863,4.55169805076671));
#13386=CARTESIAN_POINT('Ctrl Pts',(3.46841582920963,2.6041305389052,4.54428644564855));
#13387=CARTESIAN_POINT('Ctrl Pts',(3.70013763173937,2.6212603119689,4.53317265659175));
#13388=CARTESIAN_POINT('Ctrl Pts',(3.84020232447629,2.43586801205837,4.52205886753494));
#13389=CARTESIAN_POINT('Ctrl Pts',(3.76040710518764,2.21764531427324,4.51094507847815));
#13390=CARTESIAN_POINT('Ctrl Pts',(3.53378944408678,2.16633392770918,4.49983128942133));
#13391=CARTESIAN_POINT('Ctrl Pts',(3.40663178603677,2.29085017634376,4.4913187539107));
#13392=CARTESIAN_POINT('Ctrl Pts',(3.39448316034026,2.37944724185309,4.48651081475233));
#13393=CARTESIAN_POINT('Ctrl Pts',(3.39465010046741,2.39982347235041,4.48540747194623));
#13394=CARTESIAN_POINT('Origin',(3.6,2.4,5.35459252805377));
#13395=CARTESIAN_POINT('',(3.3946525152789,2.40017600729827,4.62540747194623));
#13396=CARTESIAN_POINT('',(3.39454318727431,2.3998121083938,4.61959252805377));
#13397=CARTESIAN_POINT('',(3.394525,2.40000000000001,5.35459252805377));
#13398=CARTESIAN_POINT('Ctrl Pts',(3.39454318727431,2.3998121083938,4.61959252805377));
#13399=CARTESIAN_POINT('Ctrl Pts',(3.39501368913604,2.45149296169584,4.61679038323269));
#13400=CARTESIAN_POINT('Ctrl Pts',(3.44097934710978,2.57224452612634,4.61028364205933));
#13401=CARTESIAN_POINT('Ctrl Pts',(3.64379902916374,2.63888350626668,4.60007230453372));
#13402=CARTESIAN_POINT('Ctrl Pts',(3.8244536406683,2.49275908427381,4.5889585154769));
#13403=CARTESIAN_POINT('Ctrl Pts',(3.79966328939795,2.26173122045618,4.57784472642011));
#13404=CARTESIAN_POINT('Ctrl Pts',(3.59211886499353,2.15726233868846,4.56673093736329));
#13405=CARTESIAN_POINT('Ctrl Pts',(3.42236627044389,2.25700668735564,4.55731353790786));
#13406=CARTESIAN_POINT('Ctrl Pts',(3.39492411875798,2.36286981206378,4.55160073480468));
#13407=CARTESIAN_POINT('Ctrl Pts',(3.39484822543359,2.40004689761745,4.54959252805377));
#13408=CARTESIAN_POINT('Ctrl Pts',(3.3946525152789,2.40017600729827,4.62540747194623));
#13409=CARTESIAN_POINT('Ctrl Pts',(3.3944854829676,2.42064195048213,4.62429930431288));
#13410=CARTESIAN_POINT('Ctrl Pts',(3.40670159662045,2.50933048007129,4.61948654032727));
#13411=CARTESIAN_POINT('Ctrl Pts',(3.53409308462842,2.63375189718637,4.61096917998938));
#13412=CARTESIAN_POINT('Ctrl Pts',(3.76064388996454,2.58214612691277,4.59985539093257));
#13413=CARTESIAN_POINT('Ctrl Pts',(3.84015552099323,2.36381994099575,4.58874160187577));
#13414=CARTESIAN_POINT('Ctrl Pts',(3.6998500801025,2.17860977340027,4.57762781281896));
#13415=CARTESIAN_POINT('Ctrl Pts',(3.46820102232696,2.19603680731826,4.56651643617579));
#13416=CARTESIAN_POINT('Ctrl Pts',(3.3941881204111,2.33203010926412,4.55910965588488));
#13417=CARTESIAN_POINT('Ctrl Pts',(3.39418406069018,2.40000082771773,4.55540747194623));
#13418=CARTESIAN_POINT('Origin',(3.6,2.4,5.35459252805377));
#13419=CARTESIAN_POINT('',(3.39480596940119,2.39989608913133,4.69540747194623));
#13420=CARTESIAN_POINT('',(3.394211384704,2.40006787741663,4.68959252805377));
#13421=CARTESIAN_POINT('',(3.394525,2.40000000000001,5.35459252805377));
#13422=CARTESIAN_POINT('Ctrl Pts',(3.394211384704,2.40006787741663,4.68959252805377));
#13423=CARTESIAN_POINT('Ctrl Pts',(3.39419531260529,2.40380178642024,4.68938922436523));
#13424=CARTESIAN_POINT('Ctrl Pts',(3.3959796032358,2.47555925126455,4.68548132432442));
#13425=CARTESIAN_POINT('Ctrl Pts',(3.47964553527297,2.61094664572852,4.67786882793135));
#13426=CARTESIAN_POINT('Ctrl Pts',(3.71195459435803,2.61552228034691,4.66675503887453));
#13427=CARTESIAN_POINT('Ctrl Pts',(3.84179034357568,2.42282792757511,4.65564124981774));
#13428=CARTESIAN_POINT('Ctrl Pts',(3.75031264922961,2.20923891380705,4.64452746076093));
#13429=CARTESIAN_POINT('Ctrl Pts',(3.5212520823821,2.17025568561017,4.63341367170412));
#13430=CARTESIAN_POINT('Ctrl Pts',(3.40385053057498,2.29836868031663,4.62510202746841));
#13431=CARTESIAN_POINT('Ctrl Pts',(3.39439165865867,2.38316790612259,4.62049497958496));
#13432=CARTESIAN_POINT('Ctrl Pts',(3.39454318727431,2.3998121083938,4.61959252805377));
#13433=CARTESIAN_POINT('Ctrl Pts',(3.39480596940119,2.39989608913133,4.69540747194623));
#13434=CARTESIAN_POINT('Ctrl Pts',(3.39499356749685,2.44086040282664,4.69319354909316));
#13435=CARTESIAN_POINT('Ctrl Pts',(3.42673277743261,2.55063876982526,4.68727502988781));
#13436=CARTESIAN_POINT('Ctrl Pts',(3.60557055501943,2.64280164712995,4.67765191433021));
#13437=CARTESIAN_POINT('Ctrl Pts',(3.80701249526159,2.52700195958257,4.6665381252734));
#13438=CARTESIAN_POINT('Ctrl Pts',(3.81897355090948,2.29495593812904,4.65542433621659));
#13439=CARTESIAN_POINT('Ctrl Pts',(3.63050563208088,2.15905793778677,4.6443105471598));
#13440=CARTESIAN_POINT('Ctrl Pts',(3.43569204443384,2.23525749529523,4.63430492573634));
#13441=CARTESIAN_POINT('Ctrl Pts',(3.39504387077152,2.35222445101461,4.62800390066515));
#13442=CARTESIAN_POINT('Ctrl Pts',(3.3946525152789,2.40017600729827,4.62540747194623));
#13443=CARTESIAN_POINT('Origin',(3.6,2.4,5.35459252805377));
#13444=CARTESIAN_POINT('',(3.39427329960995,2.39987978133526,4.76540747194623));
#13445=CARTESIAN_POINT('',(3.3947435825044,2.40014509868052,4.75959252805377));
#13446=CARTESIAN_POINT('',(3.394525,2.40000000000001,5.35459252805377));
#13447=CARTESIAN_POINT('Ctrl Pts',(3.3947435825044,2.40014509868052,4.75959252805377));
#13448=CARTESIAN_POINT('Ctrl Pts',(3.39458577035565,2.4243482239957,4.7582834691455));
#13449=CARTESIAN_POINT('Ctrl Pts',(3.40973683471182,2.51685424764646,4.75326981388497));
#13450=CARTESIAN_POINT('Ctrl Pts',(3.54682833602434,2.63697354002902,4.74455156227216));
#13451=CARTESIAN_POINT('Ctrl Pts',(3.77025746491439,2.57319376479756,4.73343777321537));
#13452=CARTESIAN_POINT('Ctrl Pts',(3.83784800531731,2.35088777249601,4.72232398415856));
#13453=CARTESIAN_POINT('Ctrl Pts',(3.68773356907346,2.1735347589994,4.71121019510175));
#13454=CARTESIAN_POINT('Ctrl Pts',(3.46153062024069,2.20292038334059,4.70029970973349));
#13455=CARTESIAN_POINT('Ctrl Pts',(3.3944881781145,2.3357625601094,4.6930938207175));
#13456=CARTESIAN_POINT('Ctrl Pts',(3.394211384704,2.40006787741663,4.68959252805377));
#13457=CARTESIAN_POINT('Ctrl Pts',(3.39427329960995,2.39987978133526,4.76540747194623));
#13458=CARTESIAN_POINT('Ctrl Pts',(3.39469744196064,2.4608980648022,4.76208779387343));
#13459=CARTESIAN_POINT('Ctrl Pts',(3.45579877538026,2.59074744458416,4.75506351944837));
#13460=CARTESIAN_POINT('Ctrl Pts',(3.67655778221991,2.63048335496042,4.74433464867103));
#13461=CARTESIAN_POINT('Ctrl Pts',(3.8351627244929,2.46068083668937,4.73322085961423));
#13462=CARTESIAN_POINT('Ctrl Pts',(3.77852055811084,2.23533646042905,4.72210707055742));
#13463=CARTESIAN_POINT('Ctrl Pts',(3.55847650032912,2.16071048934957,4.71099328150062));
#13464=CARTESIAN_POINT('Ctrl Pts',(3.41270208696854,2.27634402495147,4.70209341529689));
#13465=CARTESIAN_POINT('Ctrl Pts',(3.39467965627817,2.37231409061976,4.69689814544543));
#13466=CARTESIAN_POINT('Ctrl Pts',(3.39480596940119,2.39989608913133,4.69540747194623));
#13467=CARTESIAN_POINT('Origin',(3.6,2.4,5.35459252805377));
#13468=CARTESIAN_POINT('',(3.39444175184043,2.40017991402784,4.83540747194624));
#13469=CARTESIAN_POINT('',(3.39473574996246,2.39985120338455,4.82959252805377));
#13470=CARTESIAN_POINT('',(3.394525,2.40000000000001,5.35459252805377));
#13471=CARTESIAN_POINT('Ctrl Pts',(3.39473574996246,2.39985120338455,4.82959252805377));
#13472=CARTESIAN_POINT('Ctrl Pts',(3.39503501794323,2.44449429908603,4.82717771392578));
#13473=CARTESIAN_POINT('Ctrl Pts',(3.43129921147106,2.55806759504416,4.82105830344552));
#13474=CARTESIAN_POINT('Ctrl Pts',(3.61869057107309,2.64214530157901,4.811234296613));
#13475=CARTESIAN_POINT('Ctrl Pts',(3.81357662871545,2.51562312999728,4.80012050755618));
#13476=CARTESIAN_POINT('Ctrl Pts',(3.81297357597085,2.28326979627357,4.78900671849939));
#13477=CARTESIAN_POINT('Ctrl Pts',(3.61743339385551,2.1577609418312,4.77789292944258));
#13478=CARTESIAN_POINT('Ctrl Pts',(3.43084782690273,2.24264334099221,4.76808819929404));
#13479=CARTESIAN_POINT('Ctrl Pts',(3.39503237387128,2.35585412553307,4.76198806549777));
#13480=CARTESIAN_POINT('Ctrl Pts',(3.3947435825044,2.40014509868052,4.75959252805377));
#13481=CARTESIAN_POINT('Ctrl Pts',(3.39444175184043,2.40017991402784,4.83540747194624));
#13482=CARTESIAN_POINT('Ctrl Pts',(3.39432006446725,2.41345772041588,4.83468663500598));
#13483=CARTESIAN_POINT('Ctrl Pts',(3.40154214948563,2.49484232576125,4.83026120171345));
#13484=CARTESIAN_POINT('Ctrl Pts',(3.51011506296999,2.62561996593247,4.82213117206865));
#13485=CARTESIAN_POINT('Ctrl Pts',(3.74080745251389,2.59788110634618,4.81101738301186));
#13486=CARTESIAN_POINT('Ctrl Pts',(3.84261718390667,2.38901942599691,4.79990359395504));
#13487=CARTESIAN_POINT('Ctrl Pts',(3.72235665540369,2.19020838956081,4.78878980489825));
#13488=CARTESIAN_POINT('Ctrl Pts',(3.49010169259086,2.18342199335841,4.77767601584144));
#13489=CARTESIAN_POINT('Ctrl Pts',(3.3977657456792,2.31768599948744,4.76988190485744));
#13490=CARTESIAN_POINT('Ctrl Pts',(3.39422412009908,2.39280468183069,4.7657923902257));
#13491=CARTESIAN_POINT('Ctrl Pts',(3.39427329960995,2.39987978133526,4.76540747194623));
#13492=CARTESIAN_POINT('Origin',(3.6,2.4,5.35459252805377));
#13493=CARTESIAN_POINT('',(3.39485784124953,2.40000781019044,4.90540747194623));
#13494=CARTESIAN_POINT('',(3.39420665921585,2.39993826201568,4.89959252805377));
#13495=CARTESIAN_POINT('',(3.394525,2.40000000000001,5.35459252805377));
#13496=CARTESIAN_POINT('Ctrl Pts',(3.39420665921585,2.39993826201568,4.89959252805377));
#13497=CARTESIAN_POINT('Ctrl Pts',(3.39446259615796,2.46459365987715,4.89607195870605));
#13498=CARTESIAN_POINT('Ctrl Pts',(3.46215556435864,2.59774588363475,4.88884679300606));
#13499=CARTESIAN_POINT('Ctrl Pts',(3.68890792061744,2.62600678347214,4.87791703095382));
#13500=CARTESIAN_POINT('Ctrl Pts',(3.83809973223177,2.44787694680091,4.86680324189701));
#13501=CARTESIAN_POINT('Ctrl Pts',(3.76935615869971,2.22592479776177,4.85568945284022));
#13502=CARTESIAN_POINT('Ctrl Pts',(3.54559897248035,2.16330565547811,4.8445756637834));
#13503=CARTESIAN_POINT('Ctrl Pts',(3.40943456861369,2.28386778049975,4.83587668885459));
#13504=CARTESIAN_POINT('Ctrl Pts',(3.39457590721621,2.37600677138249,4.83088231027805));
#13505=CARTESIAN_POINT('Ctrl Pts',(3.39473574996246,2.39985120338455,4.82959252805377));
#13506=CARTESIAN_POINT('Ctrl Pts',(3.39485784124953,2.40000781019044,4.90540747194623));
#13507=CARTESIAN_POINT('Ctrl Pts',(3.39484637525965,2.43382668251502,4.90358087978625));
#13508=CARTESIAN_POINT('Ctrl Pts',(3.41876409372263,2.5362199118863,4.898049691274));
#13509=CARTESIAN_POINT('Ctrl Pts',(3.58026192098975,2.64206213906777,4.88881390640948));
#13510=CARTESIAN_POINT('Ctrl Pts',(3.79266519873933,2.54786410019675,4.87770011735268));
#13511=CARTESIAN_POINT('Ctrl Pts',(3.82871983510845,2.3183243735256,4.86658632829587));
#13512=CARTESIAN_POINT('Ctrl Pts',(3.65542461254465,2.16354327402962,4.85547253923907));
#13513=CARTESIAN_POINT('Ctrl Pts',(3.44592887095679,2.22119506991598,4.84507958712252));
#13514=CARTESIAN_POINT('Ctrl Pts',(3.39494545222641,2.34521910726469,4.83839123135825));
#13515=CARTESIAN_POINT('Ctrl Pts',(3.39444175184043,2.40017991402784,4.83540747194624));
#13516=CARTESIAN_POINT('Origin',(3.6,2.4,5.35459252805377));
#13517=CARTESIAN_POINT('',(3.39447042093573,2.39981603086916,4.97540747194623));
#13518=CARTESIAN_POINT('',(3.39455384621585,2.40018770306997,4.96959252805377));
#13519=CARTESIAN_POINT('',(3.394525,2.40000000000001,5.35459252805377));
#13520=CARTESIAN_POINT('Ctrl Pts',(3.39455384621585,2.40018770306997,4.96959252805377));
#13521=CARTESIAN_POINT('Ctrl Pts',(3.39439993536132,2.41718968163228,4.9686707998386));
#13522=CARTESIAN_POINT('Ctrl Pts',(3.40410689916048,2.50235241402357,4.96404447527116));
#13523=CARTESIAN_POINT('Ctrl Pts',(3.52244569778922,2.63014998309056,4.95571355435144));
#13524=CARTESIAN_POINT('Ctrl Pts',(3.7513008249214,2.58997827483123,4.94459976529465));
#13525=CARTESIAN_POINT('Ctrl Pts',(3.84166859114005,2.37591729705878,4.93348597623783));
#13526=CARTESIAN_POINT('Ctrl Pts',(3.71083435517744,2.18389949043478,4.92237218718104));
#13527=CARTESIAN_POINT('Ctrl Pts',(3.47855217697512,2.18968093094735,4.91125839812423));
#13528=CARTESIAN_POINT('Ctrl Pts',(3.39580021960588,2.32515686494945,4.90366517841514));
#13529=CARTESIAN_POINT('Ctrl Pts',(3.39419328089429,2.3965585986654,4.89977655505832));
#13530=CARTESIAN_POINT('Ctrl Pts',(3.39420665921585,2.39993826201568,4.89959252805377));
#13531=CARTESIAN_POINT('Ctrl Pts',(3.39447042093573,2.39981603086916,4.97540747194623));
#13532=CARTESIAN_POINT('Ctrl Pts',(3.39496908070531,2.45384921408654,4.97247512456653));
#13533=CARTESIAN_POINT('Ctrl Pts',(3.44450059321654,2.57695438413994,4.96583818083455));
#13534=CARTESIAN_POINT('Ctrl Pts',(3.652145851588,2.63720135146115,4.95549664075031));
#13535=CARTESIAN_POINT('Ctrl Pts',(3.82756721950384,2.48483414141864,4.9443828516935));
#13536=CARTESIAN_POINT('Ctrl Pts',(3.79469373046592,2.25481727983819,4.9332690626367));
#13537=CARTESIAN_POINT('Ctrl Pts',(3.58361486203243,2.15768780841241,4.9221552735799));
#13538=CARTESIAN_POINT('Ctrl Pts',(3.41976019074743,2.26186083674666,4.91286807668307));
#13539=CARTESIAN_POINT('Ctrl Pts',(3.39486962996599,2.36523705764074,4.90728547613852));
#13540=CARTESIAN_POINT('Ctrl Pts',(3.39485784124953,2.40000781019044,4.90540747194623));
#13541=CARTESIAN_POINT('Origin',(3.6,2.4,5.35459252805377));
#13542=CARTESIAN_POINT('',(3.3942529072965,2.40010656251954,5.04540747194623));
#13543=CARTESIAN_POINT('',(3.39484564919972,2.39994744459104,5.03959252805377));
#13544=CARTESIAN_POINT('',(3.394525,2.40000000000001,5.35459252805377));
#13545=CARTESIAN_POINT('Ctrl Pts',(3.39484564919972,2.39994744459104,5.03959252805377));
#13546=CARTESIAN_POINT('Ctrl Pts',(3.39493157223083,2.43748021568483,5.03756504461887));
#13547=CARTESIAN_POINT('Ctrl Pts',(3.42276238606253,2.54371108636155,5.03183296483171));
#13548=CARTESIAN_POINT('Ctrl Pts',(3.59337897158896,2.64277529828296,5.02239628869227));
#13549=CARTESIAN_POINT('Ctrl Pts',(3.80037832359127,2.53723050760561,5.01128249963547));
#13550=CARTESIAN_POINT('Ctrl Pts',(3.82396912389365,2.30607707315216,5.00016871057866));
#13551=CARTESIAN_POINT('Ctrl Pts',(3.64255844494981,2.16089236073089,4.98905492152186));
#13552=CARTESIAN_POINT('Ctrl Pts',(3.44046962361553,2.22845545212382,4.97886286068023));
#13553=CARTESIAN_POINT('Ctrl Pts',(3.39501853158186,2.34885558191993,4.97237539619086));
#13554=CARTESIAN_POINT('Ctrl Pts',(3.39455384621585,2.40018770306997,4.96959252805377));
#13555=CARTESIAN_POINT('Ctrl Pts',(3.3942529072965,2.40010656251954,5.04540747194623));
#13556=CARTESIAN_POINT('Ctrl Pts',(3.39421422426863,2.40623506914945,5.04507396569907));
#13557=CARTESIAN_POINT('Ctrl Pts',(3.39724233203131,2.4804004332851,5.04103586309963));
#13558=CARTESIAN_POINT('Ctrl Pts',(3.48711398178203,2.61503583311392,5.03329316414794));
#13559=CARTESIAN_POINT('Ctrl Pts',(3.71944062032543,2.61146538882495,5.02217937509113));
#13560=CARTESIAN_POINT('Ctrl Pts',(3.84244192441188,2.41433825182845,5.01106558603433));
#13561=CARTESIAN_POINT('Ctrl Pts',(3.74353337567863,2.20408716238119,4.99995179697753));
#13562=CARTESIAN_POINT('Ctrl Pts',(3.51324710536571,2.17315730898832,4.98883800792072));
#13563=CARTESIAN_POINT('Ctrl Pts',(3.40217617393534,2.30323677769677,4.98065656624362));
#13564=CARTESIAN_POINT('Ctrl Pts',(3.39433909628525,2.38558611032407,4.97617972091879));
#13565=CARTESIAN_POINT('Ctrl Pts',(3.39447042093573,2.39981603086916,4.97540747194623));
#13566=CARTESIAN_POINT('Origin',(3.6,2.4,5.35459252805377));
#13567=CARTESIAN_POINT('',(3.39479089114249,2.40011619889285,5.11540747194623));
#13568=CARTESIAN_POINT('',(3.39436118415265,2.39983962587988,5.10959252805377));
#13569=CARTESIAN_POINT('',(3.394525,2.40000000000001,5.35459252805377));
#13570=CARTESIAN_POINT('Ctrl Pts',(3.39436118415265,2.39983962587988,5.10959252805377));
#13571=CARTESIAN_POINT('Ctrl Pts',(3.39485594839208,2.45749534742618,5.10645928939915));
#13572=CARTESIAN_POINT('Ctrl Pts',(3.45020483086988,2.58415305598872,5.09962145439226));
#13573=CARTESIAN_POINT('Ctrl Pts',(3.66489494817768,2.63403475512075,5.08907902303309));
#13574=CARTESIAN_POINT('Ctrl Pts',(3.83182128848718,2.47240567698227,5.0779652339763));
#13575=CARTESIAN_POINT('Ctrl Pts',(3.78655899556261,2.24450261226871,5.06685144491949));
#13576=CARTESIAN_POINT('Ctrl Pts',(3.57053712771522,2.15892819449186,5.05573765586269));
#13577=CARTESIAN_POINT('Ctrl Pts',(3.41597203014558,2.26936665662614,5.04665135024078));
#13578=CARTESIAN_POINT('Ctrl Pts',(3.39477457457446,2.36890073212835,5.04126964097114));
#13579=CARTESIAN_POINT('Ctrl Pts',(3.39484564919972,2.39994744459104,5.03959252805377));
#13580=CARTESIAN_POINT('Ctrl Pts',(3.39479089114249,2.40011619889285,5.11540747194623));
#13581=CARTESIAN_POINT('Ctrl Pts',(3.39465311263348,2.42674223574529,5.11396821047934));
#13582=CARTESIAN_POINT('Ctrl Pts',(3.4118399484044,2.5217320012959,5.10882435266019));
#13583=CARTESIAN_POINT('Ctrl Pts',(3.55516852834243,2.63869087044012,5.09997589848876));
#13584=CARTESIAN_POINT('Ctrl Pts',(3.77622353148193,2.56711958879047,5.08886210943196));
#13585=CARTESIAN_POINT('Ctrl Pts',(3.8359804180852,2.34258029751366,5.07774832037515));
#13586=CARTESIAN_POINT('Ctrl Pts',(3.6797411123384,2.17059868763558,5.06663453131835));
#13587=CARTESIAN_POINT('Ctrl Pts',(3.45739289886954,2.2074502474941,5.05585424850871));
#13588=CARTESIAN_POINT('Ctrl Pts',(3.39464391638139,2.33815945287815,5.04877856205133));
#13589=CARTESIAN_POINT('Ctrl Pts',(3.3942529072965,2.40010656251954,5.04540747194623));
#13590=CARTESIAN_POINT('Origin',(3.6,2.4,5.35459252805377));
#13591=CARTESIAN_POINT('',(3.39473291096846,2.39977036782444,5.18540747194623));
#13592=CARTESIAN_POINT('',(3.39434265438876,2.4001499379742,5.17959252805377));
#13593=CARTESIAN_POINT('',(3.394525,2.40000000000001,5.35459252805377));
#13594=CARTESIAN_POINT('',(3.54698297828114,2.20148256743283,5.2));
#13595=CARTESIAN_POINT('Ctrl Pts',(3.54698297828114,2.20148256743283,5.2));
#13596=CARTESIAN_POINT('Ctrl Pts',(3.48097120902544,2.21911198848201,5.19629540364773));
#13597=CARTESIAN_POINT('Ctrl Pts',(3.40750559920538,2.28872805295596,5.19143122762981));
#13598=CARTESIAN_POINT('Ctrl Pts',(3.39457126112442,2.3783468402669,5.18656705161189));
#13599=CARTESIAN_POINT('Ctrl Pts',(3.39473291096846,2.39977036782444,5.18540747194623));
#13600=CARTESIAN_POINT('',(3.6531315533849,2.20112677566065,5.2));
#13601=CARTESIAN_POINT('Origin',(3.6,2.4,5.2));
#13602=CARTESIAN_POINT('Ctrl Pts',(3.65313162618093,2.20112654952031,5.2));
#13603=CARTESIAN_POINT('Ctrl Pts',(3.58867175365004,2.1839946978326,5.19636770818145));
#13604=CARTESIAN_POINT('Ctrl Pts',(3.45069166079049,2.21593288928867,5.1895652175327));
#13605=CARTESIAN_POINT('Ctrl Pts',(3.39482801182151,2.34184093155955,5.18276272688396));
#13606=CARTESIAN_POINT('Ctrl Pts',(3.39434265438876,2.4001499379742,5.17959252805377));
#13607=CARTESIAN_POINT('Origin',(3.6,-2.4,4.7));
#13608=CARTESIAN_POINT('',(3.4332441194689,-2.40012144310043,4.38714803633902));
#13609=CARTESIAN_POINT('',(3.43319918361158,-2.39990306414324,4.36785196366098));
#13610=CARTESIAN_POINT('',(3.4334,-2.4,4.7));
#13611=CARTESIAN_POINT('',(3.43648706727485,-2.43192304546281,4.3));
#13612=CARTESIAN_POINT('Ctrl Pts',(3.43319918361158,-2.39990306414324,4.36785196366098));
#13613=CARTESIAN_POINT('Ctrl Pts',(3.43315842575224,-2.39409443322767,4.36746222055426));
#13614=CARTESIAN_POINT('Ctrl Pts',(3.43343544638748,-2.38828969410672,4.36707247744754));
#13615=CARTESIAN_POINT('Ctrl Pts',(3.43404308035483,-2.38251974365232,4.36668273434082));
#13616=CARTESIAN_POINT('Ctrl Pts',(3.43981877860357,-2.32767505996788,4.36297813798856));
#13617=CARTESIAN_POINT('Ctrl Pts',(3.47546516768456,-2.27597350876472,4.35927354163629));
#13618=CARTESIAN_POINT('Ctrl Pts',(3.52467802663468,-2.2510856178596,4.35556894528402));
#13619=CARTESIAN_POINT('Ctrl Pts',(3.57389088558479,-2.22619772695447,4.35186434893175));
#13620=CARTESIAN_POINT('Ctrl Pts',(3.63667021440403,-2.22812349634739,4.34815975257949));
#13621=CARTESIAN_POINT('Ctrl Pts',(3.68426556377096,-2.25596352517201,4.34445515622722));
#13622=CARTESIAN_POINT('Ctrl Pts',(3.73186091313788,-2.28380355399663,4.34075055987495));
#13623=CARTESIAN_POINT('Ctrl Pts',(3.7642722830525,-2.33755784225296,4.33704596352268));
#13624=CARTESIAN_POINT('Ctrl Pts',(3.76670489686818,-2.39266164590465,4.33334136717041));
#13625=CARTESIAN_POINT('Ctrl Pts',(3.76913751068386,-2.44776544955635,4.32963677081814));
#13626=CARTESIAN_POINT('Ctrl Pts',(3.74159136840061,-2.50421876860342,4.32593217446587));
#13627=CARTESIAN_POINT('Ctrl Pts',(3.69659414024548,-2.53611221831126,4.32222757811361));
#13628=CARTESIAN_POINT('Ctrl Pts',(3.65159691209034,-2.56800566801911,4.31852298176134));
#13629=CARTESIAN_POINT('Ctrl Pts',(3.58914859806332,-2.57533924838774,4.31481838540907));
#13630=CARTESIAN_POINT('Ctrl Pts',(3.53802492988379,-2.55491157781525,4.3111137890568));
#13631=CARTESIAN_POINT('Ctrl Pts',(3.48690126170426,-2.53448390724277,4.30740919270454));
#13632=CARTESIAN_POINT('Ctrl Pts',(3.44710223937223,-2.48629498572918,4.30370459635227));
#13633=CARTESIAN_POINT('Ctrl Pts',(3.43648706727485,-2.43192304546281,4.3));
#13634=CARTESIAN_POINT('',(3.59474332937116,-2.23318013131002,4.3));
#13635=CARTESIAN_POINT('Origin',(3.6,-2.4,4.3));
#13636=CARTESIAN_POINT('',(3.43365449489478,-2.40006497081539,4.31714803633902));
#13637=CARTESIAN_POINT('Ctrl Pts',(3.5947433329992,-2.23317993884958,4.3));
#13638=CARTESIAN_POINT('Ctrl Pts',(3.54069367702075,-2.23495318942066,4.30363229181855));
#13639=CARTESIAN_POINT('Ctrl Pts',(3.48748281579126,-2.26542182682866,4.30726458363711));
#13640=CARTESIAN_POINT('Ctrl Pts',(3.45871387185408,-2.31121589220503,4.31089687545567));
#13641=CARTESIAN_POINT('Ctrl Pts',(3.44221012289161,-2.33748636499654,4.31298059575012));
#13642=CARTESIAN_POINT('Ctrl Pts',(3.43375001435867,-2.36880031414598,4.31506431604457));
#13643=CARTESIAN_POINT('Ctrl Pts',(3.43365449489478,-2.40006497081539,4.31714803633902));
#13644=CARTESIAN_POINT('',(3.4334,-2.4,4.2));
#13645=CARTESIAN_POINT('',(3.4334,-2.4,4.7));
#13646=CARTESIAN_POINT('Origin',(3.6,-2.4,4.2));
#13647=CARTESIAN_POINT('Ctrl Pts',(3.43365449489478,-2.40006497081539,4.31714803633902));
#13648=CARTESIAN_POINT('Ctrl Pts',(3.43358019259399,-2.42438499763772,4.31876891239684));
#13649=CARTESIAN_POINT('Ctrl Pts',(3.43856722876717,-2.44867519801865,4.32038978845465));
#13650=CARTESIAN_POINT('Ctrl Pts',(3.44876666940262,-2.4705384776482,4.32201066451247));
#13651=CARTESIAN_POINT('Ctrl Pts',(3.47207802031749,-2.52050813792769,4.32571526086474));
#13652=CARTESIAN_POINT('Ctrl Pts',(3.52261765592676,-2.55780017703868,4.329419857217));
#13653=CARTESIAN_POINT('Ctrl Pts',(3.57725038923478,-2.56532196913419,4.33312445356927));
#13654=CARTESIAN_POINT('Ctrl Pts',(3.6318831225428,-2.57284376122971,4.33682904992154));
#13655=CARTESIAN_POINT('Ctrl Pts',(3.69060895354956,-2.55059530630975,4.34053364627381));
#13656=CARTESIAN_POINT('Ctrl Pts',(3.72655438362155,-2.50877157126828,4.34423824262608));
#13657=CARTESIAN_POINT('Ctrl Pts',(3.76249981369354,-2.4669478362268,4.34794283897835));
#13658=CARTESIAN_POINT('Ctrl Pts',(3.77566484283074,-2.40554882106382,4.35164743533061));
#13659=CARTESIAN_POINT('Ctrl Pts',(3.76002306731497,-2.35266772394791,4.35535203168288));
#13660=CARTESIAN_POINT('Ctrl Pts',(3.74438129179919,-2.29978662683201,4.35905662803515));
#13661=CARTESIAN_POINT('Ctrl Pts',(3.69993271163044,-2.25542344776319,4.36276122438742));
#13662=CARTESIAN_POINT('Ctrl Pts',(3.64702014743753,-2.23988444780227,4.36646582073969));
#13663=CARTESIAN_POINT('Ctrl Pts',(3.59410758324462,-2.22434544784136,4.37017041709196));
#13664=CARTESIAN_POINT('Ctrl Pts',(3.53273103502755,-2.23763062698835,4.37387501344422));
#13665=CARTESIAN_POINT('Ctrl Pts',(3.49097949059372,-2.27365834937589,4.37757960979649));
#13666=CARTESIAN_POINT('Ctrl Pts',(3.45503346139427,-2.30467644890953,4.38076908531067));
#13667=CARTESIAN_POINT('Ctrl Pts',(3.43363419992272,-2.35255214998637,4.38395856082484));
#13668=CARTESIAN_POINT('Ctrl Pts',(3.4332441194689,-2.40012144310043,4.38714803633902));
#13669=CARTESIAN_POINT('Origin',(3.6,-2.4,4.7));
#13670=CARTESIAN_POINT('',(3.4332753032246,-2.39986752249821,4.45714803633902));
#13671=CARTESIAN_POINT('',(3.43362893615635,-2.39991676750829,4.43785196366098));
#13672=CARTESIAN_POINT('',(3.4334,-2.4,4.7));
#13673=CARTESIAN_POINT('Ctrl Pts',(3.43362893615635,-2.39991676750829,4.43785196366098));
#13674=CARTESIAN_POINT('Ctrl Pts',(3.43352745251214,-2.37748041857078,4.43635646533454));
#13675=CARTESIAN_POINT('Ctrl Pts',(3.43774838897563,-2.35508066415019,4.43486096700809));
#13676=CARTESIAN_POINT('Ctrl Pts',(3.44647311482898,-2.33459946287839,4.43336546868165));
#13677=CARTESIAN_POINT('Ctrl Pts',(3.46808570175023,-2.28386414463698,4.42966087232938));
#13678=CARTESIAN_POINT('Ctrl Pts',(3.51733510423541,-2.24490173470295,4.42595627597711));
#13679=CARTESIAN_POINT('Ctrl Pts',(3.57168220229163,-2.23554374099052,4.42225167962485));
#13680=CARTESIAN_POINT('Ctrl Pts',(3.62602930034785,-2.22618574727809,4.41854708327258));
#13681=CARTESIAN_POINT('Ctrl Pts',(3.68547409397512,-2.24643216978725,4.41484248692031));
#13682=CARTESIAN_POINT('Ctrl Pts',(3.72281103935986,-2.2870168380163,4.41113789056804));
#13683=CARTESIAN_POINT('Ctrl Pts',(3.7601479847446,-2.32760150624535,4.40743329421577));
#13684=CARTESIAN_POINT('Ctrl Pts',(3.77537708188681,-2.38852442019428,4.4037286978635));
#13685=CARTESIAN_POINT('Ctrl Pts',(3.76152924259544,-2.44190442427593,4.40002410151124));
#13686=CARTESIAN_POINT('Ctrl Pts',(3.74768140330407,-2.49528442835759,4.39631950515897));
#13687=CARTESIAN_POINT('Ctrl Pts',(3.70475662757912,-2.54112152257198,4.3926149088067));
#13688=CARTESIAN_POINT('Ctrl Pts',(3.65239849228647,-2.55843697682615,4.38891031245443));
#13689=CARTESIAN_POINT('Ctrl Pts',(3.60004035699382,-2.57575243108032,4.38520571610217));
#13690=CARTESIAN_POINT('Ctrl Pts',(3.53824886213347,-2.56454624537428,4.3815011197499));
#13691=CARTESIAN_POINT('Ctrl Pts',(3.49530561841154,-2.52994924443839,4.37779652339763));
#13692=CARTESIAN_POINT('Ctrl Pts',(3.45688023078761,-2.49899203076829,4.37448167015208));
#13693=CARTESIAN_POINT('Ctrl Pts',(3.43354583842081,-2.4493067834413,4.37116681690653));
#13694=CARTESIAN_POINT('Ctrl Pts',(3.43319918361158,-2.39990306414324,4.36785196366098));
#13695=CARTESIAN_POINT('Ctrl Pts',(3.4332441194689,-2.40012144310043,4.38714803633902));
#13696=CARTESIAN_POINT('Ctrl Pts',(3.4331811189632,-2.40780419031934,4.38766315717711));
#13697=CARTESIAN_POINT('Ctrl Pts',(3.43366612887655,-2.41547894509172,4.3881782780152));
#13698=CARTESIAN_POINT('Ctrl Pts',(3.43472637398198,-2.42307339909524,4.3886933988533));
#13699=CARTESIAN_POINT('Ctrl Pts',(3.44235134245467,-2.47769046079897,4.39239799520556));
#13700=CARTESIAN_POINT('Ctrl Pts',(3.47972782005064,-2.52815431857834,4.39610259155783));
#13701=CARTESIAN_POINT('Ctrl Pts',(3.5297501656918,-2.5513695031952,4.3998071879101));
#13702=CARTESIAN_POINT('Ctrl Pts',(3.57977251133296,-2.57458468781207,4.40351178426237));
#13703=CARTESIAN_POINT('Ctrl Pts',(3.64244072501932,-2.57055119926642,4.40721638061463));
#13704=CARTESIAN_POINT('Ctrl Pts',(3.68907438543537,-2.54111518550135,4.4109209769669));
#13705=CARTESIAN_POINT('Ctrl Pts',(3.73570804585142,-2.51167917173628,4.41462557331917));
#13706=CARTESIAN_POINT('Ctrl Pts',(3.76630715299715,-2.4568406327518,4.41833016967144));
#13707=CARTESIAN_POINT('Ctrl Pts',(3.76686783098938,-2.40169663747488,4.42203476602371));
#13708=CARTESIAN_POINT('Ctrl Pts',(3.7674285089816,-2.34655264219797,4.42573936237597));
#13709=CARTESIAN_POINT('Ctrl Pts',(3.73795075782031,-2.29110319062863,4.42944395872824));
#13710=CARTESIAN_POINT('Ctrl Pts',(3.69192524795617,-2.26072508833266,4.43314855508051));
#13711=CARTESIAN_POINT('Ctrl Pts',(3.64589973809204,-2.23034698603669,4.43685315143278));
#13712=CARTESIAN_POINT('Ctrl Pts',(3.58332646952505,-2.2250402330141,4.44055774778505));
#13713=CARTESIAN_POINT('Ctrl Pts',(3.53284244819528,-2.24723347009038,4.44426234413732));
#13714=CARTESIAN_POINT('Ctrl Pts',(3.48235842686551,-2.26942670716666,4.44796694048958));
#13715=CARTESIAN_POINT('Ctrl Pts',(3.44396365277294,-2.31911993434182,4.45167153684185));
#13716=CARTESIAN_POINT('Ctrl Pts',(3.43522971460805,-2.37357077679719,4.45537613319412));
#13717=CARTESIAN_POINT('Ctrl Pts',(3.43383723789082,-2.38225203019296,4.45596676757575));
#13718=CARTESIAN_POINT('Ctrl Pts',(3.4331987050974,-2.39105421663124,4.45655740195739));
#13719=CARTESIAN_POINT('Ctrl Pts',(3.4332753032246,-2.39986752249821,4.45714803633902));
#13720=CARTESIAN_POINT('Origin',(3.6,-2.4,4.7));
#13721=CARTESIAN_POINT('',(3.43366207720083,-2.39996197521424,4.52714803633902));
#13722=CARTESIAN_POINT('',(3.43350143827108,-2.40014312936039,4.50785196366098));
#13723=CARTESIAN_POINT('',(3.4334,-2.4,4.7));
#13724=CARTESIAN_POINT('Ctrl Pts',(3.43350143827108,-2.40014312936039,4.50785196366098));
#13725=CARTESIAN_POINT('Ctrl Pts',(3.43382055454292,-2.36119271753362,4.50525071011481));
#13726=CARTESIAN_POINT('Ctrl Pts',(3.44745634567654,-2.3220410177822,4.50264945656865));
#13727=CARTESIAN_POINT('Ctrl Pts',(3.4724157519356,-2.29243605104842,4.50004820302248));
#13728=CARTESIAN_POINT('Ctrl Pts',(3.50796189295608,-2.25027389736965,4.49634360667021));
#13729=CARTESIAN_POINT('Ctrl Pts',(3.56647488846456,-2.22747467908062,4.49263901031794));
#13730=CARTESIAN_POINT('Ctrl Pts',(3.62117593657879,-2.23447258988711,4.48893441396567));
#13731=CARTESIAN_POINT('Ctrl Pts',(3.67587698469302,-2.2414705006936,4.4852298176134));
#13732=CARTESIAN_POINT('Ctrl Pts',(3.726766085413,-2.27826554059562,4.48152522126114));
#13733=CARTESIAN_POINT('Ctrl Pts',(3.75055354862185,-2.32801824658462,4.47782062490887));
#13734=CARTESIAN_POINT('Ctrl Pts',(3.7743410118307,-2.37777095257363,4.4741160285566));
#13735=CARTESIAN_POINT('Ctrl Pts',(3.77102683752841,-2.44048132464963,4.47041143220433));
#13736=CARTESIAN_POINT('Ctrl Pts',(3.74212778560952,-2.48744961415947,4.46670683585206));
#13737=CARTESIAN_POINT('Ctrl Pts',(3.71322873369063,-2.53441790366931,4.4630022394998));
#13738=CARTESIAN_POINT('Ctrl Pts',(3.65874480415513,-2.56564411061299,4.45929764314753));
#13739=CARTESIAN_POINT('Ctrl Pts',(3.60361085781629,-2.56683736686161,4.45559304679526));
#13740=CARTESIAN_POINT('Ctrl Pts',(3.54847691147744,-2.56803062311024,4.45188845044299));
#13741=CARTESIAN_POINT('Ctrl Pts',(3.49269294833524,-2.5391909286638,4.44818385409072));
#13742=CARTESIAN_POINT('Ctrl Pts',(3.46178885244281,-2.49351696816619,4.44447925773846));
#13743=CARTESIAN_POINT('Ctrl Pts',(3.44336034614035,-2.46628100333426,4.44227015971263));
#13744=CARTESIAN_POINT('Ctrl Pts',(3.43377884425998,-2.43305896049386,4.4400610616868));
#13745=CARTESIAN_POINT('Ctrl Pts',(3.43362893615635,-2.39991676750829,4.43785196366098));
#13746=CARTESIAN_POINT('Ctrl Pts',(3.4332753032246,-2.39986752249821,4.45714803633902));
#13747=CARTESIAN_POINT('Ctrl Pts',(3.43367914638464,-2.44633332293026,4.46026199830965));
#13748=CARTESIAN_POINT('Ctrl Pts',(3.45396108248041,-2.49310820388228,4.46337596028029));
#13749=CARTESIAN_POINT('Ctrl Pts',(3.48843309316639,-2.52409905740531,4.46648992225092));
#13750=CARTESIAN_POINT('Ctrl Pts',(3.52944351212684,-2.56096803782247,4.47019451860319));
#13751=CARTESIAN_POINT('Ctrl Pts',(3.59053745228497,-2.57549754092119,4.47389911495546));
#13752=CARTESIAN_POINT('Ctrl Pts',(3.64375492615303,-2.56103806030718,4.47760371130773));
#13753=CARTESIAN_POINT('Ctrl Pts',(3.69697240002109,-2.54657857969317,4.48130830766));
#13754=CARTESIAN_POINT('Ctrl Pts',(3.74231340759908,-2.50313011536643,4.48501290401227));
#13755=CARTESIAN_POINT('Ctrl Pts',(3.75902737934242,-2.45057710185421,4.48871750036453));
#13756=CARTESIAN_POINT('Ctrl Pts',(3.77574135108577,-2.39802408834199,4.4924220967168));
#13757=CARTESIAN_POINT('Ctrl Pts',(3.76382828699448,-2.33636652564429,4.49612669306907));
#13758=CARTESIAN_POINT('Ctrl Pts',(3.72874026856414,-2.29382234772163,4.49983128942134));
#13759=CARTESIAN_POINT('Ctrl Pts',(3.6936522501338,-2.25127816979896,4.5035358857736));
#13760=CARTESIAN_POINT('Ctrl Pts',(3.63538927736442,-2.22784737665133,4.50724048212587));
#13761=CARTESIAN_POINT('Ctrl Pts',(3.58061573003626,-2.23425320323999,4.51094507847814));
#13762=CARTESIAN_POINT('Ctrl Pts',(3.52584218270809,-2.24065902982864,4.51464967483041));
#13763=CARTESIAN_POINT('Ctrl Pts',(3.47455806082114,-2.27690147615359,4.51835427118267));
#13764=CARTESIAN_POINT('Ctrl Pts',(3.45023383359826,-2.32639398133752,4.52205886753494));
#13765=CARTESIAN_POINT('Ctrl Pts',(3.43909540927391,-2.34905733333477,4.5237552571363));
#13766=CARTESIAN_POINT('Ctrl Pts',(3.4336100971438,-2.37449903703717,4.52545164673766));
#13767=CARTESIAN_POINT('Ctrl Pts',(3.43366207720083,-2.39996197521424,4.52714803633902));
#13768=CARTESIAN_POINT('Origin',(3.6,-2.4,4.7));
#13769=CARTESIAN_POINT('',(3.43341475097665,-2.4001523433056,4.59714803633902));
#13770=CARTESIAN_POINT('',(3.43312356989615,-2.39999932887968,4.57785196366098));
#13771=CARTESIAN_POINT('',(3.4334,-2.4,4.7));
#13772=CARTESIAN_POINT('Ctrl Pts',(3.4331235712606,-2.39999932888299,4.57785196366098));
#13773=CARTESIAN_POINT('Ctrl Pts',(3.43312027533203,-2.34481656196242,4.57414495489509));
#13774=CARTESIAN_POINT('Ctrl Pts',(3.46320503039949,-2.28963688420389,4.57043794612919));
#13775=CARTESIAN_POINT('Ctrl Pts',(3.50958660961886,-2.25973894891049,4.5667309373633));
#13776=CARTESIAN_POINT('Ctrl Pts',(3.55593800505376,-2.22986047032491,4.56302634101103));
#13777=CARTESIAN_POINT('Ctrl Pts',(3.61856500889817,-2.22523083965654,4.55932174465877));
#13778=CARTESIAN_POINT('Ctrl Pts',(3.66880601775922,-2.24796883366633,4.5556171483065));
#13779=CARTESIAN_POINT('Ctrl Pts',(3.71904702662027,-2.27070682767613,4.55191255195423));
#13780=CARTESIAN_POINT('Ctrl Pts',(3.75690204049796,-2.32081244636408,4.54820795560196));
#13781=CARTESIAN_POINT('Ctrl Pts',(3.765046497567,-2.37535456915184,4.54450335924969));
#13782=CARTESIAN_POINT('Ctrl Pts',(3.77319095463605,-2.4298966919396,4.54079876289742));
#13783=CARTESIAN_POINT('Ctrl Pts',(3.75162485489646,-2.48887531882715,4.53709416654515));
#13784=CARTESIAN_POINT('Ctrl Pts',(3.71021804632554,-2.52529854692327,4.53338957019289));
#13785=CARTESIAN_POINT('Ctrl Pts',(3.66881123775463,-2.56172177501939,4.52968497384062));
#13786=CARTESIAN_POINT('Ctrl Pts',(3.60756372035239,-2.57558960432407,4.52598037748835));
#13787=CARTESIAN_POINT('Ctrl Pts',(3.55450576746795,-2.56055534384899,4.52227578113609));
#13788=CARTESIAN_POINT('Ctrl Pts',(3.5014478145835,-2.5455210833739,4.51857118478382));
#13789=CARTESIAN_POINT('Ctrl Pts',(3.45657942621685,-2.50158473311904,4.51486658843155));
#13790=CARTESIAN_POINT('Ctrl Pts',(3.44043487529976,-2.44885401345736,4.51116199207928));
#13791=CARTESIAN_POINT('Ctrl Pts',(3.43562653117309,-2.43314918230523,4.51005864927318));
#13792=CARTESIAN_POINT('Ctrl Pts',(3.43336608251409,-2.41666426269897,4.50895530646708));
#13793=CARTESIAN_POINT('Ctrl Pts',(3.43350143827108,-2.40014312936039,4.50785196366098));
#13794=CARTESIAN_POINT('Ctrl Pts',(3.43366207720083,-2.39996197521424,4.52714803633902));
#13795=CARTESIAN_POINT('Ctrl Pts',(3.43372361182786,-2.43010531274957,4.52915624308993));
#13796=CARTESIAN_POINT('Ctrl Pts',(3.4415451707818,-2.46027840851952,4.53116444984084));
#13797=CARTESIAN_POINT('Ctrl Pts',(3.45693460775185,-2.48590718316162,4.53317265659175));
#13798=CARTESIAN_POINT('Ctrl Pts',(3.48532394168714,-2.53318531575888,4.53687725294402));
#13799=CARTESIAN_POINT('Ctrl Pts',(3.53946694211655,-2.5649990169105,4.54058184929628));
#13800=CARTESIAN_POINT('Ctrl Pts',(3.59458475789197,-2.56678856593634,4.54428644564855));
#13801=CARTESIAN_POINT('Ctrl Pts',(3.64970257366739,-2.56857811496219,4.54799104200082));
#13802=CARTESIAN_POINT('Ctrl Pts',(3.70579520478882,-2.54034351186226,4.55169563835309));
#13803=CARTESIAN_POINT('Ctrl Pts',(3.73719154055164,-2.49500648282243,4.55540023470536));
#13804=CARTESIAN_POINT('Ctrl Pts',(3.76858787631446,-2.4496694537826,4.55910483105763));
#13805=CARTESIAN_POINT('Ctrl Pts',(3.77528791671867,-2.38722999880286,4.56280942740989));
#13806=CARTESIAN_POINT('Ctrl Pts',(3.75422535028399,-2.33626388852243,4.56651402376216));
#13807=CARTESIAN_POINT('Ctrl Pts',(3.73316278384931,-2.28529777824199,4.57021862011443));
#13808=CARTESIAN_POINT('Ctrl Pts',(3.68433761057573,-2.24580501266085,4.5739232164667));
#13809=CARTESIAN_POINT('Ctrl Pts',(3.63009494786823,-2.23585967988047,4.57762781281896));
#13810=CARTESIAN_POINT('Ctrl Pts',(3.57585228516072,-2.22591434710008,4.58133240917123));
#13811=CARTESIAN_POINT('Ctrl Pts',(3.51619213301928,-2.24551644712046,4.5850370055235));
#13812=CARTESIAN_POINT('Ctrl Pts',(3.47841829836813,-2.28569496771878,4.58874160187577));
#13813=CARTESIAN_POINT('Ctrl Pts',(3.4498462907659,-2.31608587207317,4.59154374669685));
#13814=CARTESIAN_POINT('Ctrl Pts',(3.43379623586762,-2.35824928979842,4.59434589151794));
#13815=CARTESIAN_POINT('Ctrl Pts',(3.43341475097665,-2.4001523433056,4.59714803633902));
#13816=CARTESIAN_POINT('Origin',(3.6,-2.4,4.7));
#13817=CARTESIAN_POINT('',(3.43314572405529,-2.39994496470472,4.66714803633902));
#13818=CARTESIAN_POINT('',(3.43350339621029,-2.39985729254273,4.64785196366098));
#13819=CARTESIAN_POINT('',(3.4334,-2.4,4.7));
#13820=CARTESIAN_POINT('Ctrl Pts',(3.43350339621029,-2.39985729254273,4.64785196366098));
#13821=CARTESIAN_POINT('Ctrl Pts',(3.43336796571017,-2.38326341978069,4.64674379602763));
#13822=CARTESIAN_POINT('Ctrl Pts',(3.43564862259693,-2.36670593582693,4.64563562839428));
#13823=CARTESIAN_POINT('Ctrl Pts',(3.44049848254047,-2.3509387164529,4.64452746076093));
#13824=CARTESIAN_POINT('Ctrl Pts',(3.45671152911857,-2.29822901656582,4.64082286440866));
#13825=CARTESIAN_POINT('Ctrl Pts',(3.50163696254783,-2.25435099787568,4.6371182680564));
#13826=CARTESIAN_POINT('Ctrl Pts',(3.55471440347455,-2.23938568444105,4.63341367170413));
#13827=CARTESIAN_POINT('Ctrl Pts',(3.60779184440126,-2.22442037100641,4.62970907535186));
#13828=CARTESIAN_POINT('Ctrl Pts',(3.66902129282543,-2.23836776282728,4.62600447899959));
#13829=CARTESIAN_POINT('Ctrl Pts',(3.71038074448169,-2.27484475695027,4.62229988264732));
#13830=CARTESIAN_POINT('Ctrl Pts',(3.75174019613796,-2.31132175107326,4.61859528629505));
#13831=CARTESIAN_POINT('Ctrl Pts',(3.77322965102632,-2.37032834749837,4.61489068994278));
#13832=CARTESIAN_POINT('Ctrl Pts',(3.76501433826252,-2.42485984278043,4.61118609359052));
#13833=CARTESIAN_POINT('Ctrl Pts',(3.75679902549871,-2.47939133806249,4.60748149723825));
#13834=CARTESIAN_POINT('Ctrl Pts',(3.71887894508274,-2.52944773220152,4.60377690088598));
#13835=CARTESIAN_POINT('Ctrl Pts',(3.66860843684067,-2.55212043258282,4.60007230453372));
#13836=CARTESIAN_POINT('Ctrl Pts',(3.6183379285986,-2.57479313296412,4.59636770818145));
#13837=CARTESIAN_POINT('Ctrl Pts',(3.55571699253044,-2.5700821395877,4.59266311182918));
#13838=CARTESIAN_POINT('Ctrl Pts',(3.50940445510819,-2.54014346528121,4.58895851547691));
#13839=CARTESIAN_POINT('Ctrl Pts',(3.46312207616628,-2.51022428688169,4.58525633153827));
#13840=CARTESIAN_POINT('Ctrl Pts',(3.43312686289939,-2.45511027311999,4.58155414759963));
#13841=CARTESIAN_POINT('Ctrl Pts',(3.4331235712606,-2.39999932888299,4.57785196366098));
#13842=CARTESIAN_POINT('Ctrl Pts',(3.43341475097665,-2.4001523433056,4.59714803633902));
#13843=CARTESIAN_POINT('Ctrl Pts',(3.43329189093694,-2.41364753260286,4.5980504878702));
#13844=CARTESIAN_POINT('Ctrl Pts',(3.43479419036014,-2.42711571666781,4.59895293940139));
#13845=CARTESIAN_POINT('Ctrl Pts',(3.43802675920227,-2.44015494791281,4.59985539093257));
#13846=CARTESIAN_POINT('Ctrl Pts',(3.45129657184842,-2.49368146633226,4.60355998728484));
#13847=CARTESIAN_POINT('Ctrl Pts',(3.49372371430156,-2.53997956199491,4.60726458363711));
#13848=CARTESIAN_POINT('Ctrl Pts',(3.54589116423991,-2.55786064889342,4.61096917998938));
#13849=CARTESIAN_POINT('Ctrl Pts',(3.59805861417826,-2.57574173579194,4.61467377634165));
#13850=CARTESIAN_POINT('Ctrl Pts',(3.65996637160182,-2.56520581392632,4.61837837269391));
#13851=CARTESIAN_POINT('Ctrl Pts',(3.70328200028476,-2.53107470768073,4.62208296904618));
#13852=CARTESIAN_POINT('Ctrl Pts',(3.74659762896771,-2.49694360143515,4.62578756539845));
#13853=CARTESIAN_POINT('Ctrl Pts',(3.77132112891003,-2.43921731080961,4.62949216175072));
#13854=CARTESIAN_POINT('Ctrl Pts',(3.76613765017139,-2.3843146000394,4.63319675810299));
#13855=CARTESIAN_POINT('Ctrl Pts',(3.76095417143275,-2.32941188926919,4.63690135445526));
#13856=CARTESIAN_POINT('Ctrl Pts',(3.72586371401314,-2.27733275835431,4.64060595080752));
#13857=CARTESIAN_POINT('Ctrl Pts',(3.67692562472706,-2.25191151686662,4.64431054715979));
#13858=CARTESIAN_POINT('Ctrl Pts',(3.62798753544098,-2.22649027537894,4.64801514351206));
#13859=CARTESIAN_POINT('Ctrl Pts',(3.56520181428843,-2.22772692331845,4.65171973986433));
#13860=CARTESIAN_POINT('Ctrl Pts',(3.51730270257413,-2.25505550174341,4.6554243362166));
#13861=CARTESIAN_POINT('Ctrl Pts',(3.46940359085983,-2.28238408016837,4.65912893256887));
#13862=CARTESIAN_POINT('Ctrl Pts',(3.43639108858378,-2.33580458907878,4.66283352892113));
#13863=CARTESIAN_POINT('Ctrl Pts',(3.43337355460624,-2.39086882965689,4.6665381252734));
#13864=CARTESIAN_POINT('Ctrl Pts',(3.43320795605525,-2.39389068741188,4.66674142896194));
#13865=CARTESIAN_POINT('Ctrl Pts',(3.43313269272996,-2.39691749555954,4.66694473265048));
#13866=CARTESIAN_POINT('Ctrl Pts',(3.43314572405529,-2.39994496470472,4.66714803633902));
#13867=CARTESIAN_POINT('Origin',(3.6,-2.4,4.7));
#13868=CARTESIAN_POINT('',(3.43357723227316,-2.39988235337877,4.73714803633902));
#13869=CARTESIAN_POINT('',(3.43362781745768,-2.40008425136911,4.71785196366098));
#13870=CARTESIAN_POINT('',(3.4334,-2.4,4.7));
#13871=CARTESIAN_POINT('Ctrl Pts',(3.43362781745768,-2.40008425136911,4.71785196366098));
#13872=CARTESIAN_POINT('Ctrl Pts',(3.43377992278221,-2.36687021363152,4.7156380408079));
#13873=CARTESIAN_POINT('Ctrl Pts',(3.44340627006936,-2.33357497132763,4.71342411795483));
#13874=CARTESIAN_POINT('Ctrl Pts',(3.46191047910031,-2.30630353350919,4.71121019510175));
#13875=CARTESIAN_POINT('Ctrl Pts',(3.49287390006255,-2.260669753216,4.70750559874949));
#13876=CARTESIAN_POINT('Ctrl Pts',(3.54869526474406,-2.23190257855334,4.70380100239722));
#13877=CARTESIAN_POINT('Ctrl Pts',(3.60382760906969,-2.23316747012655,4.70009640604495));
#13878=CARTESIAN_POINT('Ctrl Pts',(3.65895995339532,-2.23443236169976,4.69639180969269));
#13879=CARTESIAN_POINT('Ctrl Pts',(3.71340327736507,-2.26572931950883,4.69268721334041));
#13880=CARTESIAN_POINT('Ctrl Pts',(3.74224128504954,-2.31273511334664,4.68898261698815));
#13881=CARTESIAN_POINT('Ctrl Pts',(3.77107929273401,-2.35974090718445,4.68527802063588));
#13882=CARTESIAN_POINT('Ctrl Pts',(3.7743119841332,-2.42245553705099,4.68157342428361));
#13883=CARTESIAN_POINT('Ctrl Pts',(3.75045989969766,-2.47217729697168,4.67786882793135));
#13884=CARTESIAN_POINT('Ctrl Pts',(3.72660781526212,-2.52189905689238,4.67416423157908));
#13885=CARTESIAN_POINT('Ctrl Pts',(3.67567095499184,-2.55862794686723,4.67045963522681));
#13886=CARTESIAN_POINT('Ctrl Pts',(3.62096086182118,-2.56555478213231,4.66675503887454));
#13887=CARTESIAN_POINT('Ctrl Pts',(3.56625076865053,-2.57248161739739,4.66305044252227));
#13888=CARTESIAN_POINT('Ctrl Pts',(3.50776744257951,-2.54960639795269,4.65934584617));
#13889=CARTESIAN_POINT('Ctrl Pts',(3.47227610940747,-2.50739809768834,4.65564124981773));
#13890=CARTESIAN_POINT('Ctrl Pts',(3.44740141107113,-2.47781569988784,4.65304482109882));
#13891=CARTESIAN_POINT('Ctrl Pts',(3.43382070888877,-2.43873661594181,4.6504483923799));
#13892=CARTESIAN_POINT('Ctrl Pts',(3.43350339621029,-2.39985729254273,4.64785196366098));
#13893=CARTESIAN_POINT('Ctrl Pts',(3.43314572405529,-2.39994496470472,4.66714803633902));
#13894=CARTESIAN_POINT('Ctrl Pts',(3.43337014931821,-2.45208398679426,4.67064932900275));
#13895=CARTESIAN_POINT('Ctrl Pts',(3.45978247638053,-2.50441905856693,4.67415062166648));
#13896=CARTESIAN_POINT('Ctrl Pts',(3.50195948177967,-2.53504002133992,4.67765191433021));
#13897=CARTESIAN_POINT('Ctrl Pts',(3.54658550860969,-2.56743900019905,4.68135651068247));
#13898=CARTESIAN_POINT('Ctrl Pts',(3.60886012794877,-2.57552898567153,4.68506110703474));
#13899=CARTESIAN_POINT('Ctrl Pts',(3.66028300713527,-2.55560755003253,4.68876570338701));
#13900=CARTESIAN_POINT('Ctrl Pts',(3.71170588632177,-2.53568611439352,4.69247029973927));
#13901=CARTESIAN_POINT('Ctrl Pts',(3.7522770253557,-2.48775325764304,4.69617489609154));
#13902=CARTESIAN_POINT('Ctrl Pts',(3.76342881240416,-2.43374572347072,4.69987949244381));
#13903=CARTESIAN_POINT('Ctrl Pts',(3.77458059945262,-2.3797381892984,4.70358408879608));
#13904=CARTESIAN_POINT('Ctrl Pts',(3.75631303451563,-2.31965597770425,4.70728868514835));
#13905=CARTESIAN_POINT('Ctrl Pts',(3.71698637227073,-2.28099605351363,4.71099328150061));
#13906=CARTESIAN_POINT('Ctrl Pts',(3.67765971002583,-2.24233612932302,4.71469787785288));
#13907=CARTESIAN_POINT('Ctrl Pts',(3.61727395047302,-2.22509849253594,4.71840247420515));
#13908=CARTESIAN_POINT('Ctrl Pts',(3.5634649788822,-2.23717204537206,4.72210707055742));
#13909=CARTESIAN_POINT('Ctrl Pts',(3.50965600729138,-2.24924559820818,4.72581166690969));
#13910=CARTESIAN_POINT('Ctrl Pts',(3.46242382366254,-2.29063034066749,4.72951626326196));
#13911=CARTESIAN_POINT('Ctrl Pts',(3.44338450465812,-2.34238631069604,4.73322085961423));
#13912=CARTESIAN_POINT('Ctrl Pts',(3.43665675680651,-2.36067483856233,4.73452991852249));
#13913=CARTESIAN_POINT('Ctrl Pts',(3.43344927751834,-2.38025835744364,4.73583897743076));
#13914=CARTESIAN_POINT('Ctrl Pts',(3.43357723227316,-2.39988235337877,4.73714803633902));
#13915=CARTESIAN_POINT('Origin',(3.6,-2.4,4.7));
#13916=CARTESIAN_POINT('',(3.43357088161517,-2.40012064492246,4.80714803633902));
#13917=CARTESIAN_POINT('',(3.43319592655187,-2.40009747379871,4.78785196366098));
#13918=CARTESIAN_POINT('',(3.4334,-2.4,4.7));
#13919=CARTESIAN_POINT('Ctrl Pts',(3.43319592655187,-2.40009747379871,4.78785196366098));
#13920=CARTESIAN_POINT('Ctrl Pts',(3.43353982295269,-2.35062359307345,4.78453228558818));
#13921=CARTESIAN_POINT('Ctrl Pts',(3.45695304474081,-2.30086703036466,4.78121260751538));
#13922=CARTESIAN_POINT('Ctrl Pts',(3.49547520498793,-2.2699142173685,4.77789292944258));
#13923=CARTESIAN_POINT('Ctrl Pts',(3.53846402836278,-2.23537241072238,4.77418833309031));
#13924=CARTESIAN_POINT('Ctrl Pts',(3.6002686999986,-2.22424776884202,4.77048373673804));
#13925=CARTESIAN_POINT('Ctrl Pts',(3.65260396146494,-2.24163154716497,4.76677914038577));
#13926=CARTESIAN_POINT('Ctrl Pts',(3.70493922293128,-2.25901532548792,4.76307454403351));
#13927=CARTESIAN_POINT('Ctrl Pts',(3.74780507422814,-2.30490752401418,4.75936994768124));
#13928=CARTESIAN_POINT('Ctrl Pts',(3.7615837154436,-2.35830531786175,4.75566535132897));
#13929=CARTESIAN_POINT('Ctrl Pts',(3.77536235665906,-2.41170311170932,4.75196075497671));
#13930=CARTESIAN_POINT('Ctrl Pts',(3.76005378779311,-2.4726065008782,4.74825615862444));
#13931=CARTESIAN_POINT('Ctrl Pts',(3.72266406219276,-2.51314270396953,4.74455156227217));
#13932=CARTESIAN_POINT('Ctrl Pts',(3.68527433659241,-2.55367890706087,4.7408469659199));
#13933=CARTESIAN_POINT('Ctrl Pts',(3.62580345425764,-2.57384792407467,4.73714236956763));
#13934=CARTESIAN_POINT('Ctrl Pts',(3.57146860171181,-2.56441929000846,4.73343777321536));
#13935=CARTESIAN_POINT('Ctrl Pts',(3.51713374916598,-2.55499065594226,4.7297331768631));
#13936=CARTESIAN_POINT('Ctrl Pts',(3.46793492640908,-2.51596437079605,4.72602858051083));
#13937=CARTESIAN_POINT('Ctrl Pts',(3.4463882536521,-2.46520103526108,4.72232398415856));
#13938=CARTESIAN_POINT('Ctrl Pts',(3.43771819866623,-2.44477463739825,4.72083331065937));
#13939=CARTESIAN_POINT('Ctrl Pts',(3.43352540224658,-2.42244785170318,4.71934263716017));
#13940=CARTESIAN_POINT('Ctrl Pts',(3.43362781745768,-2.40008425136911,4.71785196366098));
#13941=CARTESIAN_POINT('Ctrl Pts',(3.43357723227316,-2.39988235337877,4.73714803633902));
#13942=CARTESIAN_POINT('Ctrl Pts',(3.43381138552965,-2.4357936609347,4.73954357378302));
#13943=CARTESIAN_POINT('Ctrl Pts',(3.44521519749436,-2.4718405175289,4.74193911122702));
#13944=CARTESIAN_POINT('Ctrl Pts',(3.46665596946098,-2.50033503922361,4.74433464867103));
#13945=CARTESIAN_POINT('Ctrl Pts',(3.49981320764826,-2.54440060012484,4.74803924502329));
#13946=CARTESIAN_POINT('Ctrl Pts',(3.55697413840284,-2.57040452432951,4.75174384137556));
#13947=CARTESIAN_POINT('Ctrl Pts',(3.61197873764036,-2.56644596847307,4.75544843772783));
#13948=CARTESIAN_POINT('Ctrl Pts',(3.66698333687788,-2.56248741261664,4.7591530340801));
#13949=CARTESIAN_POINT('Ctrl Pts',(3.71983160459833,-2.52856637669909,4.76285763043237));
#13950=CARTESIAN_POINT('Ctrl Pts',(3.7463372314094,-2.48020701515346,4.76656222678464));
#13951=CARTESIAN_POINT('Ctrl Pts',(3.77284285822047,-2.43184765360783,4.7702668231369));
#13952=CARTESIAN_POINT('Ctrl Pts',(3.77300584412214,-2.36904996643411,4.77397141948917));
#13953=CARTESIAN_POINT('Ctrl Pts',(3.74675159769234,-2.32055367125447,4.77767601584144));
#13954=CARTESIAN_POINT('Ctrl Pts',(3.72049735126253,-2.27205737607482,4.78138061219371));
#13955=CARTESIAN_POINT('Ctrl Pts',(3.66782587250124,-2.23786247288924,4.78508520854598));
#13956=CARTESIAN_POINT('Ctrl Pts',(3.61284256233116,-2.23361845303891,4.78878980489824));
#13957=CARTESIAN_POINT('Ctrl Pts',(3.55785925216109,-2.22937443318857,4.79249440125051));
#13958=CARTESIAN_POINT('Ctrl Pts',(3.50056411058224,-2.25508129667347,4.79619899760278));
#13959=CARTESIAN_POINT('Ctrl Pts',(3.46717858402372,-2.29897415165191,4.79990359395505));
#13960=CARTESIAN_POINT('Ctrl Pts',(3.44541647189655,-2.32758538921762,4.80231840808304));
#13961=CARTESIAN_POINT('Ctrl Pts',(3.43381352935432,-2.36392383491678,4.80473322221103));
#13962=CARTESIAN_POINT('Ctrl Pts',(3.43357088161517,-2.40012064492246,4.80714803633902));
#13963=CARTESIAN_POINT('Origin',(3.6,-2.4,4.7));
#13964=CARTESIAN_POINT('',(3.43314189260959,-2.4000500574177,4.87714803633902));
#13965=CARTESIAN_POINT('',(3.43333250832843,-2.39985412494998,4.85785196366098));
#13966=CARTESIAN_POINT('',(3.4334,-2.4,4.7));
#13967=CARTESIAN_POINT('Ctrl Pts',(3.43333250832843,-2.39985412494998,4.85785196366098));
#13968=CARTESIAN_POINT('Ctrl Pts',(3.43323384369475,-2.3890884237173,4.85713112672072));
#13969=CARTESIAN_POINT('Ctrl Pts',(3.43418764919828,-2.37834013090661,4.85641028978047));
#13970=CARTESIAN_POINT('Ctrl Pts',(3.4362574396422,-2.36781122023692,4.85568945284021));
#13971=CARTESIAN_POINT('Ctrl Pts',(3.44689471098651,-2.31370000328629,4.85198485648794));
#13972=CARTESIAN_POINT('Ctrl Pts',(3.48700781310569,-2.26538319325753,4.84828026013567));
#13973=CARTESIAN_POINT('Ctrl Pts',(3.53823875735816,-2.24497325223528,4.8445756637834));
#13974=CARTESIAN_POINT('Ctrl Pts',(3.58946970161063,-2.22456331121304,4.84087106743114));
#13975=CARTESIAN_POINT('Ctrl Pts',(3.65181848799641,-2.23206023919731,4.83716647107887));
#13976=CARTESIAN_POINT('Ctrl Pts',(3.69675084088435,-2.26403302458561,4.8334618747266));
#13977=CARTESIAN_POINT('Ctrl Pts',(3.74168319377229,-2.2960058099739,4.82975727837434));
#13978=CARTESIAN_POINT('Ctrl Pts',(3.76919911316239,-2.35245445276622,4.82605268202207));
#13979=CARTESIAN_POINT('Ctrl Pts',(3.76670578251992,-2.40754491150309,4.8223480856698));
#13980=CARTESIAN_POINT('Ctrl Pts',(3.76421245187744,-2.46263537023996,4.81864348931753));
#13981=CARTESIAN_POINT('Ctrl Pts',(3.73170987120238,-2.51636764492139,4.81493889296526));
#13982=CARTESIAN_POINT('Ctrl Pts',(3.68407303084285,-2.54415085535669,4.81123429661299));
#13983=CARTESIAN_POINT('Ctrl Pts',(3.63643619048332,-2.57193406579199,4.80752970026073));
#13984=CARTESIAN_POINT('Ctrl Pts',(3.57366509043931,-2.57376821198116,4.80382510390846));
#13985=CARTESIAN_POINT('Ctrl Pts',(3.52448728058231,-2.54881388652042,4.80012050755619));
#13986=CARTESIAN_POINT('Ctrl Pts',(3.47530947072531,-2.52385956105968,4.79641591120392));
#13987=CARTESIAN_POINT('Ctrl Pts',(3.43972495105532,-2.47211676394902,4.79271131485165));
#13988=CARTESIAN_POINT('Ctrl Pts',(3.43401917877726,-2.41726587968776,4.78900671849938));
#13989=CARTESIAN_POINT('Ctrl Pts',(3.43342633252912,-2.41156671411356,4.78862180021992));
#13990=CARTESIAN_POINT('Ctrl Pts',(3.43315605159773,-2.40583399421718,4.78823688194045));
#13991=CARTESIAN_POINT('Ctrl Pts',(3.43319592655187,-2.40009747379871,4.78785196366098));
#13992=CARTESIAN_POINT('Ctrl Pts',(3.43357088161517,-2.40012064492246,4.80714803633902));
#13993=CARTESIAN_POINT('Ctrl Pts',(3.43344128044335,-2.4194538108087,4.8084378185633));
#13994=CARTESIAN_POINT('Ctrl Pts',(3.43655249964156,-2.4387465714195,4.80972760078758));
#13995=CARTESIAN_POINT('Ctrl Pts',(3.44308755405667,-2.45679995496896,4.81101738301185));
#13996=CARTESIAN_POINT('Ctrl Pts',(3.46185796218633,-2.50865405683559,4.81472197936412));
#13997=CARTESIAN_POINT('Ctrl Pts',(3.50887468998386,-2.55028341409687,4.81842657571639));
#13998=CARTESIAN_POINT('Ctrl Pts',(3.56262026536972,-2.56263611534763,4.82213117206866));
#13999=CARTESIAN_POINT('Ctrl Pts',(3.61636584075558,-2.5749888165984,4.82583576842092));
#14000=CARTESIAN_POINT('Ctrl Pts',(3.67684026372979,-2.55806486183865,4.82954036477319));
#14001=CARTESIAN_POINT('Ctrl Pts',(3.71636707170489,-2.51960959492959,4.83324496112546));
#14002=CARTESIAN_POINT('Ctrl Pts',(3.75589387967999,-2.48115432802054,4.83694955747773));
#14003=CARTESIAN_POINT('Ctrl Pts',(3.77447307265599,-2.42116774896216,4.84065415383));
#14004=CARTESIAN_POINT('Ctrl Pts',(3.76360177761623,-2.36710305580748,4.84435875018227));
#14005=CARTESIAN_POINT('Ctrl Pts',(3.75273048257646,-2.3130383626528,4.84806334653453));
#14006=CARTESIAN_POINT('Ctrl Pts',(3.71240869952093,-2.26489555540181,4.8517679428868));
#14007=CARTESIAN_POINT('Ctrl Pts',(3.66108992110507,-2.24470746278141,4.85547253923907));
#14008=CARTESIAN_POINT('Ctrl Pts',(3.60977114268922,-2.224519370161,4.85917713559134));
#14009=CARTESIAN_POINT('Ctrl Pts',(3.54745536891304,-2.23228599217118,4.86288173194361));
#14010=CARTESIAN_POINT('Ctrl Pts',(3.50266176699964,-2.26445289020885,4.86658632829587));
#14011=CARTESIAN_POINT('Ctrl Pts',(3.4600933015382,-2.29502188733407,4.87010689764359));
#14012=CARTESIAN_POINT('Ctrl Pts',(3.43334940736011,-2.34762718854044,4.87362746699131));
#14013=CARTESIAN_POINT('Ctrl Pts',(3.43314189260959,-2.4000500574177,4.87714803633902));
#14014=CARTESIAN_POINT('Origin',(3.6,-2.4,4.7));
#14015=CARTESIAN_POINT('',(3.43342339329134,-2.39984780956037,4.94714803633902));
#14016=CARTESIAN_POINT('',(3.43366987537036,-2.39999366746476,4.92785196366098));
#14017=CARTESIAN_POINT('',(3.4334,-2.4,4.7));
#14018=CARTESIAN_POINT('Ctrl Pts',(3.43366987537036,-2.39999366746476,4.92785196366098));
#14019=CARTESIAN_POINT('Ctrl Pts',(3.43366057869757,-2.37257318362641,4.926025371501));
#14020=CARTESIAN_POINT('Ctrl Pts',(3.44006468998231,-2.34515678783965,4.92419877934102));
#14021=CARTESIAN_POINT('Ctrl Pts',(3.45290605548974,-2.32118937188857,4.92237218718104));
#14022=CARTESIAN_POINT('Ctrl Pts',(3.47895022498703,-2.27257994300186,4.91866759082877));
#14023=CARTESIAN_POINT('Ctrl Pts',(3.53147325377826,-2.23815747156893,4.9149629944765));
#14024=CARTESIAN_POINT('Ctrl Pts',(3.58643767991325,-2.23367559683213,4.91125839812423));
#14025=CARTESIAN_POINT('Ctrl Pts',(3.64140210604824,-2.22919372209532,4.90755380177196));
#14026=CARTESIAN_POINT('Ctrl Pts',(3.69880792952698,-2.25465244405464,4.9038492054197));
#14027=CARTESIAN_POINT('Ctrl Pts',(3.7323830497203,-2.29840043424344,4.90014460906743));
#14028=CARTESIAN_POINT('Ctrl Pts',(3.76595816991362,-2.34214842443224,4.89644001271516));
#14029=CARTESIAN_POINT('Ctrl Pts',(3.77570258682152,-2.40418568285053,4.89273541636289));
#14030=CARTESIAN_POINT('Ctrl Pts',(3.75715671279198,-2.45612050640859,4.88903082001062));
#14031=CARTESIAN_POINT('Ctrl Pts',(3.73861083876244,-2.50805532996664,4.88532622365835));
#14032=CARTESIAN_POINT('Ctrl Pts',(3.69177467379546,-2.54988771866446,4.88162162730609));
#14033=CARTESIAN_POINT('Ctrl Pts',(3.63808305436706,-2.56247284260842,4.87791703095382));
#14034=CARTESIAN_POINT('Ctrl Pts',(3.58439143493865,-2.57505796655237,4.87421243460155));
#14035=CARTESIAN_POINT('Ctrl Pts',(3.52384436104883,-2.55839582574246,4.87050783824928));
#14036=CARTESIAN_POINT('Ctrl Pts',(3.48415154438863,-2.52011194340126,4.86680324189701));
#14037=CARTESIAN_POINT('Ctrl Pts',(3.45218211937245,-2.4892773035642,4.863819482485));
#14038=CARTESIAN_POINT('Ctrl Pts',(3.4337409107187,-2.4444165781012,4.86083572307299));
#14039=CARTESIAN_POINT('Ctrl Pts',(3.43333250832843,-2.39985412494998,4.85785196366098));
#14040=CARTESIAN_POINT('Ctrl Pts',(3.43314189260959,-2.4000500574177,4.87714803633902));
#14041=CARTESIAN_POINT('Ctrl Pts',(3.43313104541013,-2.4027903026953,4.87733206334358));
#14042=CARTESIAN_POINT('Ctrl Pts',(3.43319270505025,-2.40553004950279,4.87751609034813));
#14043=CARTESIAN_POINT('Ctrl Pts',(3.43332840145004,-2.40826612443654,4.87770011735268));
#14044=CARTESIAN_POINT('Ctrl Pts',(3.43606006786446,-2.46334528656136,4.88140471370495));
#14045=CARTESIAN_POINT('Ctrl Pts',(3.46879483074392,-2.51693643674581,4.88510931005721));
#14046=CARTESIAN_POINT('Ctrl Pts',(3.51655144023777,-2.54451328122398,4.88881390640948));
#14047=CARTESIAN_POINT('Ctrl Pts',(3.56430804973163,-2.57209012570216,4.89251850276175));
#14048=CARTESIAN_POINT('Ctrl Pts',(3.62708650583988,-2.57365266447405,4.89622309911402));
#14049=CARTESIAN_POINT('Ctrl Pts',(3.67615589214678,-2.54848579281353,4.89992769546629));
#14050=CARTESIAN_POINT('Ctrl Pts',(3.72522527845368,-2.52331892115301,4.90363229181856));
#14051=CARTESIAN_POINT('Ctrl Pts',(3.76058559495924,-2.47142263906009,4.90733688817082));
#14052=CARTESIAN_POINT('Ctrl Pts',(3.76605399230753,-2.41654757430046,4.91104148452309));
#14053=CARTESIAN_POINT('Ctrl Pts',(3.77152238965583,-2.36167250954082,4.91474608087536));
#14054=CARTESIAN_POINT('Ctrl Pts',(3.74709886784687,-2.30381866211447,4.91845067722763));
#14055=CARTESIAN_POINT('Ctrl Pts',(3.70396099012833,-2.26946317336186,4.9221552735799));
#14056=CARTESIAN_POINT('Ctrl Pts',(3.6608231124098,-2.23510768460924,4.92585986993216));
#14057=CARTESIAN_POINT('Ctrl Pts',(3.5989708787817,-2.22425055453036,4.92956446628443));
#14058=CARTESIAN_POINT('Ctrl Pts',(3.54671131468788,-2.24186061024559,4.9332690626367));
#14059=CARTESIAN_POINT('Ctrl Pts',(3.49445175059407,-2.25947066596082,4.93697365898896));
#14060=CARTESIAN_POINT('Ctrl Pts',(3.45178485603454,-2.30554790747016,4.94067825534124));
#14061=CARTESIAN_POINT('Ctrl Pts',(3.43823737724635,-2.35900482396987,4.94438285169351));
#14062=CARTESIAN_POINT('Ctrl Pts',(3.43486667440692,-2.37230526038685,4.94530457990868));
#14063=CARTESIAN_POINT('Ctrl Pts',(3.43329860172231,-2.38606253373953,4.94622630812385));
#14064=CARTESIAN_POINT('Ctrl Pts',(3.43342339329134,-2.39984780956037,4.94714803633902));
#14065=CARTESIAN_POINT('Origin',(3.6,-2.4,4.7));
#14066=CARTESIAN_POINT('',(3.43365998837939,-2.40004261214837,5.01714803633902));
#14067=CARTESIAN_POINT('',(3.4333557533513,-2.40014916294441,4.99785196366098));
#14068=CARTESIAN_POINT('',(3.4334,-2.4,4.7));
#14069=CARTESIAN_POINT('Ctrl Pts',(3.4333557533513,-2.40014916294441,4.99785196366098));
#14070=CARTESIAN_POINT('Ctrl Pts',(3.43376006878861,-2.35633883086337,4.99491961628128));
#14071=CARTESIAN_POINT('Ctrl Pts',(3.45150379646176,-2.31223873171809,4.99198726890157));
#14072=CARTESIAN_POINT('Ctrl Pts',(3.48249984549986,-2.28150334481789,4.98905492152186));
#14073=CARTESIAN_POINT('Ctrl Pts',(3.5216588656746,-2.24267363351424,4.98535032516959));
#14074=CARTESIAN_POINT('Ctrl Pts',(3.58196947066853,-2.22517489033693,4.98164572881732));
#14075=CARTESIAN_POINT('Ctrl Pts',(3.63583017024712,-2.23701551447795,4.97794113246505));
#14076=CARTESIAN_POINT('Ctrl Pts',(3.68969086982571,-2.24885613861896,4.97423653611278));
#14077=CARTESIAN_POINT('Ctrl Pts',(3.73710166398897,-2.29003613007831,4.97053193976052));
#14078=CARTESIAN_POINT('Ctrl Pts',(3.75636473388799,-2.34170923218213,4.96682734340825));
#14079=CARTESIAN_POINT('Ctrl Pts',(3.775627803787,-2.39338233428594,4.96312274705599));
#14080=CARTESIAN_POINT('Ctrl Pts',(3.76674314942177,-2.45554854703422,4.95941815070372));
#14081=CARTESIAN_POINT('Ctrl Pts',(3.73377688327324,-2.49975715069431,4.95571355435145));
#14082=CARTESIAN_POINT('Ctrl Pts',(3.7008106171247,-2.54396575435439,4.95200895799918));
#14083=CARTESIAN_POINT('Ctrl Pts',(3.64376273919286,-2.57021674892629,4.94830436164691));
#14084=CARTESIAN_POINT('Ctrl Pts',(3.58874153428106,-2.56649621787192,4.94459976529464));
#14085=CARTESIAN_POINT('Ctrl Pts',(3.53372032936927,-2.56277568681755,4.94089516894238));
#14086=CARTESIAN_POINT('Ctrl Pts',(3.48072579747752,-2.52908363013692,4.93719057259011));
#14087=CARTESIAN_POINT('Ctrl Pts',(3.45401118663332,-2.48083940862635,4.93348597623784));
#14088=CARTESIAN_POINT('Ctrl Pts',(3.4404685098097,-2.45638253353524,4.93160797204555));
#14089=CARTESIAN_POINT('Ctrl Pts',(3.43367943371122,-2.42818593979086,4.92972996785327));
#14090=CARTESIAN_POINT('Ctrl Pts',(3.43366987537036,-2.39999366746476,4.92785196366098));
#14091=CARTESIAN_POINT('Ctrl Pts',(3.43342339329134,-2.39984780956037,4.94714803633902));
#14092=CARTESIAN_POINT('Ctrl Pts',(3.43380016214308,-2.44146810957007,4.94993090447612));
#14093=CARTESIAN_POINT('Ctrl Pts',(3.44960819947038,-2.48334366548894,4.95271377261321));
#14094=CARTESIAN_POINT('Ctrl Pts',(3.47782660292827,-2.51367238728015,4.95549664075031));
#14095=CARTESIAN_POINT('Ctrl Pts',(3.51539137041525,-2.55404644260063,4.95920123710258));
#14096=CARTESIAN_POINT('Ctrl Pts',(3.57494896840608,-2.57395796175148,4.96290583345484));
#14097=CARTESIAN_POINT('Ctrl Pts',(3.62924252448225,-2.56429432528282,4.96661042980711));
#14098=CARTESIAN_POINT('Ctrl Pts',(3.68353608055842,-2.55463068881416,4.97031502615938));
#14099=CARTESIAN_POINT('Ctrl Pts',(3.73256559471993,-2.51539189672599,4.97401962251165));
#14100=CARTESIAN_POINT('Ctrl Pts',(3.75389243176138,-2.46453580432507,4.97772421886392));
#14101=CARTESIAN_POINT('Ctrl Pts',(3.77521926880282,-2.41367971192415,4.98142881521619));
#14102=CARTESIAN_POINT('Ctrl Pts',(3.7688434287242,-2.35120631921049,4.98513341156845));
#14103=CARTESIAN_POINT('Ctrl Pts',(3.73768285095733,-2.30570692939164,4.98883800792072));
#14104=CARTESIAN_POINT('Ctrl Pts',(3.70652227319045,-2.26020753957279,4.99254260427299));
#14105=CARTESIAN_POINT('Ctrl Pts',(3.65057695773533,-2.23168215264876,4.99624720062526));
#14106=CARTESIAN_POINT('Ctrl Pts',(3.59545059530862,-2.23318557212546,4.99995179697752));
#14107=CARTESIAN_POINT('Ctrl Pts',(3.5403242328819,-2.23468899160217,5.00365639332979));
#14108=CARTESIAN_POINT('Ctrl Pts',(3.48601682348359,-2.2662212174796,5.00736098968206));
#14109=CARTESIAN_POINT('Ctrl Pts',(3.4573824612349,-2.31335135092863,5.01106558603433));
#14110=CARTESIAN_POINT('Ctrl Pts',(3.44171120056098,-2.3391451367466,5.01309306946923));
#14111=CARTESIAN_POINT('Ctrl Pts',(3.43372965513495,-2.36961088327844,5.01512055290413));
#14112=CARTESIAN_POINT('Ctrl Pts',(3.43365998837939,-2.40004261214837,5.01714803633902));
#14113=CARTESIAN_POINT('Origin',(3.6,-2.4,4.7));
#14114=CARTESIAN_POINT('',(3.43326718206005,-2.40013003210005,5.08714803633902));
#14115=CARTESIAN_POINT('',(3.43317939237559,-2.39991359865598,5.06785196366098));
#14116=CARTESIAN_POINT('',(3.4334,-2.4,4.7));
#14117=CARTESIAN_POINT('Ctrl Pts',(3.43317939237559,-2.39991359865598,5.06785196366098));
#14118=CARTESIAN_POINT('Ctrl Pts',(3.43314802801357,-2.39494457971841,5.06751845741381));
#14119=CARTESIAN_POINT('Ctrl Pts',(3.43335080279482,-2.38997815623028,5.06718495116665));
#14120=CARTESIAN_POINT('Ctrl Pts',(3.43379605546717,-2.38503356765244,5.06685144491949));
#14121=CARTESIAN_POINT('Ctrl Pts',(3.43874193411214,-2.33010894490636,5.06314684856722));
#14122=CARTESIAN_POINT('Ctrl Pts',(3.47360673801625,-2.27787849376484,5.05944225221495));
#14123=CARTESIAN_POINT('Ctrl Pts',(3.52243437581894,-2.25224575672994,5.05573765586269));
#14124=CARTESIAN_POINT('Ctrl Pts',(3.57126201362163,-2.22661301969504,5.05203305951042));
#14125=CARTESIAN_POINT('Ctrl Pts',(3.63405248532289,-2.22757799676674,5.04832846315815));
#14126=CARTESIAN_POINT('Ctrl Pts',(3.68206938357278,-2.25469907052132,5.04462386680588));
#14127=CARTESIAN_POINT('Ctrl Pts',(3.73008628182266,-2.28182014427589,5.04091927045361));
#14128=CARTESIAN_POINT('Ctrl Pts',(3.76332960662116,-2.33509731471334,5.03721467410135));
#14129=CARTESIAN_POINT('Ctrl Pts',(3.7665853578407,-2.39014797778335,5.03351007774908));
#14130=CARTESIAN_POINT('Ctrl Pts',(3.76984110906023,-2.44519864085336,5.02980548139681));
#14131=CARTESIAN_POINT('Ctrl Pts',(3.7431092867008,-2.50202279655593,5.02610088504454));
#14132=CARTESIAN_POINT('Ctrl Pts',(3.69862386285843,-2.53461455026518,5.02239628869228));
#14133=CARTESIAN_POINT('Ctrl Pts',(3.65413843901607,-2.56720630397444,5.01869169234001));
#14134=CARTESIAN_POINT('Ctrl Pts',(3.59189941369078,-2.57556565569037,5.01498709598774));
#14135=CARTESIAN_POINT('Ctrl Pts',(3.54039082873623,-2.55586689947754,5.01128249963547));
#14136=CARTESIAN_POINT('Ctrl Pts',(3.48888224378167,-2.53616814326471,5.0075779032832));
#14137=CARTESIAN_POINT('Ctrl Pts',(3.44810409919785,-2.48841127912311,5.00387330693093));
#14138=CARTESIAN_POINT('Ctrl Pts',(3.43671874458371,-2.43445250733732,5.00016871057866));
#14139=CARTESIAN_POINT('Ctrl Pts',(3.43434538792972,-2.42320442465572,4.9993964616061));
#14140=CARTESIAN_POINT('Ctrl Pts',(3.43324927477267,-2.41168684233781,4.99862421263354));
#14141=CARTESIAN_POINT('Ctrl Pts',(3.4333557533513,-2.40014916294441,4.99785196366098));
#14142=CARTESIAN_POINT('Ctrl Pts',(3.43365998837939,-2.40004261214837,5.01714803633902));
#14143=CARTESIAN_POINT('Ctrl Pts',(3.43360236077384,-2.42521541736454,5.01882514925639));
#14144=CARTESIAN_POINT('Ctrl Pts',(3.43895837597341,-2.45036494625428,5.02050226217376));
#14145=CARTESIAN_POINT('Ctrl Pts',(3.44985377805168,-2.47282762403026,5.02217937509113));
#14146=CARTESIAN_POINT('Ctrl Pts',(3.47392077221621,-2.52244572266223,5.0258839714434));
#14147=CARTESIAN_POINT('Ctrl Pts',(3.52501607564434,-2.55895387890556,5.02958856779567));
#14148=CARTESIAN_POINT('Ctrl Pts',(3.57975563405926,-2.56564394064586,5.03329316414793));
#14149=CARTESIAN_POINT('Ctrl Pts',(3.63449519247418,-2.57233400238615,5.0369977605002));
#14150=CARTESIAN_POINT('Ctrl Pts',(3.69287900587587,-2.54920596962341,5.04070235685248));
#14151=CARTESIAN_POINT('Ctrl Pts',(3.72818738886538,-2.5068444924534,5.04440695320474));
#14152=CARTESIAN_POINT('Ctrl Pts',(3.76349577185488,-2.4644830152834,5.04811154955701));
#14153=CARTESIAN_POINT('Ctrl Pts',(3.77572872443219,-2.40288809370614,5.05181614590928));
#14154=CARTESIAN_POINT('Ctrl Pts',(3.75928777076399,-2.35024904339754,5.05552074226154));
#14155=CARTESIAN_POINT('Ctrl Pts',(3.74284681709578,-2.29760999308894,5.05922533861381));
#14156=CARTESIAN_POINT('Ctrl Pts',(3.69773195718207,-2.25392681404901,5.06292993496608));
#14157=CARTESIAN_POINT('Ctrl Pts',(3.6445902539118,-2.239191259641,5.06663453131835));
#14158=CARTESIAN_POINT('Ctrl Pts',(3.59144855064154,-2.22445570523299,5.07033912767062));
#14159=CARTESIAN_POINT('Ctrl Pts',(3.53028000401472,-2.2386677754569,5.07404372402289));
#14160=CARTESIAN_POINT('Ctrl Pts',(3.48907876340423,-2.27532343849,5.07774832037515));
#14161=CARTESIAN_POINT('Ctrl Pts',(3.45423196569032,-2.3063257203596,5.08088155902977));
#14162=CARTESIAN_POINT('Ctrl Pts',(3.43366833898609,-2.35338253026132,5.0840147976844));
#14163=CARTESIAN_POINT('Ctrl Pts',(3.43326718206005,-2.40013003210005,5.08714803633902));
#14164=CARTESIAN_POINT('Origin',(3.6,-2.4,4.7));
#14165=CARTESIAN_POINT('',(3.43325215766083,-2.39987843114813,5.15714803633902));
#14166=CARTESIAN_POINT('',(3.43361559198215,-2.39990578567643,5.13785196366098));
#14167=CARTESIAN_POINT('',(3.4334,-2.4,4.7));
#14168=CARTESIAN_POINT('',(3.72690708798524,-2.29206413469515,5.2));
#14169=CARTESIAN_POINT('Ctrl Pts',(3.43325215766083,-2.39987843114813,5.15714803633902));
#14170=CARTESIAN_POINT('Ctrl Pts',(3.43364568926707,-2.44715561674071,5.16031823516921));
#14171=CARTESIAN_POINT('Ctrl Pts',(3.45475450700198,-2.49473162154361,5.1634884339994));
#14172=CARTESIAN_POINT('Ctrl Pts',(3.49032381647516,-2.52575978121339,5.16665863282959));
#14173=CARTESIAN_POINT('Ctrl Pts',(3.53188901196771,-2.56201832942672,5.17036322918186));
#14174=CARTESIAN_POINT('Ctrl Pts',(3.59320078561411,-2.575679906312,5.17406782553413));
#14175=CARTESIAN_POINT('Ctrl Pts',(3.64619137793262,-2.5603849196725,5.17777242188639));
#14176=CARTESIAN_POINT('Ctrl Pts',(3.69918197025112,-2.545089933033,5.18147701823866));
#14177=CARTESIAN_POINT('Ctrl Pts',(3.74385138124173,-2.50083838286872,5.18518161459093));
#14178=CARTESIAN_POINT('Ctrl Pts',(3.75975547145412,-2.44813183978448,5.1888862109432));
#14179=CARTESIAN_POINT('Ctrl Pts',(3.7756595616665,-2.39542529670025,5.19259080729546));
#14180=CARTESIAN_POINT('Ctrl Pts',(3.76279833110066,-2.33426376069605,5.19629540364773));
#14181=CARTESIAN_POINT('Ctrl Pts',(3.72690708798524,-2.29206413469515,5.2));
#14182=CARTESIAN_POINT('',(3.47285247305911,-2.29187966783456,5.2));
#14183=CARTESIAN_POINT('Origin',(3.6,-2.4,5.2));
#14184=CARTESIAN_POINT('Ctrl Pts',(3.47285232078578,-2.29187955100914,5.2));
#14185=CARTESIAN_POINT('Ctrl Pts',(3.50793811899511,-2.25072740472549,5.19636770818144));
#14186=CARTESIAN_POINT('Ctrl Pts',(3.5649358740211,-2.22812243199181,5.19273541636289));
#14187=CARTESIAN_POINT('Ctrl Pts',(3.61867624862122,-2.23418211249055,5.18910312454433));
#14188=CARTESIAN_POINT('Ctrl Pts',(3.67348638108252,-2.24036241721079,5.18539852819207));
#14189=CARTESIAN_POINT('Ctrl Pts',(3.72490815931237,-2.27635993281072,5.1816939318398));
#14190=CARTESIAN_POINT('Ctrl Pts',(3.74944162123119,-2.32574103985171,5.17798933548753));
#14191=CARTESIAN_POINT('Ctrl Pts',(3.77397508315002,-2.37512214689269,5.17428473913527));
#14192=CARTESIAN_POINT('Ctrl Pts',(3.77162022875783,-2.43788684537472,5.17058014278299));
#14193=CARTESIAN_POINT('Ctrl Pts',(3.74343805414309,-2.48529019582313,5.16687554643072));
#14194=CARTESIAN_POINT('Ctrl Pts',(3.71525587952836,-2.53269354627153,5.16317095007846));
#14195=CARTESIAN_POINT('Ctrl Pts',(3.66124638469108,-2.5647355486863,5.15946635372619));
#14196=CARTESIAN_POINT('Ctrl Pts',(3.60613566942556,-2.56676214228893,5.15576175737392));
#14197=CARTESIAN_POINT('Ctrl Pts',(3.55102495416005,-2.56878873589157,5.15205716102166));
#14198=CARTESIAN_POINT('Ctrl Pts',(3.49481301846629,-2.54079992068208,5.14835256466939));
#14199=CARTESIAN_POINT('Ctrl Pts',(3.46322140367409,-2.49559987057215,5.14464796831712));
#14200=CARTESIAN_POINT('Ctrl Pts',(3.44390335110665,-2.46796035452279,5.14238263343174));
#14201=CARTESIAN_POINT('Ctrl Pts',(3.43379142096037,-2.43388514918463,5.14011729854636));
#14202=CARTESIAN_POINT('Ctrl Pts',(3.43361559198215,-2.39990578567643,5.13785196366098));
#14203=CARTESIAN_POINT('Origin',(3.6,-2.4,5.35459252805377));
#14204=CARTESIAN_POINT('',(3.39427732444531,-2.39988044480691,4.34540747194623));
#14205=CARTESIAN_POINT('',(3.39483887958286,-2.40008013132228,4.33959252805377));
#14206=CARTESIAN_POINT('',(3.394525,-2.39999999999999,5.35459252805377));
#14207=CARTESIAN_POINT('',(3.78826275096636,-2.48232321801033,4.3));
#14208=CARTESIAN_POINT('Ctrl Pts',(3.39483887958286,-2.40008013132228,4.33959252805377));
#14209=CARTESIAN_POINT('Ctrl Pts',(3.39495668787724,-2.361520075325,4.33750880775932));
#14210=CARTESIAN_POINT('Ctrl Pts',(3.4239416532562,-2.25423614055743,4.3317204911126));
#14211=CARTESIAN_POINT('Ctrl Pts',(3.59702530195382,-2.15700945407857,4.32222757811361));
#14212=CARTESIAN_POINT('Ctrl Pts',(3.80250230755732,-2.26611609660926,4.31111378905681));
#14213=CARTESIAN_POINT('Ctrl Pts',(3.81563717950601,-2.41972137435598,4.30370459635227));
#14214=CARTESIAN_POINT('Ctrl Pts',(3.78826275096636,-2.48232321801033,4.3));
#14215=CARTESIAN_POINT('',(3.72235839003881,-2.56553532314028,4.3));
#14216=CARTESIAN_POINT('Origin',(3.6,-2.4,4.3));
#14217=CARTESIAN_POINT('Ctrl Pts',(3.39427732444531,-2.39988044480691,4.34540747194623));
#14218=CARTESIAN_POINT('Ctrl Pts',(3.39422705601106,-2.39271640856816,4.34501772883951));
#14219=CARTESIAN_POINT('Ctrl Pts',(3.39781628789546,-2.31750701228878,4.34092338938053));
#14220=CARTESIAN_POINT('Ctrl Pts',(3.49037003077072,-2.18326698967564,4.33312445356928));
#14221=CARTESIAN_POINT('Ctrl Pts',(3.72265543153543,-2.19039239422561,4.32201066451247));
#14222=CARTESIAN_POINT('Ctrl Pts',(3.84179827282652,-2.38799091139141,4.31096917998938));
#14223=CARTESIAN_POINT('Ctrl Pts',(3.77594285680537,-2.52582029152411,4.30363229181855));
#14224=CARTESIAN_POINT('Ctrl Pts',(3.72235852099786,-2.56553552032367,4.3));
#14225=CARTESIAN_POINT('Origin',(3.6,-2.4,5.35459252805377));
#14226=CARTESIAN_POINT('',(3.39480735688311,-2.3998973457609,4.41540747194623));
#14227=CARTESIAN_POINT('',(3.39433274578554,-2.4001497810388,4.40959252805377));
#14228=CARTESIAN_POINT('',(3.394525,-2.39999999999999,5.35459252805377));
#14229=CARTESIAN_POINT('Ctrl Pts',(3.39433274578554,-2.4001497810388,4.40959252805377));
#14230=CARTESIAN_POINT('Ctrl Pts',(3.39481384891428,-2.34148051031483,4.40640305253959));
#14231=CARTESIAN_POINT('Ctrl Pts',(3.45186170282621,-2.21384965704481,4.39950898067315));
#14232=CARTESIAN_POINT('Ctrl Pts',(3.66843098386609,-2.16697244123634,4.38891031245443));
#14233=CARTESIAN_POINT('Ctrl Pts',(3.83289206448147,-2.33111753521892,4.37779652339763));
#14234=CARTESIAN_POINT('Ctrl Pts',(3.7841810615649,-2.55829573402952,4.36668273434082));
#14235=CARTESIAN_POINT('Ctrl Pts',(3.56689372435994,-2.6406156849541,4.35556894528403));
#14236=CARTESIAN_POINT('Ctrl Pts',(3.4149557748622,-2.52850415334516,4.34653887652167));
#14237=CARTESIAN_POINT('Ctrl Pts',(3.39474723933523,-2.4300750743674,4.34121340411158));
#14238=CARTESIAN_POINT('Ctrl Pts',(3.39483887958286,-2.40008013132228,4.33959252805377));
#14239=CARTESIAN_POINT('Ctrl Pts',(3.39480735688311,-2.3998973457609,4.41540747194623));
#14240=CARTESIAN_POINT('Ctrl Pts',(3.39468219270667,-2.3722256242847,4.41391197361979));
#14241=CARTESIAN_POINT('Ctrl Pts',(3.4127838411683,-2.27616341542302,4.40871187894107));
#14242=CARTESIAN_POINT('Ctrl Pts',(3.55878722400007,-2.16065655916503,4.3998071879101));
#14243=CARTESIAN_POINT('Ctrl Pts',(3.77873474447839,-2.23556893008468,4.38869339885329));
#14244=CARTESIAN_POINT('Ctrl Pts',(3.83508286096032,-2.4609855401145,4.37757960979649));
#14245=CARTESIAN_POINT('Ctrl Pts',(3.67625990251943,-2.63058416437082,4.36646582073969));
#14246=CARTESIAN_POINT('Ctrl Pts',(3.45564722516575,-2.59057499098668,4.3557417747896));
#14247=CARTESIAN_POINT('Ctrl Pts',(3.39470486884463,-2.46081219284274,4.34872232519178));
#14248=CARTESIAN_POINT('Ctrl Pts',(3.39427732444531,-2.39988044480691,4.34540747194623));
#14249=CARTESIAN_POINT('Origin',(3.6,-2.4,5.35459252805377));
#14250=CARTESIAN_POINT('',(3.39465010821578,-2.400176527643,4.48540747194623));
#14251=CARTESIAN_POINT('',(3.39437120606287,-2.39983660975581,4.47959252805377));
#14252=CARTESIAN_POINT('',(3.394525,-2.39999999999999,5.35459252805377));
#14253=CARTESIAN_POINT('Ctrl Pts',(3.39437120606287,-2.39983660975581,4.47959252805376));
#14254=CARTESIAN_POINT('Ctrl Pts',(3.39427673427304,-2.3889667776849,4.47900189367213));
#14255=CARTESIAN_POINT('Ctrl Pts',(3.40000383699504,-2.31001856010007,4.47470666293823));
#14256=CARTESIAN_POINT('Ctrl Pts',(3.50226148839652,-2.17766948860297,4.46670683585206));
#14257=CARTESIAN_POINT('Ctrl Pts',(3.73378446004359,-2.19730463405286,4.45559304679526));
#14258=CARTESIAN_POINT('Ctrl Pts',(3.84285302402677,-2.40246926900864,4.44447925773845));
#14259=CARTESIAN_POINT('Ctrl Pts',(3.72963540924699,-2.60537350906572,4.43336546868165));
#14260=CARTESIAN_POINT('Ctrl Pts',(3.49776113780875,-2.62029753773771,4.42225167962485));
#14261=CARTESIAN_POINT('Ctrl Pts',(3.39915518843152,-2.48716469789757,4.41432736608222));
#14262=CARTESIAN_POINT('Ctrl Pts',(3.3942550445316,-2.40962524613366,4.41010764889186));
#14263=CARTESIAN_POINT('Ctrl Pts',(3.39433274578554,-2.4001497810388,4.40959252805377));
#14264=CARTESIAN_POINT('Ctrl Pts',(3.39465010821578,-2.400176527643,4.48540747194623));
#14265=CARTESIAN_POINT('Ctrl Pts',(3.3950436881435,-2.35213729673001,4.48280621840006));
#14266=CARTESIAN_POINT('Ctrl Pts',(3.43581223913156,-2.23508079066125,4.47650036850162));
#14267=CARTESIAN_POINT('Ctrl Pts',(3.63081864021225,-2.15909778094929,4.46648992225093));
#14268=CARTESIAN_POINT('Ctrl Pts',(3.81910984016012,-2.29524053287965,4.45537613319411));
#14269=CARTESIAN_POINT('Ctrl Pts',(3.80684729577664,-2.52727079162485,4.44426234413733));
#14270=CARTESIAN_POINT('Ctrl Pts',(3.60525512132335,-2.64280869447754,4.4331485550805));
#14271=CARTESIAN_POINT('Ctrl Pts',(3.42662678112532,-2.55045981030713,4.42353026435015));
#14272=CARTESIAN_POINT('Ctrl Pts',(3.39499224504393,-2.44077304866432,4.41761656997206));
#14273=CARTESIAN_POINT('Ctrl Pts',(3.39480735688311,-2.3998973457609,4.41540747194623));
#14274=CARTESIAN_POINT('Origin',(3.6,-2.4,5.35459252805377));
#14275=CARTESIAN_POINT('',(3.39418406677318,-2.39999917227821,4.55540747194623));
#14276=CARTESIAN_POINT('',(3.39484823116951,-2.39995310238382,4.54959252805377));
#14277=CARTESIAN_POINT('',(3.394525,-2.39999999999999,5.35459252805377));
#14278=CARTESIAN_POINT('Ctrl Pts',(3.39484823116951,-2.39995310238382,4.54959252805377));
#14279=CARTESIAN_POINT('Ctrl Pts',(3.3947841219125,-2.36854855723416,4.54789613845241));
#14280=CARTESIAN_POINT('Ctrl Pts',(3.41632348134282,-2.26864576454574,4.54249515249878));
#14281=CARTESIAN_POINT('Ctrl Pts',(3.57178888017207,-2.15877849637109,4.53338957019289));
#14282=CARTESIAN_POINT('Ctrl Pts',(3.78736362800739,-2.2454731342224,4.52227578113608));
#14283=CARTESIAN_POINT('Ctrl Pts',(3.83144232268012,-2.47360796667095,4.51116199207928));
#14284=CARTESIAN_POINT('Ctrl Pts',(3.66367923386702,-2.6343685886554,4.50004820302247));
#14285=CARTESIAN_POINT('Ctrl Pts',(3.44964305628728,-2.58346600654441,4.48952504834731));
#14286=CARTESIAN_POINT('Ctrl Pts',(3.39486928333363,-2.45714489513262,4.4827064900244));
#14287=CARTESIAN_POINT('Ctrl Pts',(3.39437120606287,-2.39983660975581,4.47959252805376));
#14288=CARTESIAN_POINT('Ctrl Pts',(3.39418406845602,-2.39999917228229,4.55540747194623));
#14289=CARTESIAN_POINT('Ctrl Pts',(3.39418406581063,-2.39995488126817,4.55540505953261));
#14290=CARTESIAN_POINT('Ctrl Pts',(3.39420413582033,-2.33189558582108,4.55169805076672));
#14291=CARTESIAN_POINT('Ctrl Pts',(3.46841583417461,-2.19586946879708,4.54428644564855));
#14292=CARTESIAN_POINT('Ctrl Pts',(3.70013762796088,-2.17873969637961,4.53317265659175));
#14293=CARTESIAN_POINT('Ctrl Pts',(3.84020231541317,-2.36413198929513,4.52205886753494));
#14294=CARTESIAN_POINT('Ctrl Pts',(3.7604070991348,-2.58235467884591,4.51094507847814));
#14295=CARTESIAN_POINT('Ctrl Pts',(3.53378944658573,-2.63366606347461,4.49983128942134));
#14296=CARTESIAN_POINT('Ctrl Pts',(3.40663179333208,-2.50914981953724,4.4913187539107));
#14297=CARTESIAN_POINT('Ctrl Pts',(3.39448316809474,-2.42055275737136,4.48651081475233));
#14298=CARTESIAN_POINT('Ctrl Pts',(3.39465010821578,-2.400176527643,4.48540747194623));
#14299=CARTESIAN_POINT('Origin',(3.6,-2.4,5.35459252805377));
#14300=CARTESIAN_POINT('',(3.39465252302706,-2.39982399270837,4.62540747194623));
#14301=CARTESIAN_POINT('',(3.39454319301877,-2.40018789160095,4.61959252805377));
#14302=CARTESIAN_POINT('',(3.394525,-2.39999999999999,5.35459252805377));
#14303=CARTESIAN_POINT('Ctrl Pts',(3.39454319301877,-2.40018789160095,4.61959252805377));
#14304=CARTESIAN_POINT('Ctrl Pts',(3.39501369486734,-2.34850703974388,4.61679038323268));
#14305=CARTESIAN_POINT('Ctrl Pts',(3.44097935155591,-2.22775547868952,4.61028364205933));
#14306=CARTESIAN_POINT('Ctrl Pts',(3.64379902793915,-2.16111650041238,4.60007230453371));
#14307=CARTESIAN_POINT('Ctrl Pts',(3.82445363439269,-2.30724091831967,4.58895851547691));
#14308=CARTESIAN_POINT('Ctrl Pts',(3.79966328381548,-2.53826877567792,4.57784472642011));
#14309=CARTESIAN_POINT('Ctrl Pts',(3.59211886521387,-2.64273765452468,4.5667309373633));
#14310=CARTESIAN_POINT('Ctrl Pts',(3.42236627541046,-2.54299330864641,4.55731353790785));
#14311=CARTESIAN_POINT('Ctrl Pts',(3.39492412449178,-2.43713018689806,4.55160073480468));
#14312=CARTESIAN_POINT('Ctrl Pts',(3.39484823116951,-2.39995310238382,4.54959252805377));
#14313=CARTESIAN_POINT('Ctrl Pts',(3.39465252302706,-2.39982399270837,4.62540747194623));
#14314=CARTESIAN_POINT('Ctrl Pts',(3.39448549072207,-2.37935805029673,4.62429930431288));
#14315=CARTESIAN_POINT('Ctrl Pts',(3.40670160391397,-2.29066952405396,4.61948654032727));
#14316=CARTESIAN_POINT('Ctrl Pts',(3.53409308711521,-2.16624811163355,4.61096917998937));
#14317=CARTESIAN_POINT('Ctrl Pts',(3.76064388390312,-2.21785387995996,4.59985539093258));
#14318=CARTESIAN_POINT('Ctrl Pts',(3.8401555119317,-2.4361800576391,4.58874160187577));
#14319=CARTESIAN_POINT('Ctrl Pts',(3.69985007633495,-2.62139021824623,4.57762781281896));
#14320=CARTESIAN_POINT('Ctrl Pts',(3.4682010273,-2.60396318498582,4.56651643617578));
#14321=CARTESIAN_POINT('Ctrl Pts',(3.39418812817678,-2.46796988817124,4.55910965588488));
#14322=CARTESIAN_POINT('Ctrl Pts',(3.39418406845602,-2.39999917228229,4.55540747194623));
#14323=CARTESIAN_POINT('Origin',(3.6,-2.4,5.35459252805377));
#14324=CARTESIAN_POINT('',(3.39480597714356,-2.40010391086475,4.69540747194623));
#14325=CARTESIAN_POINT('',(3.39421139045774,-2.39993212258527,4.68959252805377));
#14326=CARTESIAN_POINT('',(3.394525,-2.39999999999999,5.35459252805377));
#14327=CARTESIAN_POINT('Ctrl Pts',(3.39421139045774,-2.39993212258527,4.68959252805377));
#14328=CARTESIAN_POINT('Ctrl Pts',(3.39419531835948,-2.39619821368606,4.68938922436523));
#14329=CARTESIAN_POINT('Ctrl Pts',(3.3959796089401,-2.32444075084805,4.68548132432442));
#14330=CARTESIAN_POINT('Ctrl Pts',(3.47964553863801,-2.18905336016944,4.67786882793135));
#14331=CARTESIAN_POINT('Ctrl Pts',(3.71195459122784,-2.18447772567898,4.66675503887453));
#14332=CARTESIAN_POINT('Ctrl Pts',(3.84179033681535,-2.37717207306315,4.65564124981774));
#14333=CARTESIAN_POINT('Ctrl Pts',(3.75031264502696,-2.59076108085938,4.64452746076093));
#14334=CARTESIAN_POINT('Ctrl Pts',(3.52125208458385,-2.6297443079663,4.63341367170413));
#14335=CARTESIAN_POINT('Ctrl Pts',(3.40385053605922,-2.50163131684181,4.6251020274684));
#14336=CARTESIAN_POINT('Ctrl Pts',(3.39439166440737,-2.4168320934068,4.62049497958495));
#14337=CARTESIAN_POINT('Ctrl Pts',(3.39454319301877,-2.40018789160095,4.61959252805377));
#14338=CARTESIAN_POINT('Ctrl Pts',(3.39480597714356,-2.40010391086475,4.69540747194623));
#14339=CARTESIAN_POINT('Ctrl Pts',(3.39499357523214,-2.35913959871511,4.69319354909316));
#14340=CARTESIAN_POINT('Ctrl Pts',(3.42673278397032,-2.24936123585863,4.68727502988782));
#14341=CARTESIAN_POINT('Ctrl Pts',(3.60557055480924,-2.15719836203143,4.6776519143302));
#14342=CARTESIAN_POINT('Ctrl Pts',(3.8070124874506,-2.27299804520947,4.6665381252734));
#14343=CARTESIAN_POINT('Ctrl Pts',(3.81897354264718,-2.50504405790744,4.65542433621659));
#14344=CARTESIAN_POINT('Ctrl Pts',(3.63050563092984,-2.64094205312202,4.64431054715979));
#14345=CARTESIAN_POINT('Ctrl Pts',(3.4356920506335,-2.56474249848871,4.63430492573633));
#14346=CARTESIAN_POINT('Ctrl Pts',(3.39504387850492,-2.44777554718273,4.62800390066515));
#14347=CARTESIAN_POINT('Ctrl Pts',(3.39465252302706,-2.39982399270837,4.62540747194623));
#14348=CARTESIAN_POINT('Origin',(3.6,-2.4,5.35459252805377));
#14349=CARTESIAN_POINT('',(3.39427330737243,-2.40012021866021,4.76540747194624));
#14350=CARTESIAN_POINT('',(3.39474358824326,-2.39985490132356,4.75959252805377));
#14351=CARTESIAN_POINT('',(3.394525,-2.39999999999999,5.35459252805377));
#14352=CARTESIAN_POINT('Ctrl Pts',(3.39474358824326,-2.39985490132356,4.75959252805377));
#14353=CARTESIAN_POINT('Ctrl Pts',(3.39458577609892,-2.37565177668507,4.75828346914551));
#14354=CARTESIAN_POINT('Ctrl Pts',(3.40973684003147,-2.28314575562072,4.75326981388497));
#14355=CARTESIAN_POINT('Ctrl Pts',(3.546828337511,-2.16302646659663,4.74455156227216));
#14356=CARTESIAN_POINT('Ctrl Pts',(3.77025746015408,-2.22680624004484,4.73343777321537));
#14357=CARTESIAN_POINT('Ctrl Pts',(3.83784799866721,-2.44911222613084,4.72232398415856));
#14358=CARTESIAN_POINT('Ctrl Pts',(3.68773356662048,-2.62646523466876,4.71121019510175));
#14359=CARTESIAN_POINT('Ctrl Pts',(3.46153062411222,-2.59707961114918,4.7002997097335));
#14360=CARTESIAN_POINT('Ctrl Pts',(3.3944881838605,-2.46423743809455,4.6930938207175));
#14361=CARTESIAN_POINT('Ctrl Pts',(3.39421139045774,-2.39993212258527,4.68959252805377));
#14362=CARTESIAN_POINT('Ctrl Pts',(3.39427330737243,-2.40012021866021,4.76540747194624));
#14363=CARTESIAN_POINT('Ctrl Pts',(3.39469744970711,-2.3391019374956,4.76208779387343));
#14364=CARTESIAN_POINT('Ctrl Pts',(3.45579878082125,-2.20925256261312,4.75506351944836));
#14365=CARTESIAN_POINT('Ctrl Pts',(3.67655777933124,-2.16951665373617,4.74433464867103));
#14366=CARTESIAN_POINT('Ctrl Pts',(3.83516271561975,-2.33931916560024,4.73322085961422));
#14367=CARTESIAN_POINT('Ctrl Pts',(3.77852055137491,-2.56466353335787,4.72210707055742));
#14368=CARTESIAN_POINT('Ctrl Pts',(3.55847650189588,-2.63928950162157,4.71099328150062));
#14369=CARTESIAN_POINT('Ctrl Pts',(3.41270209403565,-2.52365597038275,4.70209341529688));
#14370=CARTESIAN_POINT('Ctrl Pts',(3.3946796640253,-2.4276859083356,4.69689814544542));
#14371=CARTESIAN_POINT('Ctrl Pts',(3.39480597714356,-2.40010391086475,4.69540747194623));
#14372=CARTESIAN_POINT('Origin',(3.6,-2.4,5.35459252805377));
#14373=CARTESIAN_POINT('',(3.39444175959654,-2.39982008597895,4.83540747194623));
#14374=CARTESIAN_POINT('',(3.39473575570154,-2.40014879661129,4.82959252805377));
#14375=CARTESIAN_POINT('',(3.394525,-2.39999999999999,5.35459252805377));
#14376=CARTESIAN_POINT('Ctrl Pts',(3.39473575570154,-2.40014879661129,4.82959252805377));
#14377=CARTESIAN_POINT('Ctrl Pts',(3.39503502367394,-2.35550570215801,4.82717771392578));
#14378=CARTESIAN_POINT('Ctrl Pts',(3.43129921618784,-2.24193240937533,4.82105830344552));
#14379=CARTESIAN_POINT('Ctrl Pts',(3.61869057055051,-2.15785470519124,4.81123429661299));
#14380=CARTESIAN_POINT('Ctrl Pts',(3.81357662274397,-2.28437687323548,4.80012050755619));
#14381=CARTESIAN_POINT('Ctrl Pts',(3.81297357001622,-2.51673020046272,4.78900671849938));
#14382=CARTESIAN_POINT('Ctrl Pts',(3.61743339336808,-2.64223905139592,4.77789292944258));
#14383=CARTESIAN_POINT('Ctrl Pts',(3.43084783163214,-2.55735665460818,4.76808819929404));
#14384=CARTESIAN_POINT('Ctrl Pts',(3.39503237960207,-2.44414587323265,4.76198806549777));
#14385=CARTESIAN_POINT('Ctrl Pts',(3.39474358824326,-2.39985490132356,4.75959252805377));
#14386=CARTESIAN_POINT('Ctrl Pts',(3.39444175959654,-2.39982008597895,4.83540747194623));
#14387=CARTESIAN_POINT('Ctrl Pts',(3.39432007222796,-2.3865422800919,4.83468663500598));
#14388=CARTESIAN_POINT('Ctrl Pts',(3.40154215697383,-2.30515767781734,4.83026120171345));
#14389=CARTESIAN_POINT('Ctrl Pts',(3.51011506636152,-2.17438004258061,4.82213117206865));
#14390=CARTESIAN_POINT('Ctrl Pts',(3.74080744720095,-2.20211890112026,4.81101738301186));
#14391=CARTESIAN_POINT('Ctrl Pts',(3.84261717475225,-2.41098057358878,4.79990359395505));
#14392=CARTESIAN_POINT('Ctrl Pts',(3.72235665078693,-2.60979160252334,4.78878980489825));
#14393=CARTESIAN_POINT('Ctrl Pts',(3.49010169673754,-2.61657799846968,4.77767601584144));
#14394=CARTESIAN_POINT('Ctrl Pts',(3.3977657533099,-2.4823139974067,4.76988190485744));
#14395=CARTESIAN_POINT('Ctrl Pts',(3.39422412786341,-2.40719531789781,4.7657923902257));
#14396=CARTESIAN_POINT('Ctrl Pts',(3.39427330737243,-2.40012021866021,4.76540747194624));
#14397=CARTESIAN_POINT('Origin',(3.6,-2.4,5.35459252805377));
#14398=CARTESIAN_POINT('',(3.39485784898994,-2.39999218980985,4.90540747194623));
#14399=CARTESIAN_POINT('',(3.39420666496973,-2.4000617379826,4.89959252805377));
#14400=CARTESIAN_POINT('',(3.394525,-2.39999999999999,5.35459252805377));
#14401=CARTESIAN_POINT('Ctrl Pts',(3.39420666496973,-2.4000617379826,4.89959252805377));
#14402=CARTESIAN_POINT('Ctrl Pts',(3.39446260190468,-2.33540634192885,4.89607195870605));
#14403=CARTESIAN_POINT('Ctrl Pts',(3.46215556821269,-2.20225412189412,4.88884679300607));
#14404=CARTESIAN_POINT('Ctrl Pts',(3.68890791813162,-2.17399322284688,4.87791703095382));
#14405=CARTESIAN_POINT('Ctrl Pts',(3.83809972557463,-2.3521230545377,4.86680324189701));
#14406=CARTESIAN_POINT('Ctrl Pts',(3.76935615396461,-2.57407519737118,4.85568945284021));
#14407=CARTESIAN_POINT('Ctrl Pts',(3.54559897400137,-2.63669433790405,4.8445756637834));
#14408=CARTESIAN_POINT('Ctrl Pts',(3.4094345739418,-2.51613221625325,4.83587668885459));
#14409=CARTESIAN_POINT('Ctrl Pts',(3.39457591295976,-2.42399322794668,4.83088231027805));
#14410=CARTESIAN_POINT('Ctrl Pts',(3.39473575570154,-2.40014879661129,4.82959252805377));
#14411=CARTESIAN_POINT('Ctrl Pts',(3.39485784898994,-2.39999218980985,4.90540747194623));
#14412=CARTESIAN_POINT('Ctrl Pts',(3.3948463830005,-2.36617331876133,4.90358087978625));
#14413=CARTESIAN_POINT('Ctrl Pts',(3.41876410056102,-2.26378009325356,4.898049691274));
#14414=CARTESIAN_POINT('Ctrl Pts',(3.5802619217345,-2.1579378700657,4.88881390640948));
#14415=CARTESIAN_POINT('Ctrl Pts',(3.7926651914697,-2.25213590538246,4.87770011735268));
#14416=CARTESIAN_POINT('Ctrl Pts',(3.8287198264784,-2.48167562339262,4.86658632829587));
#14417=CARTESIAN_POINT('Ctrl Pts',(3.65542461045338,-2.63645671704841,4.85547253923907));
#14418=CARTESIAN_POINT('Ctrl Pts',(3.44592887677019,-2.57880492333736,4.84507958712252));
#14419=CARTESIAN_POINT('Ctrl Pts',(3.39494545996352,-2.45478089066832,4.83839123135824));
#14420=CARTESIAN_POINT('Ctrl Pts',(3.39444175959654,-2.39982008597895,4.83540747194623));
#14421=CARTESIAN_POINT('Origin',(3.6,-2.4,5.35459252805377));
#14422=CARTESIAN_POINT('',(3.39447042869063,-2.40018396912367,4.97540747194623));
#14423=CARTESIAN_POINT('',(3.39455385196002,-2.39981229693528,4.96959252805377));
#14424=CARTESIAN_POINT('',(3.394525,-2.39999999999999,5.35459252805377));
#14425=CARTESIAN_POINT('Ctrl Pts',(3.39455385196002,-2.39981229693529,4.96959252805377));
#14426=CARTESIAN_POINT('Ctrl Pts',(3.39439994110979,-2.38281031884833,4.9686707998386));
#14427=CARTESIAN_POINT('Ctrl Pts',(3.40410690463755,-2.29764758883809,4.96404447527116));
#14428=CARTESIAN_POINT('Ctrl Pts',(3.52244569995759,-2.16985002334435,4.95571355435144));
#14429=CARTESIAN_POINT('Ctrl Pts',(3.75130082069111,-2.21002173048044,4.94459976529465));
#14430=CARTESIAN_POINT('Ctrl Pts',(3.84166858438312,-2.42408270226789,4.93348597623783));
#14431=CARTESIAN_POINT('Ctrl Pts',(3.71083435207858,-2.61610050352316,4.92237218718104));
#14432=CARTESIAN_POINT('Ctrl Pts',(3.47855218037073,-2.61031906317225,4.91125839812423));
#14433=CARTESIAN_POINT('Ctrl Pts',(3.3958002253152,-2.47484313295797,4.90366517841514));
#14434=CARTESIAN_POINT('Ctrl Pts',(3.39419328664854,-2.40344140123838,4.89977655505832));
#14435=CARTESIAN_POINT('Ctrl Pts',(3.39420666496973,-2.4000617379826,4.89959252805377));
#14436=CARTESIAN_POINT('Ctrl Pts',(3.39447042869063,-2.40018396912367,4.97540747194623));
#14437=CARTESIAN_POINT('Ctrl Pts',(3.39496908844141,-2.34615078794508,4.97247512456653));
#14438=CARTESIAN_POINT('Ctrl Pts',(3.44450059908404,-2.22304562253723,4.96583818083456));
#14439=CARTESIAN_POINT('Ctrl Pts',(3.65214584962031,-2.16279865748873,4.9554966407503));
#14440=CARTESIAN_POINT('Ctrl Pts',(3.82756721091734,-2.31516586178242,4.94438285169351));
#14441=CARTESIAN_POINT('Ctrl Pts',(3.79469372311971,-2.54518271468373,4.9332690626367));
#14442=CARTESIAN_POINT('Ctrl Pts',(3.58361486265069,-2.64231218244471,4.9221552735799));
#14443=CARTESIAN_POINT('Ctrl Pts',(3.41976019754822,-2.53813915804107,4.91286807668307));
#14444=CARTESIAN_POINT('Ctrl Pts',(3.39486963770596,-2.43476294104758,4.90728547613852));
#14445=CARTESIAN_POINT('Ctrl Pts',(3.39485784898994,-2.39999218980985,4.90540747194623));
#14446=CARTESIAN_POINT('Origin',(3.6,-2.4,5.35459252805377));
#14447=CARTESIAN_POINT('',(3.39425291505627,-2.39989343747799,5.04540747194623));
#14448=CARTESIAN_POINT('',(3.39484565493551,-2.40005255540929,5.03959252805377));
#14449=CARTESIAN_POINT('',(3.394525,-2.39999999999999,5.35459252805377));
#14450=CARTESIAN_POINT('Ctrl Pts',(3.39484565493551,-2.40005255540928,5.03959252805377));
#14451=CARTESIAN_POINT('Ctrl Pts',(3.39493157796431,-2.36251978536397,5.03756504461887));
#14452=CARTESIAN_POINT('Ctrl Pts',(3.42276239101834,-2.25628891765328,5.03183296483171));
#14453=CARTESIAN_POINT('Ctrl Pts',(3.59337897177386,-2.15722470850713,5.02239628869227));
#14454=CARTESIAN_POINT('Ctrl Pts',(3.8003783179889,-2.26276949623011,5.01128249963547));
#14455=CARTESIAN_POINT('Ctrl Pts',(3.82396911763155,-2.49392292422242,5.00016871057867));
#14456=CARTESIAN_POINT('Ctrl Pts',(3.64255844375993,-2.63910763258347,4.98905492152186));
#14457=CARTESIAN_POINT('Ctrl Pts',(3.44046962807591,-2.57154454308001,4.97886286068022));
#14458=CARTESIAN_POINT('Ctrl Pts',(3.39501853731303,-2.45114441665013,4.97237539619086));
#14459=CARTESIAN_POINT('Ctrl Pts',(3.39455385196002,-2.39981229693529,4.96959252805377));
#14460=CARTESIAN_POINT('Ctrl Pts',(3.39425291505627,-2.39989343747799,5.04540747194623));
#14461=CARTESIAN_POINT('Ctrl Pts',(3.39421423202935,-2.39376493107826,5.04507396569907));
#14462=CARTESIAN_POINT('Ctrl Pts',(3.39724233967252,-2.31959956972988,5.04103586309963));
#14463=CARTESIAN_POINT('Ctrl Pts',(3.48711398605093,-2.18496417501817,5.03329316414794));
#14464=CARTESIAN_POINT('Ctrl Pts',(3.71944061581356,-2.18853461914439,5.02217937509113));
#14465=CARTESIAN_POINT('Ctrl Pts',(3.84244191526684,-2.38566174871763,5.01106558603433));
#14466=CARTESIAN_POINT('Ctrl Pts',(3.74353337026135,-2.59591283022398,4.99995179697752));
#14467=CARTESIAN_POINT('Ctrl Pts',(3.51324710863985,-2.62684268245385,4.98883800792072));
#14468=CARTESIAN_POINT('Ctrl Pts',(3.40217618139952,-2.49676321865199,4.98065656624362));
#14469=CARTESIAN_POINT('Ctrl Pts',(3.3943391040451,-2.41441388913183,4.97617972091879));
#14470=CARTESIAN_POINT('Ctrl Pts',(3.39447042869063,-2.40018396912367,4.97540747194623));
#14471=CARTESIAN_POINT('Origin',(3.6,-2.4,5.35459252805377));
#14472=CARTESIAN_POINT('',(3.39479089893477,-2.39988380139174,5.11540747194623));
#14473=CARTESIAN_POINT('',(3.39436118987868,-2.40016037422423,5.10959252805377));
#14474=CARTESIAN_POINT('',(3.394525,-2.39999999999999,5.35459252805377));
#14475=CARTESIAN_POINT('Ctrl Pts',(3.39436118987868,-2.40016037422423,5.10959252805377));
#14476=CARTESIAN_POINT('Ctrl Pts',(3.39485595410064,-2.34250465429438,5.10645928939914));
#14477=CARTESIAN_POINT('Ctrl Pts',(3.45020483509149,-2.21584694899168,5.09962145439226));
#14478=CARTESIAN_POINT('Ctrl Pts',(3.66489494634582,-2.16596525152154,5.08907902303309));
#14479=CARTESIAN_POINT('Ctrl Pts',(3.83182128201397,-2.32759432498908,5.07796523397629));
#14480=CARTESIAN_POINT('Ctrl Pts',(3.78655899034249,-2.55549738341204,5.06685144491949));
#14481=CARTESIAN_POINT('Ctrl Pts',(3.57053712854092,-2.64107179875281,5.05573765586268));
#14482=CARTESIAN_POINT('Ctrl Pts',(3.4159720352905,-2.53063333972521,5.04665135024078));
#14483=CARTESIAN_POINT('Ctrl Pts',(3.39477458031215,-2.43109926700468,5.04126964097114));
#14484=CARTESIAN_POINT('Ctrl Pts',(3.39484565493551,-2.40005255540928,5.03959252805377));
#14485=CARTESIAN_POINT('Ctrl Pts',(3.39479089893477,-2.39988380139174,5.11540747194623));
#14486=CARTESIAN_POINT('Ctrl Pts',(3.39465312034679,-2.37325776527266,5.11396821047934));
#14487=CARTESIAN_POINT('Ctrl Pts',(3.41183995517004,-2.27826800227929,5.10882435266019));
#14488=CARTESIAN_POINT('Ctrl Pts',(3.55516853033383,-2.16130913937078,5.09997589848876));
#14489=CARTESIAN_POINT('Ctrl Pts',(3.77622352465696,-2.23288041708187,5.08886210943196));
#14490=CARTESIAN_POINT('Ctrl Pts',(3.83598040928192,-2.457419700552,5.07774832037515));
#14491=CARTESIAN_POINT('Ctrl Pts',(3.67974110927284,-2.62940130358481,5.06663453131835));
#14492=CARTESIAN_POINT('Ctrl Pts',(3.45739290427932,-2.59254974530072,5.05585424850871));
#14493=CARTESIAN_POINT('Ctrl Pts',(3.39464392413157,-2.46184054479285,5.04877856205133));
#14494=CARTESIAN_POINT('Ctrl Pts',(3.39425291505627,-2.39989343747799,5.04540747194623));
#14495=CARTESIAN_POINT('Origin',(3.6,-2.4,5.35459252805377));
#14496=CARTESIAN_POINT('',(3.39473290683218,-2.40022967700174,5.18540747194623));
#14497=CARTESIAN_POINT('',(3.39434265963601,-2.39985006386652,5.17959252805377));
#14498=CARTESIAN_POINT('',(3.394525,-2.39999999999999,5.35459252805377));
#14499=CARTESIAN_POINT('',(3.54698297828114,-2.59851743256717,5.2));
#14500=CARTESIAN_POINT('Ctrl Pts',(3.54698297828114,-2.59851743256717,5.2));
#14501=CARTESIAN_POINT('Ctrl Pts',(3.48097120902544,-2.58088801151799,5.19629540364773));
#14502=CARTESIAN_POINT('Ctrl Pts',(3.40750558819668,-2.51127201784738,5.19143122762981));
#14503=CARTESIAN_POINT('Ctrl Pts',(3.39457125535004,-2.42165321144002,5.18656705161189));
#14504=CARTESIAN_POINT('Ctrl Pts',(3.39473290683218,-2.40022967700174,5.18540747194623));
#14505=CARTESIAN_POINT('',(3.65313154707148,-2.59887322485902,5.2));
#14506=CARTESIAN_POINT('Origin',(3.6,-2.4,5.2));
#14507=CARTESIAN_POINT('Ctrl Pts',(3.65313161981587,-2.59887345085171,5.2));
#14508=CARTESIAN_POINT('Ctrl Pts',(3.58867174169549,-2.61600530781671,5.19636770818145));
#14509=CARTESIAN_POINT('Ctrl Pts',(3.45069167513782,-2.58406709125274,5.1895652175327));
#14510=CARTESIAN_POINT('Ctrl Pts',(3.3948280192206,-2.45815906572508,5.18276272688396));
#14511=CARTESIAN_POINT('Ctrl Pts',(3.39434265963601,-2.39985006386652,5.17959252805377));
#14512=CARTESIAN_POINT('Origin',(-3.6,-2.4,4.7));
#14513=CARTESIAN_POINT('',(-3.76675587540948,-2.40012144305632,4.38714803633902));
#14514=CARTESIAN_POINT('',(-3.76680083731002,-2.3999030629831,4.36785196366098));
#14515=CARTESIAN_POINT('',(-3.7666,-2.4,4.7));
#14516=CARTESIAN_POINT('',(-3.76351293272515,-2.4319230454628,4.3));
#14517=CARTESIAN_POINT('Ctrl Pts',(-3.76680083731002,-2.3999030629831,4.36785196366098));
#14518=CARTESIAN_POINT('Ctrl Pts',(-3.76684159509423,-2.39409443145766,
4.36746222055426));
#14519=CARTESIAN_POINT('Ctrl Pts',(-3.76656457427738,-2.38828969174785,
4.36707247744754));
#14520=CARTESIAN_POINT('Ctrl Pts',(-3.76595694000634,-2.38251974073322,
4.36668273434082));
#14521=CARTESIAN_POINT('Ctrl Pts',(-3.76018123887082,-2.32767505172373,
4.36297813798855));
#14522=CARTESIAN_POINT('Ctrl Pts',(-3.72453483587179,-2.27597349778246,
4.35927354163629));
#14523=CARTESIAN_POINT('Ctrl Pts',(-3.675321975809,-2.25108560394313,4.35556894528402));
#14524=CARTESIAN_POINT('Ctrl Pts',(-3.6261091157462,-2.22619771010379,4.35186434893175));
#14525=CARTESIAN_POINT('Ctrl Pts',(-3.56332979861965,-2.22812347636638,
4.34815975257948));
#14526=CARTESIAN_POINT('Ctrl Pts',(-3.51573443717815,-2.25596350777206,
4.34445515622722));
#14527=CARTESIAN_POINT('Ctrl Pts',(-3.46813907573665,-2.28380353917775,
4.34075055987495));
#14528=CARTESIAN_POINT('Ctrl Pts',(-3.43572766998022,-2.33755783572652,
4.33704596352268));
#14529=CARTESIAN_POINT('Ctrl Pts',(-3.43329506857802,-2.39266164758784,
4.33334136717041));
#14530=CARTESIAN_POINT('Ctrl Pts',(-3.43086246717583,-2.44776545944916,
4.32963677081814));
#14531=CARTESIAN_POINT('Ctrl Pts',(-3.45840867012789,-2.50421878662303,
4.32593217446588));
#14532=CARTESIAN_POINT('Ctrl Pts',(-3.5034058713341,-2.53611223252088,4.32222757811361));
#14533=CARTESIAN_POINT('Ctrl Pts',(-3.5484030725403,-2.56800567841873,4.31852298176134));
#14534=CARTESIAN_POINT('Ctrl Pts',(-3.61085127200066,-2.57533924304056,
4.31481838540907));
#14535=CARTESIAN_POINT('Ctrl Pts',(-3.66197494402253,-2.55491156986817,
4.3111137890568));
#14536=CARTESIAN_POINT('Ctrl Pts',(-3.7130986160444,-2.53448389669578,4.30740919270454));
#14537=CARTESIAN_POINT('Ctrl Pts',(-3.75289776062778,-2.48629498572916,
4.30370459635227));
#14538=CARTESIAN_POINT('Ctrl Pts',(-3.76351293272515,-2.4319230454628,4.3));
#14539=CARTESIAN_POINT('',(-3.60525667617797,-2.23318013248672,4.3));
#14540=CARTESIAN_POINT('Origin',(-3.6,-2.4,4.3));
#14541=CARTESIAN_POINT('',(-3.766345497777,-2.40006497186855,4.31714803633902));
#14542=CARTESIAN_POINT('Ctrl Pts',(-3.60525667255608,-2.23317994016621,
4.3));
#14543=CARTESIAN_POINT('Ctrl Pts',(-3.65930633468078,-2.23495318766097,
4.30363229181855));
#14544=CARTESIAN_POINT('Ctrl Pts',(-3.71251718041942,-2.26542183293127,
4.30726458363711));
#14545=CARTESIAN_POINT('Ctrl Pts',(-3.74128612006692,-2.31121589839408,
4.31089687545566));
#14546=CARTESIAN_POINT('Ctrl Pts',(-3.75778986656855,-2.33748637123519,
4.31298059575011));
#14547=CARTESIAN_POINT('Ctrl Pts',(-3.76624997632687,-2.36880031787527,
4.31506431604457));
#14548=CARTESIAN_POINT('Ctrl Pts',(-3.766345497777,-2.40006497186855,4.31714803633902));
#14549=CARTESIAN_POINT('',(-3.7666,-2.4,4.2));
#14550=CARTESIAN_POINT('',(-3.7666,-2.4,4.7));
#14551=CARTESIAN_POINT('Origin',(-3.6,-2.4,4.2));
#14552=CARTESIAN_POINT('Ctrl Pts',(-3.766345497777,-2.40006497186855,4.31714803633902));
#14553=CARTESIAN_POINT('Ctrl Pts',(-3.76641980162283,-2.42438499660917,
4.31876891239684));
#14554=CARTESIAN_POINT('Ctrl Pts',(-3.76143276745508,-2.44867519480749,
4.32038978845465));
#14555=CARTESIAN_POINT('Ctrl Pts',(-3.75123332790854,-2.47053847327949,
4.32201066451247));
#14556=CARTESIAN_POINT('Ctrl Pts',(-3.72792197948242,-2.52050813091336,
4.32571526086474));
#14557=CARTESIAN_POINT('Ctrl Pts',(-3.67738234157418,-2.55780017273342,
4.329419857217));
#14558=CARTESIAN_POINT('Ctrl Pts',(-3.6227496090289,-2.56532196535192,4.33312445356927));
#14559=CARTESIAN_POINT('Ctrl Pts',(-3.56811687648362,-2.57284375797042,
4.33682904992154));
#14560=CARTESIAN_POINT('Ctrl Pts',(-3.5093910493013,-2.55059530138736,4.34053364627381));
#14561=CARTESIAN_POINT('Ctrl Pts',(-3.47344562081921,-2.50877156715293,
4.34423824262608));
#14562=CARTESIAN_POINT('Ctrl Pts',(-3.43750019233712,-2.4669478329185,4.34794283897835));
#14563=CARTESIAN_POINT('Ctrl Pts',(-3.42433516255526,-2.40554882103269,
4.35164743533061));
#14564=CARTESIAN_POINT('Ctrl Pts',(-3.4399769373371,-2.35266772584057,4.35535203168288));
#14565=CARTESIAN_POINT('Ctrl Pts',(-3.45561871211893,-2.29978663064845,
4.35905662803515));
#14566=CARTESIAN_POINT('Ctrl Pts',(-3.50006729146445,-2.25542345215002,
4.36276122438742));
#14567=CARTESIAN_POINT('Ctrl Pts',(-3.55297985415763,-2.23988445249497,
4.36646582073969));
#14568=CARTESIAN_POINT('Ctrl Pts',(-3.60589241685081,-2.22434545283993,
4.37017041709195));
#14569=CARTESIAN_POINT('Ctrl Pts',(-3.66726896289165,-2.23763063202826,
4.37387501344422));
#14570=CARTESIAN_POINT('Ctrl Pts',(-3.70902050597011,-2.2736583534049,4.37757960979649));
#14571=CARTESIAN_POINT('Ctrl Pts',(-3.74496653400264,-2.3046764520682,4.38076908531067));
#14572=CARTESIAN_POINT('Ctrl Pts',(-3.76636579491573,-2.35255215149476,
4.38395856082485));
#14573=CARTESIAN_POINT('Ctrl Pts',(-3.76675587540948,-2.40012144305632,
4.38714803633902));
#14574=CARTESIAN_POINT('Origin',(-3.6,-2.4,4.7));
#14575=CARTESIAN_POINT('',(-3.76672469163696,-2.39986752250016,4.45714803633902));
#14576=CARTESIAN_POINT('',(-3.76637108132843,-2.3999167674636,4.43785196366098));
#14577=CARTESIAN_POINT('',(-3.7666,-2.4,4.7));
#14578=CARTESIAN_POINT('Ctrl Pts',(-3.76637108132843,-2.3999167674636,4.43785196366098));
#14579=CARTESIAN_POINT('Ctrl Pts',(-3.76647256500337,-2.37748041616576,
4.43635646533454));
#14580=CARTESIAN_POINT('Ctrl Pts',(-3.7622516281058,-2.3550806593951,4.43486096700809));
#14581=CARTESIAN_POINT('Ctrl Pts',(-3.7535269013147,-2.3345994559913,4.43336546868165));
#14582=CARTESIAN_POINT('Ctrl Pts',(-3.73191431207048,-2.28386413246858,
4.42966087232938));
#14583=CARTESIAN_POINT('Ctrl Pts',(-3.68266490417161,-2.24490171859149,
4.42595627597712));
#14584=CARTESIAN_POINT('Ctrl Pts',(-3.62831780053848,-2.23554372384707,
4.42225167962485));
#14585=CARTESIAN_POINT('Ctrl Pts',(-3.57397069690535,-2.22618572910265,
4.41854708327258));
#14586=CARTESIAN_POINT('Ctrl Pts',(-3.51452589753796,-2.2464321534909,4.41484248692031));
#14587=CARTESIAN_POINT('Ctrl Pts',(-3.47718894803579,-2.28701682605767,
4.41113789056804));
#14588=CARTESIAN_POINT('Ctrl Pts',(-3.43985199853362,-2.32760149862444,
4.40743329421577));
#14589=CARTESIAN_POINT('Ctrl Pts',(-3.42462289889666,-2.38852441936972,
4.40372869786351));
#14590=CARTESIAN_POINT('Ctrl Pts',(-3.4384707400222,-2.441904428893,4.40002410151124));
#14591=CARTESIAN_POINT('Ctrl Pts',(-3.45231858114774,-2.49528443841629,
4.39631950515897));
#14592=CARTESIAN_POINT('Ctrl Pts',(-3.49524336303579,-2.54112153671759,
4.3926149088067));
#14593=CARTESIAN_POINT('Ctrl Pts',(-3.54760150310682,-2.55843699301478,
4.38891031245443));
#14594=CARTESIAN_POINT('Ctrl Pts',(-3.59995964317784,-2.57575244931197,
4.38520571610217));
#14595=CARTESIAN_POINT('Ctrl Pts',(-3.66175114143183,-2.56454626360505,
4.3815011197499));
#14596=CARTESIAN_POINT('Ctrl Pts',(-3.70469439092283,-2.52994925871274,
4.37779652339763));
#14597=CARTESIAN_POINT('Ctrl Pts',(-3.74311978370889,-2.49899204150246,
4.37448167015208));
#14598=CARTESIAN_POINT('Ctrl Pts',(-3.76645418313973,-2.44930678746824,
4.37116681690653));
#14599=CARTESIAN_POINT('Ctrl Pts',(-3.76680083731002,-2.3999030629831,4.36785196366098));
#14600=CARTESIAN_POINT('Ctrl Pts',(-3.76675587540948,-2.40012144305632,
4.38714803633902));
#14601=CARTESIAN_POINT('Ctrl Pts',(-3.76681887592163,-2.40780419002449,
4.38766315717712));
#14602=CARTESIAN_POINT('Ctrl Pts',(-3.76633386603033,-2.41547894454867,
4.38817827801521));
#14603=CARTESIAN_POINT('Ctrl Pts',(-3.76527362096253,-2.42307339831024,
4.3886933988533));
#14604=CARTESIAN_POINT('Ctrl Pts',(-3.75764865276043,-2.47769045827401,
4.39239799520556));
#14605=CARTESIAN_POINT('Ctrl Pts',(-3.72027217624014,-2.52815431463659,
4.39610259155783));
#14606=CARTESIAN_POINT('Ctrl Pts',(-3.67024983212249,-2.55136949856929,
4.3998071879101));
#14607=CARTESIAN_POINT('Ctrl Pts',(-3.62022748800484,-2.57458468250198,
4.40351178426236));
#14608=CARTESIAN_POINT('Ctrl Pts',(-3.55755927628983,-2.57055119400479,
4.40721638061464));
#14609=CARTESIAN_POINT('Ctrl Pts',(-3.51092561732084,-2.54111518112976,
4.4109209769669));
#14610=CARTESIAN_POINT('Ctrl Pts',(-3.46429195835185,-2.51167916825472,
4.41462557331917));
#14611=CARTESIAN_POINT('Ctrl Pts',(-3.43369285212889,-2.45684063100183,
4.41833016967144));
#14612=CARTESIAN_POINT('Ctrl Pts',(-3.433132174149,-2.40169663743424,4.4220347660237));
#14613=CARTESIAN_POINT('Ctrl Pts',(-3.4325714961691,-2.34655264386664,4.42573936237597));
#14614=CARTESIAN_POINT('Ctrl Pts',(-3.46204924643229,-2.29110319398435,
4.42944395872824));
#14615=CARTESIAN_POINT('Ctrl Pts',(-3.50807475488023,-2.26072509261964,
4.43314855508051));
#14616=CARTESIAN_POINT('Ctrl Pts',(-3.55410026332817,-2.23034699125494,
4.43685315143278));
#14617=CARTESIAN_POINT('Ctrl Pts',(-3.61667352996086,-2.22504023840783,
4.44055774778505));
#14618=CARTESIAN_POINT('Ctrl Pts',(-3.66715754973313,-2.24723347480277,
4.44426234413731));
#14619=CARTESIAN_POINT('Ctrl Pts',(-3.71764156950539,-2.26942671119771,
4.44796694048958));
#14620=CARTESIAN_POINT('Ctrl Pts',(-3.75603634241723,-2.3191199368347,4.45167153684185));
#14621=CARTESIAN_POINT('Ctrl Pts',(-3.76477028031358,-2.37357077761011,
4.45537613319412));
#14622=CARTESIAN_POINT('Ctrl Pts',(-3.76616275698799,-2.38225203073804,
4.45596676757575));
#14623=CARTESIAN_POINT('Ctrl Pts',(-3.76680128976178,-2.39105421690488,
4.45655740195739));
#14624=CARTESIAN_POINT('Ctrl Pts',(-3.76672469163696,-2.39986752250016,
4.45714803633902));
#14625=CARTESIAN_POINT('Origin',(-3.6,-2.4,4.7));
#14626=CARTESIAN_POINT('',(-3.76633791767176,-2.39996197521538,4.52714803633902));
#14627=CARTESIAN_POINT('',(-3.76649857915956,-2.40014312937522,4.50785196366098));
#14628=CARTESIAN_POINT('',(-3.7666,-2.4,4.7));
#14629=CARTESIAN_POINT('Ctrl Pts',(-3.76649857915956,-2.40014312937522,
4.50785196366098));
#14630=CARTESIAN_POINT('Ctrl Pts',(-3.76617946285532,-2.36119271347016,
4.50525071011481));
#14631=CARTESIAN_POINT('Ctrl Pts',(-3.75254367029535,-2.32204100961925,
4.50264945656865));
#14632=CARTESIAN_POINT('Ctrl Pts',(-3.7275842614224,-2.29243603978678,4.50004820302248));
#14633=CARTESIAN_POINT('Ctrl Pts',(-3.69203811667935,-2.25027388169498,
4.49634360667021));
#14634=CARTESIAN_POINT('Ctrl Pts',(-3.63352511503972,-2.22747466102272,
4.49263901031794));
#14635=CARTESIAN_POINT('Ctrl Pts',(-3.57882406120147,-2.23447257256027,
4.48893441396567));
#14636=CARTESIAN_POINT('Ctrl Pts',(-3.52412300736323,-2.24147048409781,
4.4852298176134));
#14637=CARTESIAN_POINT('Ctrl Pts',(-3.47323390132638,-2.27826552784516,
4.48152522126114));
#14638=CARTESIAN_POINT('Ctrl Pts',(-3.44944643562249,-2.32801823904553,
4.47782062490887));
#14639=CARTESIAN_POINT('Ctrl Pts',(-3.42565896991859,-2.37777095024589,
4.4741160285566));
#14640=CARTESIAN_POINT('Ctrl Pts',(-3.42897314454765,-2.44048132889927,
4.47041143220433));
#14641=CARTESIAN_POINT('Ctrl Pts',(-3.45787219950101,-2.4874496233209,4.46670683585206));
#14642=CARTESIAN_POINT('Ctrl Pts',(-3.48677125445436,-2.53441791774253,
4.46300223949979));
#14643=CARTESIAN_POINT('Ctrl Pts',(-3.54125518973201,-2.56564412793241,
4.45929764314753));
#14644=CARTESIAN_POINT('Ctrl Pts',(-3.59638914182557,-2.56683738431542,
4.45559304679526));
#14645=CARTESIAN_POINT('Ctrl Pts',(-3.65152309391912,-2.56803064069842,
4.45188845044299));
#14646=CARTESIAN_POINT('Ctrl Pts',(-3.7073070628286,-2.53919094327454,4.44818385409072));
#14647=CARTESIAN_POINT('Ctrl Pts',(-3.73821116198855,-2.49351697797843,
4.44447925773846));
#14648=CARTESIAN_POINT('Ctrl Pts',(-3.75663967023947,-2.4662810102851,4.44227015971263));
#14649=CARTESIAN_POINT('Ctrl Pts',(-3.76622117317942,-2.43305896393576,
4.4400610616868));
#14650=CARTESIAN_POINT('Ctrl Pts',(-3.76637108132843,-2.3999167674636,4.43785196366098));
#14651=CARTESIAN_POINT('Ctrl Pts',(-3.76672469163696,-2.39986752250016,
4.45714803633902));
#14652=CARTESIAN_POINT('Ctrl Pts',(-3.76632084848944,-2.44633332149978,
4.46026199830965));
#14653=CARTESIAN_POINT('Ctrl Pts',(-3.74603891301781,-2.49310820101244,
4.46337596028029));
#14654=CARTESIAN_POINT('Ctrl Pts',(-3.71156690339415,-2.52409905358083,
4.46648992225092));
#14655=CARTESIAN_POINT('Ctrl Pts',(-3.67055648569751,-2.56096803286229,
4.47019451860319));
#14656=CARTESIAN_POINT('Ctrl Pts',(-3.60946254742337,-2.57549753551134,
4.47389911495546));
#14657=CARTESIAN_POINT('Ctrl Pts',(-3.55624507519594,-2.56103805534263,
4.47760371130773));
#14658=CARTESIAN_POINT('Ctrl Pts',(-3.5030276029685,-2.54657857517392,4.48130830765999));
#14659=CARTESIAN_POINT('Ctrl Pts',(-3.45768659678778,-2.50313011218745,
4.48501290401226));
#14660=CARTESIAN_POINT('Ctrl Pts',(-3.44097262555956,-2.45057710029542,
4.48871750036453));
#14661=CARTESIAN_POINT('Ctrl Pts',(-3.42425865433133,-2.39802408840339,
4.4924220967168));
#14662=CARTESIAN_POINT('Ctrl Pts',(-3.43617171805559,-2.33636652760581,
4.49612669306907));
#14663=CARTESIAN_POINT('Ctrl Pts',(-3.47125973540437,-2.29382235099447,
4.49983128942134));
#14664=CARTESIAN_POINT('Ctrl Pts',(-3.50634775275315,-2.25127817438312,
4.5035358857736));
#14665=CARTESIAN_POINT('Ctrl Pts',(-3.56461072372645,-2.22784738195801,
4.50724048212587));
#14666=CARTESIAN_POINT('Ctrl Pts',(-3.61938426936618,-2.23425320834927,
4.51094507847814));
#14667=CARTESIAN_POINT('Ctrl Pts',(-3.67415781500591,-2.24065903474052,
4.51464967483041));
#14668=CARTESIAN_POINT('Ctrl Pts',(-3.72544193531206,-2.27690147994813,
4.51835427118268));
#14669=CARTESIAN_POINT('Ctrl Pts',(-3.74976616178516,-2.3263939836064,4.52205886753495));
#14670=CARTESIAN_POINT('Ctrl Pts',(-3.76090458576616,-2.34905733490504,
4.52375525713631));
#14671=CARTESIAN_POINT('Ctrl Pts',(-3.76638989772718,-2.37449903782319,
4.52545164673766));
#14672=CARTESIAN_POINT('Ctrl Pts',(-3.76633791767176,-2.39996197521538,
4.52714803633902));
#14673=CARTESIAN_POINT('Origin',(-3.6,-2.4,4.7));
#14674=CARTESIAN_POINT('',(-3.7665852438883,-2.4001523433009,4.59714803633902));
#14675=CARTESIAN_POINT('',(-3.76687644757351,-2.39999932887962,4.57785196366098));
#14676=CARTESIAN_POINT('',(-3.7666,-2.4,4.7));
#14677=CARTESIAN_POINT('Ctrl Pts',(-3.76687644620932,-2.39999932888293,
4.57785196366098));
#14678=CARTESIAN_POINT('Ctrl Pts',(-3.76687974213825,-2.34481655618538,
4.57414495489509));
#14679=CARTESIAN_POINT('Ctrl Pts',(-3.73679498392134,-2.28963687265016,
4.57043794612919));
#14680=CARTESIAN_POINT('Ctrl Pts',(-3.69041339984634,-2.25973893422683,
4.5667309373633));
#14681=CARTESIAN_POINT('Ctrl Pts',(-3.64406199955899,-2.22986045251336,
4.56302634101103));
#14682=CARTESIAN_POINT('Ctrl Pts',(-3.58143498915818,-2.22523082136041,
4.55932174465877));
#14683=CARTESIAN_POINT('Ctrl Pts',(-3.53119397503756,-2.24796881775056,
4.5556171483065));
#14684=CARTESIAN_POINT('Ctrl Pts',(-3.48095296091694,-2.27070681414072,
4.55191255195423));
#14685=CARTESIAN_POINT('Ctrl Pts',(-3.44309794307651,-2.32081243807398,
4.54820795560196));
#14686=CARTESIAN_POINT('Ctrl Pts',(-3.43495348515474,-2.3753545665717,4.54450335924969));
#14687=CARTESIAN_POINT('Ctrl Pts',(-3.42680902723298,-2.42989669506942,
4.54079876289742));
#14688=CARTESIAN_POINT('Ctrl Pts',(-3.44837512922987,-2.4888753281316,4.53709416654516));
#14689=CARTESIAN_POINT('Ctrl Pts',(-3.48978194213576,-2.52529856004066,
4.53338957019289));
#14690=CARTESIAN_POINT('Ctrl Pts',(-3.53118875504166,-2.56172179194972,
4.52968497384062));
#14691=CARTESIAN_POINT('Ctrl Pts',(-3.59243627885656,-2.57558962270566,
4.52598037748835));
#14692=CARTESIAN_POINT('Ctrl Pts',(-3.64549423729516,-2.5605553606569,4.52227578113609));
#14693=CARTESIAN_POINT('Ctrl Pts',(-3.69855219573377,-2.54552109860814,
4.51857118478382));
#14694=CARTESIAN_POINT('Ctrl Pts',(-3.74342058879608,-2.50158474375469,
4.51486658843155));
#14695=CARTESIAN_POINT('Ctrl Pts',(-3.759565141404,-2.4488540185723,4.51116199207928));
#14696=CARTESIAN_POINT('Ctrl Pts',(-3.76437348603424,-2.43314918577593,
4.51005864927318));
#14697=CARTESIAN_POINT('Ctrl Pts',(-3.76663393493028,-2.41666426444364,
4.50895530646708));
#14698=CARTESIAN_POINT('Ctrl Pts',(-3.76649857915956,-2.40014312937522,
4.50785196366098));
#14699=CARTESIAN_POINT('Ctrl Pts',(-3.76633791767176,-2.39996197521538,
4.52714803633902));
#14700=CARTESIAN_POINT('Ctrl Pts',(-3.76627638304661,-2.43010531182154,
4.52915624308993));
#14701=CARTESIAN_POINT('Ctrl Pts',(-3.75845482433377,-2.46027840666142,
4.53116444984084));
#14702=CARTESIAN_POINT('Ctrl Pts',(-3.74306538783811,-2.48590718051351,
4.53317265659175));
#14703=CARTESIAN_POINT('Ctrl Pts',(-3.71467605477792,-2.53318531165342,
4.53687725294402));
#14704=CARTESIAN_POINT('Ctrl Pts',(-3.66053305601751,-2.56499901182434,
4.54058184929628));
#14705=CARTESIAN_POINT('Ctrl Pts',(-3.60541524194112,-2.56678856079501,
4.54428644564855));
#14706=CARTESIAN_POINT('Ctrl Pts',(-3.55029742786473,-2.56857810976569,
4.54799104200082));
#14707=CARTESIAN_POINT('Ctrl Pts',(-3.49420479847236,-2.54034350753613,
4.55169563835309));
#14708=CARTESIAN_POINT('Ctrl Pts',(-3.46280846367734,-2.49500647989383,
4.55540023470536));
#14709=CARTESIAN_POINT('Ctrl Pts',(-3.43141212888233,-2.44966945225154,
4.55910483105763));
#14710=CARTESIAN_POINT('Ctrl Pts',(-3.42471208868465,-2.38722999919651,
4.56280942740989));
#14711=CARTESIAN_POINT('Ctrl Pts',(-3.44577465447007,-2.33626389048712,
4.56651402376216));
#14712=CARTESIAN_POINT('Ctrl Pts',(-3.46683722025548,-2.28529778177773,
4.57021862011443));
#14713=CARTESIAN_POINT('Ctrl Pts',(-3.515662392024,-2.24580501741397,4.5739232164667));
#14714=CARTESIAN_POINT('Ctrl Pts',(-3.56990505305945,-2.23585968494016,
4.57762781281897));
#14715=CARTESIAN_POINT('Ctrl Pts',(-3.62414771409491,-2.22591435246634,
4.58133240917123));
#14716=CARTESIAN_POINT('Ctrl Pts',(-3.68380786439731,-2.24551645188247,
4.5850370055235));
#14717=CARTESIAN_POINT('Ctrl Pts',(-3.72158169788407,-2.28569497124226,
4.58874160187577));
#14718=CARTESIAN_POINT('Ctrl Pts',(-3.75015370460556,-2.31608587465984,
4.59154374669686));
#14719=CARTESIAN_POINT('Ctrl Pts',(-3.76620375900909,-2.35824929108539,
4.59434589151794));
#14720=CARTESIAN_POINT('Ctrl Pts',(-3.7665852438883,-2.4001523433009,4.59714803633902));
#14721=CARTESIAN_POINT('Origin',(-3.6,-2.4,4.7));
#14722=CARTESIAN_POINT('',(-3.76685427080137,-2.39994496470643,4.66714803633902));
#14723=CARTESIAN_POINT('',(-3.76649662121988,-2.39985729252779,4.64785196366098));
#14724=CARTESIAN_POINT('',(-3.7666,-2.4,4.7));
#14725=CARTESIAN_POINT('Ctrl Pts',(-3.76649662121988,-2.39985729252779,
4.64785196366098));
#14726=CARTESIAN_POINT('Ctrl Pts',(-3.76663205173418,-2.38326341802857,
4.64674379602763));
#14727=CARTESIAN_POINT('Ctrl Pts',(-3.76435139460867,-2.36670593234144,
4.64563562839428));
#14728=CARTESIAN_POINT('Ctrl Pts',(-3.7595015341574,-2.35093871131677,4.64452746076093));
#14729=CARTESIAN_POINT('Ctrl Pts',(-3.74328848588199,-2.29822900591163,
4.64082286440866));
#14730=CARTESIAN_POINT('Ctrl Pts',(-3.69836304774957,-2.25435098262799,
4.63711826805639));
#14731=CARTESIAN_POINT('Ctrl Pts',(-3.64528560126629,-2.23938566762668,
4.63341367170413));
#14732=CARTESIAN_POINT('Ctrl Pts',(-3.59220815478301,-2.22442035262536,
4.62970907535186));
#14733=CARTESIAN_POINT('Ctrl Pts',(-3.53097869994887,-2.23836774590636,
4.62600447899959));
#14734=CARTESIAN_POINT('Ctrl Pts',(-3.48961924396277,-2.27484474384805,
4.62229988264732));
#14735=CARTESIAN_POINT('Ctrl Pts',(-3.44825978797668,-2.31132174178974,
4.61859528629506));
#14736=CARTESIAN_POINT('Ctrl Pts',(-3.42677033083864,-2.37032834439211,
4.61489068994278));
#14737=CARTESIAN_POINT('Ctrl Pts',(-3.43498564446249,-2.42485984538296,
4.61118609359052));
#14738=CARTESIAN_POINT('Ctrl Pts',(-3.44320095808634,-2.47939134637381,
4.60748149723825));
#14739=CARTESIAN_POINT('Ctrl Pts',(-3.48112104247208,-2.52944774575313,
4.60377690088598));
#14740=CARTESIAN_POINT('Ctrl Pts',(-3.53139155597687,-2.55212044850799,
4.60007230453371));
#14741=CARTESIAN_POINT('Ctrl Pts',(-3.58166206948165,-2.57479315126284,
4.59636770818145));
#14742=CARTESIAN_POINT('Ctrl Pts',(-3.64428301210547,-2.57008215739322,
4.59266311182917));
#14743=CARTESIAN_POINT('Ctrl Pts',(-3.69059555437608,-2.54014347995252,
4.58895851547691));
#14744=CARTESIAN_POINT('Ctrl Pts',(-3.73687793816318,-2.51022429842083,
4.58525633153826));
#14745=CARTESIAN_POINT('Ctrl Pts',(-3.76687315457017,-2.45511027888938,
4.58155414759962));
#14746=CARTESIAN_POINT('Ctrl Pts',(-3.76687644620932,-2.39999932888293,
4.57785196366098));
#14747=CARTESIAN_POINT('Ctrl Pts',(-3.7665852438883,-2.4001523433009,4.59714803633902));
#14748=CARTESIAN_POINT('Ctrl Pts',(-3.76670810392422,-2.41364753218216,
4.59805048787021));
#14749=CARTESIAN_POINT('Ctrl Pts',(-3.76520580454733,-2.42711571583196,
4.59895293940139));
#14750=CARTESIAN_POINT('Ctrl Pts',(-3.76197323580484,-2.44015494667501,
4.59985539093257));
#14751=CARTESIAN_POINT('Ctrl Pts',(-3.74870342356775,-2.49368146344449,
4.60355998728484));
#14752=CARTESIAN_POINT('Ctrl Pts',(-3.70627628242244,-2.53997955767999,
4.60726458363711));
#14753=CARTESIAN_POINT('Ctrl Pts',(-3.65410883409218,-2.55786064402731,
4.61096917998938));
#14754=CARTESIAN_POINT('Ctrl Pts',(-3.60194138576191,-2.57574173037463,
4.61467377634165));
#14755=CARTESIAN_POINT('Ctrl Pts',(-3.54003363024668,-2.56520580883379,
4.61837837269391));
#14756=CARTESIAN_POINT('Ctrl Pts',(-3.49671800289895,-2.53107470364031,
4.62208296904618));
#14757=CARTESIAN_POINT('Ctrl Pts',(-3.45340237555123,-2.49694359844684,
4.62578756539845));
#14758=CARTESIAN_POINT('Ctrl Pts',(-3.42867887637101,-2.43921730960073,
4.62949216175072));
#14759=CARTESIAN_POINT('Ctrl Pts',(-3.43386235494986,-2.38431460052291,
4.63319675810299));
#14760=CARTESIAN_POINT('Ctrl Pts',(-3.43904583352872,-2.3294118914451,4.63690135445526));
#14761=CARTESIAN_POINT('Ctrl Pts',(-3.47413628986665,-2.27733276213558,
4.64060595080752));
#14762=CARTESIAN_POINT('Ctrl Pts',(-3.52307437764419,-2.25191152143151,
4.64431054715979));
#14763=CARTESIAN_POINT('Ctrl Pts',(-3.57201246542174,-2.22649028072744,
4.64801514351206));
#14764=CARTESIAN_POINT('Ctrl Pts',(-3.6347981846389,-2.22772692862883,4.65171973986433));
#14765=CARTESIAN_POINT('Ctrl Pts',(-3.68269729487669,-2.25505550621137,
4.65542433621659));
#14766=CARTESIAN_POINT('Ctrl Pts',(-3.73059640511449,-2.28238408379392,
4.65912893256886));
#14767=CARTESIAN_POINT('Ctrl Pts',(-3.76360890637291,-2.33580459105762,
4.66283352892113));
#14768=CARTESIAN_POINT('Ctrl Pts',(-3.76662644025744,-2.39086882993835,
4.6665381252734));
#14769=CARTESIAN_POINT('Ctrl Pts',(-3.76679203880333,-2.3938906876002,4.66674142896194));
#14770=CARTESIAN_POINT('Ctrl Pts',(-3.76686730212629,-2.39691749565456,
4.66694473265048));
#14771=CARTESIAN_POINT('Ctrl Pts',(-3.76685427080137,-2.39994496470643,
4.66714803633902));
#14772=CARTESIAN_POINT('Origin',(-3.6,-2.4,4.7));
#14773=CARTESIAN_POINT('',(-3.7664227625968,-2.39988235338239,4.73714803633902));
#14774=CARTESIAN_POINT('',(-3.76637219995946,-2.40008425137793,4.71785196366098));
#14775=CARTESIAN_POINT('',(-3.7666,-2.4,4.7));
#14776=CARTESIAN_POINT('Ctrl Pts',(-3.76637219995946,-2.40008425137793,
4.71785196366098));
#14777=CARTESIAN_POINT('Ctrl Pts',(-3.76622009461901,-2.36687021016323,
4.7156380408079));
#14778=CARTESIAN_POINT('Ctrl Pts',(-3.7565937463241,-2.33357496437374,4.71342411795483));
#14779=CARTESIAN_POINT('Ctrl Pts',(-3.73808953535598,-2.30630352370031,
4.71121019510175));
#14780=CARTESIAN_POINT('Ctrl Pts',(-3.70712611115225,-2.26066973862981,
4.70750559874949));
#14781=CARTESIAN_POINT('Ctrl Pts',(-3.65130474062691,-2.23190256095558,
4.70380100239722));
#14782=CARTESIAN_POINT('Ctrl Pts',(-3.5961723905296,-2.23316745266121,4.70009640604495));
#14783=CARTESIAN_POINT('Ctrl Pts',(-3.54104004043228,-2.23443234436684,
4.69639180969269));
#14784=CARTESIAN_POINT('Ctrl Pts',(-3.48659671076299,-2.26572930545233,
4.69268721334042));
#14785=CARTESIAN_POINT('Ctrl Pts',(-3.45775870005953,-2.31273510421107,
4.68898261698815));
#14786=CARTESIAN_POINT('Ctrl Pts',(-3.42892068935607,-2.35974090296982,
4.68527802063588));
#14787=CARTESIAN_POINT('Ctrl Pts',(-3.42568799761845,-2.42245553940182,
4.68157342428361));
#14788=CARTESIAN_POINT('Ctrl Pts',(-3.44954008455102,-2.47217730452778,
4.67786882793134));
#14789=CARTESIAN_POINT('Ctrl Pts',(-3.47339217148359,-2.52189906965374,
4.67416423157907));
#14790=CARTESIAN_POINT('Ctrl Pts',(-3.52432903708635,-2.55862796347366,
4.6704596352268));
#14791=CARTESIAN_POINT('Ctrl Pts',(-3.57903913598448,-2.56555479946389,
4.66675503887454));
#14792=CARTESIAN_POINT('Ctrl Pts',(-3.63374923488261,-2.57248163545412,
4.66305044252227));
#14793=CARTESIAN_POINT('Ctrl Pts',(-3.69223256707613,-2.54960641361466,
4.65934584617));
#14794=CARTESIAN_POINT('Ctrl Pts',(-3.72772390396368,-2.50739810893161,
4.65564124981774));
#14795=CARTESIAN_POINT('Ctrl Pts',(-3.75259860490409,-2.47781570803419,
4.65304482109882));
#14796=CARTESIAN_POINT('Ctrl Pts',(-3.76617930850818,-2.43873661999706,
4.6504483923799));
#14797=CARTESIAN_POINT('Ctrl Pts',(-3.76649662121988,-2.39985729252779,
4.64785196366098));
#14798=CARTESIAN_POINT('Ctrl Pts',(-3.76685427080137,-2.39994496470643,
4.66714803633902));
#14799=CARTESIAN_POINT('Ctrl Pts',(-3.76662984554536,-2.45208398518876,
4.67064932900275));
#14800=CARTESIAN_POINT('Ctrl Pts',(-3.74021751929721,-2.50441905534817,
4.67415062166648));
#14801=CARTESIAN_POINT('Ctrl Pts',(-3.6980405151982,-2.53504001717725,4.6776519143302));
#14802=CARTESIAN_POINT('Ctrl Pts',(-3.65341448974379,-2.56743899503768,
4.68135651068247));
#14803=CARTESIAN_POINT('Ctrl Pts',(-3.59113987232435,-2.57552898026078,
4.68506110703474));
#14804=CARTESIAN_POINT('Ctrl Pts',(-3.53971699472298,-2.55560754523587,
4.68876570338701));
#14805=CARTESIAN_POINT('Ctrl Pts',(-3.48829411712161,-2.53568611021095,
4.69247029973928));
#14806=CARTESIAN_POINT('Ctrl Pts',(-3.4477229793383,-2.48775325493802,4.69617489609154));
#14807=CARTESIAN_POINT('Ctrl Pts',(-3.4365711926336,-2.4337457224305,4.69987949244381));
#14808=CARTESIAN_POINT('Ctrl Pts',(-3.42541940592889,-2.37973818992299,
4.70358408879608));
#14809=CARTESIAN_POINT('Ctrl Pts',(-3.44368697030278,-2.31965598018089,
4.70728868514835));
#14810=CARTESIAN_POINT('Ctrl Pts',(-3.48301363133541,-2.28099605718198,
4.71099328150062));
#14811=CARTESIAN_POINT('Ctrl Pts',(-3.52234029236805,-2.24233613418307,
4.71469787785288));
#14812=CARTESIAN_POINT('Ctrl Pts',(-3.58272605005944,-2.22509849792735,
4.71840247420515));
#14813=CARTESIAN_POINT('Ctrl Pts',(-3.63653501999159,-2.23717205039129,
4.72210707055742));
#14814=CARTESIAN_POINT('Ctrl Pts',(-3.69034398992373,-2.24924560285524,
4.72581166690969));
#14815=CARTESIAN_POINT('Ctrl Pts',(-3.73757617209662,-2.29063034403885,
4.72951626326196));
#14816=CARTESIAN_POINT('Ctrl Pts',(-3.75661549051415,-2.342386312472,4.73322085961422));
#14817=CARTESIAN_POINT('Ctrl Pts',(-3.76334323815838,-2.36067483977454,
4.73452991852249));
#14818=CARTESIAN_POINT('Ctrl Pts',(-3.76655071734768,-2.38025835805218,
4.73583897743076));
#14819=CARTESIAN_POINT('Ctrl Pts',(-3.7664227625968,-2.39988235338239,4.73714803633902));
#14820=CARTESIAN_POINT('Origin',(-3.6,-2.4,4.7));
#14821=CARTESIAN_POINT('',(-3.76642911325459,-2.40012064491874,4.80714803633902));
#14822=CARTESIAN_POINT('',(-3.76680409091049,-2.40009747380892,4.78785196366098));
#14823=CARTESIAN_POINT('',(-3.7666,-2.4,4.7));
#14824=CARTESIAN_POINT('Ctrl Pts',(-3.76680409091049,-2.40009747380892,
4.78785196366098));
#14825=CARTESIAN_POINT('Ctrl Pts',(-3.76646019447366,-2.35062358790434,
4.78453228558818));
#14826=CARTESIAN_POINT('Ctrl Pts',(-3.74304697023447,-2.30086701998663,
4.78121260751538));
#14827=CARTESIAN_POINT('Ctrl Pts',(-3.70452480595454,-2.26991420375009,
4.77789292944258));
#14828=CARTESIAN_POINT('Ctrl Pts',(-3.66153597807928,-2.23537239348787,
4.77418833309031));
#14829=CARTESIAN_POINT('Ctrl Pts',(-3.59973129997326,-2.22424775044289,
4.77048373673805));
#14830=CARTESIAN_POINT('Ctrl Pts',(-3.54739603302806,-2.24163153058572,
4.76677914038578));
#14831=CARTESIAN_POINT('Ctrl Pts',(-3.49506076608285,-2.25901531072854,
4.76307454403351));
#14832=CARTESIAN_POINT('Ctrl Pts',(-3.45219491029846,-2.30490751405916,
4.75936994768124));
#14833=CARTESIAN_POINT('Ctrl Pts',(-3.43841626764055,-2.35830531349683,
4.75566535132897));
#14834=CARTESIAN_POINT('Ctrl Pts',(-3.42463762498264,-2.4117031129345,4.7519607549767));
#14835=CARTESIAN_POINT('Ctrl Pts',(-3.4399461954512,-2.47260650847922,4.74825615862444));
#14836=CARTESIAN_POINT('Ctrl Pts',(-3.47733592496581,-2.51314271581421,
4.74455156227217));
#14837=CARTESIAN_POINT('Ctrl Pts',(-3.51472565448041,-2.55367892314919,
4.7408469659199));
#14838=CARTESIAN_POINT('Ctrl Pts',(-3.57419654304106,-2.57384794227444,
4.73714236956763));
#14839=CARTESIAN_POINT('Ctrl Pts',(-3.62853140127509,-2.56441930722117,
4.73343777321536));
#14840=CARTESIAN_POINT('Ctrl Pts',(-3.68286625950912,-2.55499067216789,
4.7297331768631));
#14841=CARTESIAN_POINT('Ctrl Pts',(-3.73206508741654,-2.5159643829361,4.72602858051083));
#14842=CARTESIAN_POINT('Ctrl Pts',(-3.75361176242918,-2.46520104208683,
4.72232398415856));
#14843=CARTESIAN_POINT('Ctrl Pts',(-3.7622818183227,-2.4447746420856,4.72083331065936));
#14844=CARTESIAN_POINT('Ctrl Pts',(-3.76647461518129,-2.42244785405319,
4.71934263716017));
#14845=CARTESIAN_POINT('Ctrl Pts',(-3.76637219995946,-2.40008425137793,
4.71785196366098));
#14846=CARTESIAN_POINT('Ctrl Pts',(-3.7664227625968,-2.39988235338239,4.73714803633902));
#14847=CARTESIAN_POINT('Ctrl Pts',(-3.76618860934753,-2.43579365983134,
4.73954357378302));
#14848=CARTESIAN_POINT('Ctrl Pts',(-3.75478479773435,-2.47184051531438,
4.74193911122703));
#14849=CARTESIAN_POINT('Ctrl Pts',(-3.73334402642865,-2.50033503613074,
4.74433464867103));
#14850=CARTESIAN_POINT('Ctrl Pts',(-3.70018678926345,-2.54440059567364,
4.7480392450233));
#14851=CARTESIAN_POINT('Ctrl Pts',(-3.64302586027087,-2.57040451907673,
4.75174384137556));
#14852=CARTESIAN_POINT('Ctrl Pts',(-3.58802126272889,-2.56644596334232,
4.75544843772783));
#14853=CARTESIAN_POINT('Ctrl Pts',(-3.53301666518691,-2.56248740760791,
4.7591530340801));
#14854=CARTESIAN_POINT('Ctrl Pts',(-3.48016839909552,-2.52856637273599,
4.76285763043237));
#14855=CARTESIAN_POINT('Ctrl Pts',(-3.4536627731015,-2.48020701268106,4.76656222678464));
#14856=CARTESIAN_POINT('Ctrl Pts',(-3.42715714710748,-2.43184765262612,
4.77026682313691));
#14857=CARTESIAN_POINT('Ctrl Pts',(-3.42699416121083,-2.36904996738817,
4.77397141948918));
#14858=CARTESIAN_POINT('Ctrl Pts',(-3.45324840683133,-2.32055367370344,
4.77767601584144));
#14859=CARTESIAN_POINT('Ctrl Pts',(-3.47950265245184,-2.2720573800187,4.78138061219371));
#14860=CARTESIAN_POINT('Ctrl Pts',(-3.53217412958951,-2.23786247788719,
4.78508520854597));
#14861=CARTESIAN_POINT('Ctrl Pts',(-3.58715743806471,-2.23361845816768,
4.78878980489824));
#14862=CARTESIAN_POINT('Ctrl Pts',(-3.6421407465399,-2.22937443844816,4.79249440125051));
#14863=CARTESIAN_POINT('Ctrl Pts',(-3.69943588635261,-2.25508130114064,
4.79619899760278));
#14864=CARTESIAN_POINT('Ctrl Pts',(-3.73282141188201,-2.29897415476607,
4.79990359395505));
#14865=CARTESIAN_POINT('Ctrl Pts',(-3.75458352333835,-2.32758539144982,
4.80231840808304));
#14866=CARTESIAN_POINT('Ctrl Pts',(-3.76618646552292,-2.36392383602884,
4.80473322221103));
#14867=CARTESIAN_POINT('Ctrl Pts',(-3.76642911325459,-2.40012064491874,
4.80714803633902));
#14868=CARTESIAN_POINT('Origin',(-3.6,-2.4,4.7));
#14869=CARTESIAN_POINT('',(-3.76685810224694,-2.40005005741615,4.87714803633902));
#14870=CARTESIAN_POINT('',(-3.76666750911963,-2.3998541249347,4.85785196366098));
#14871=CARTESIAN_POINT('',(-3.7666,-2.4,4.7));
#14872=CARTESIAN_POINT('Ctrl Pts',(-3.76666750911963,-2.3998541249347,4.85785196366098));
#14873=CARTESIAN_POINT('Ctrl Pts',(-3.76676617376365,-2.38908842257499,
4.85713112672072));
#14874=CARTESIAN_POINT('Ctrl Pts',(-3.76581236816026,-2.37834012863908,
4.85641028978047));
#14875=CARTESIAN_POINT('Ctrl Pts',(-3.76374257749965,-2.36781121686714,
4.85568945284021));
#14876=CARTESIAN_POINT('Ctrl Pts',(-3.75310530504175,-2.31369999425172,
4.85198485648794));
#14877=CARTESIAN_POINT('Ctrl Pts',(-3.71299219872321,-2.26538317916478,
4.84828026013567));
#14878=CARTESIAN_POINT('Ctrl Pts',(-3.66176124910748,-2.24497323600586,
4.8445756637834));
#14879=CARTESIAN_POINT('Ctrl Pts',(-3.61053029949175,-2.22456329284695,
4.84087106743114));
#14880=CARTESIAN_POINT('Ctrl Pts',(-3.54818150657882,-2.23206022161606,
4.83716647107887));
#14881=CARTESIAN_POINT('Ctrl Pts',(-3.50324914898701,-2.26403301035152,
4.8334618747266));
#14882=CARTESIAN_POINT('Ctrl Pts',(-3.45831679139521,-2.29600579908698,
4.82975727837433));
#14883=CARTESIAN_POINT('Ctrl Pts',(-3.43080086912452,-2.35245444778878,
4.82605268202206));
#14884=CARTESIAN_POINT('Ctrl Pts',(-3.43329420002801,-2.40754491229296,
4.82234808566979));
#14885=CARTESIAN_POINT('Ctrl Pts',(-3.43578753093151,-2.46263537679713,
4.81864348931753));
#14886=CARTESIAN_POINT('Ctrl Pts',(-3.4682901150092,-2.51636765710367,4.81493889296526));
#14887=CARTESIAN_POINT('Ctrl Pts',(-3.51592696035573,-2.54415087044753,
4.81123429661299));
#14888=CARTESIAN_POINT('Ctrl Pts',(-3.56356380570226,-2.5719340837914,4.80752970026073));
#14889=CARTESIAN_POINT('Ctrl Pts',(-3.62633491231765,-2.57376823017258,
4.80382510390846));
#14890=CARTESIAN_POINT('Ctrl Pts',(-3.67551272732296,-2.54881390209942,
4.80012050755619));
#14891=CARTESIAN_POINT('Ctrl Pts',(-3.72469054232828,-2.52385957402626,
4.79641591120392));
#14892=CARTESIAN_POINT('Ctrl Pts',(-3.76027506572354,-2.47211677149876,
4.79271131485165));
#14893=CARTESIAN_POINT('Ctrl Pts',(-3.76598083859892,-2.41726588149528,
4.78900671849938));
#14894=CARTESIAN_POINT('Ctrl Pts',(-3.76657368490912,-2.41156671532445,
4.78862180021991));
#14895=CARTESIAN_POINT('Ctrl Pts',(-3.7668439658688,-2.40583399482793,4.78823688194045));
#14896=CARTESIAN_POINT('Ctrl Pts',(-3.76680409091049,-2.40009747380892,
4.78785196366098));
#14897=CARTESIAN_POINT('Ctrl Pts',(-3.76642911325459,-2.40012064491874,
4.80714803633902));
#14898=CARTESIAN_POINT('Ctrl Pts',(-3.76655871442242,-2.41945381020902,
4.8084378185633));
#14899=CARTESIAN_POINT('Ctrl Pts',(-3.76344749532011,-2.43874657022512,
4.80972760078758));
#14900=CARTESIAN_POINT('Ctrl Pts',(-3.75691244110645,-2.45679995321808,
4.81101738301185));
#14901=CARTESIAN_POINT('Ctrl Pts',(-3.73814203355539,-2.50865405348629,
4.81472197936412));
#14902=CARTESIAN_POINT('Ctrl Pts',(-3.69112530720718,-2.55028340946432,
4.81842657571639));
#14903=CARTESIAN_POINT('Ctrl Pts',(-3.63737973347804,-2.56263611033431,
4.82213117206866));
#14904=CARTESIAN_POINT('Ctrl Pts',(-3.58363415974891,-2.5749888112043,4.82583576842093));
#14905=CARTESIAN_POINT('Ctrl Pts',(-3.52315973863885,-2.55806485696625,
4.82954036477319));
#14906=CARTESIAN_POINT('Ctrl Pts',(-3.48363293188217,-2.51960959124259,
4.83324496112546));
#14907=CARTESIAN_POINT('Ctrl Pts',(-3.44410612512549,-2.48115432551893,
4.83694955747773));
#14908=CARTESIAN_POINT('Ctrl Pts',(-3.42552693272221,-2.42116774830966,
4.84065415383));
#14909=CARTESIAN_POINT('Ctrl Pts',(-3.43639822742686,-2.36710305682155,
4.84435875018227));
#14910=CARTESIAN_POINT('Ctrl Pts',(-3.44726952213151,-2.31303836533343,
4.84806334653454));
#14911=CARTESIAN_POINT('Ctrl Pts',(-3.48759130394411,-2.26489555956646,
4.8517679428868));
#14912=CARTESIAN_POINT('Ctrl Pts',(-3.53891008077804,-2.24470746756836,
4.85547253923907));
#14913=CARTESIAN_POINT('Ctrl Pts',(-3.59022885761198,-2.22451937557026,
4.85917713559134));
#14914=CARTESIAN_POINT('Ctrl Pts',(-3.65254462946725,-2.23228599734102,
4.86288173194361));
#14915=CARTESIAN_POINT('Ctrl Pts',(-3.69733822999987,-2.26445289438714,
4.86658632829587));
#14916=CARTESIAN_POINT('Ctrl Pts',(-3.73990669414912,-2.29502189057005,
4.87010689764359));
#14917=CARTESIAN_POINT('Ctrl Pts',(-3.76665058750282,-2.34762719015485,
4.87362746699131));
#14918=CARTESIAN_POINT('Ctrl Pts',(-3.76685810224694,-2.40005005741615,
4.87714803633902));
#14919=CARTESIAN_POINT('Origin',(-3.6,-2.4,4.7));
#14920=CARTESIAN_POINT('',(-3.76657660157387,-2.39984780956506,4.94714803633902));
#14921=CARTESIAN_POINT('',(-3.76633014204238,-2.3999936674641,4.92785196366098));
#14922=CARTESIAN_POINT('',(-3.7666,-2.4,4.7));
#14923=CARTESIAN_POINT('Ctrl Pts',(-3.76633014204238,-2.3999936674641,4.92785196366098));
#14924=CARTESIAN_POINT('Ctrl Pts',(-3.76633943871615,-2.37257318075516,
4.926025371501));
#14925=CARTESIAN_POINT('Ctrl Pts',(-3.75993532676097,-2.34515678209823,
4.92419877934102));
#14926=CARTESIAN_POINT('Ctrl Pts',(-3.74709395990921,-2.32118936363805,
4.92237218718104));
#14927=CARTESIAN_POINT('Ctrl Pts',(-3.72104978768541,-2.27257992966252,
4.91866759082877));
#14928=CARTESIAN_POINT('Ctrl Pts',(-3.66852675339565,-2.23815745462599,
4.9149629944765));
#14929=CARTESIAN_POINT('Ctrl Pts',(-3.61356232150655,-2.23367557941999,
4.91125839812423));
#14930=CARTESIAN_POINT('Ctrl Pts',(-3.55859788961746,-2.22919370421399,
4.90755380177196));
#14931=CARTESIAN_POINT('Ctrl Pts',(-3.50119206012902,-2.25465242883852,
4.90384920541969));
#14932=CARTESIAN_POINT('Ctrl Pts',(-3.4676169364208,-2.2984004236072,4.90014460906743));
#14933=CARTESIAN_POINT('Ctrl Pts',(-3.43404181271257,-2.34214841837589,
4.89644001271516));
#14934=CARTESIAN_POINT('Ctrl Pts',(-3.42429739478456,-2.40418568328873,
4.89273541636289));
#14935=CARTESIAN_POINT('Ctrl Pts',(-3.44284327075563,-2.45612051228373,
4.88903082001062));
#14936=CARTESIAN_POINT('Ctrl Pts',(-3.46138914672669,-2.50805534127872,
4.88532622365836));
#14937=CARTESIAN_POINT('Ctrl Pts',(-3.50822531659685,-2.54988773435588,
4.88162162730609));
#14938=CARTESIAN_POINT('Ctrl Pts',(-3.56191694164611,-2.56247285961735,
4.87791703095382));
#14939=CARTESIAN_POINT('Ctrl Pts',(-3.61560856669538,-2.57505798487881,
4.87421243460155));
#14940=CARTESIAN_POINT('Ctrl Pts',(-3.67615564692375,-2.55839584232458,
4.87050783824928));
#14941=CARTESIAN_POINT('Ctrl Pts',(-3.7158484677393,-2.52011195597552,4.86680324189701));
#14942=CARTESIAN_POINT('Ctrl Pts',(-3.74781789610229,-2.48927731291044,
4.863819482485));
#14943=CARTESIAN_POINT('Ctrl Pts',(-3.76625910668661,-2.44441658275108,
4.86083572307299));
#14944=CARTESIAN_POINT('Ctrl Pts',(-3.76666750911963,-2.3998541249347,4.85785196366098));
#14945=CARTESIAN_POINT('Ctrl Pts',(-3.76685810224694,-2.40005005741615,
4.87714803633902));
#14946=CARTESIAN_POINT('Ctrl Pts',(-3.76686894944607,-2.40279030260928,
4.87733206334357));
#14947=CARTESIAN_POINT('Ctrl Pts',(-3.76680728980785,-2.40553004933232,
4.87751609034813));
#14948=CARTESIAN_POINT('Ctrl Pts',(-3.76667159341225,-2.40826612418172,
4.87770011735268));
#14949=CARTESIAN_POINT('Ctrl Pts',(-3.76393992708203,-2.46334528460871,
4.88140471370495));
#14950=CARTESIAN_POINT('Ctrl Pts',(-3.73120516521163,-2.5169364331412,4.88510931005721));
#14951=CARTESIAN_POINT('Ctrl Pts',(-3.6834485571899,-2.54451327676931,4.88881390640948));
#14952=CARTESIAN_POINT('Ctrl Pts',(-3.63569194916816,-2.57209012039741,
4.89251850276175));
#14953=CARTESIAN_POINT('Ctrl Pts',(-3.57291349499508,-2.57365265912114,
4.89622309911402));
#14954=CARTESIAN_POINT('Ctrl Pts',(-3.52384411020076,-2.5484857882364,4.89992769546629));
#14955=CARTESIAN_POINT('Ctrl Pts',(-3.47477472540644,-2.52331891735167,
4.90363229181856));
#14956=CARTESIAN_POINT('Ctrl Pts',(-3.43941440999087,-2.47142263685848,
4.90733688817082));
#14957=CARTESIAN_POINT('Ctrl Pts',(-3.43394601281114,-2.41654757379038,
4.91104148452309));
#14958=CARTESIAN_POINT('Ctrl Pts',(-3.42847761563141,-2.36167251072229,
4.91474608087536));
#14959=CARTESIAN_POINT('Ctrl Pts',(-3.45290113668751,-2.30381866507929,
4.91845067722763));
#14960=CARTESIAN_POINT('Ctrl Pts',(-3.4960390130763,-2.2694631773857,4.9221552735799));
#14961=CARTESIAN_POINT('Ctrl Pts',(-3.53917688946509,-2.23510768969211,
4.92585986993217));
#14962=CARTESIAN_POINT('Ctrl Pts',(-3.60102912118658,-2.22425055994793,
4.92956446628443));
#14963=CARTESIAN_POINT('Ctrl Pts',(-3.65328868366947,-2.24186061512031,
4.9332690626367));
#14964=CARTESIAN_POINT('Ctrl Pts',(-3.70554824615237,-2.25947067029269,
4.93697365898897));
#14965=CARTESIAN_POINT('Ctrl Pts',(-3.74821513939667,-2.30554791038164,
4.94067825534123));
#14966=CARTESIAN_POINT('Ctrl Pts',(-3.76176261776726,-2.35900482523354,
4.9443828516935));
#14967=CARTESIAN_POINT('Ctrl Pts',(-3.76513332050279,-2.37230526124053,
4.94530457990868));
#14968=CARTESIAN_POINT('Ctrl Pts',(-3.76670139313906,-2.38606253416914,
4.94622630812385));
#14969=CARTESIAN_POINT('Ctrl Pts',(-3.76657660157387,-2.39984780956506,
4.94714803633902));
#14970=CARTESIAN_POINT('Origin',(-3.6,-2.4,4.7));
#14971=CARTESIAN_POINT('',(-3.76634000649331,-2.40004261214866,5.01714803633902));
#14972=CARTESIAN_POINT('',(-3.76664426409402,-2.40014916296054,4.99785196366098));
#14973=CARTESIAN_POINT('',(-3.7666,-2.4,4.7));
#14974=CARTESIAN_POINT('Ctrl Pts',(-3.76664426409402,-2.40014916296054,
4.99785196366098));
#14975=CARTESIAN_POINT('Ctrl Pts',(-3.76623994861442,-2.35633882629306,
4.99491961628127));
#14976=CARTESIAN_POINT('Ctrl Pts',(-3.74849621908403,-2.31223872253049,
4.99198726890157));
#14977=CARTESIAN_POINT('Ctrl Pts',(-3.71750016680111,-2.28150333241251,
4.98905492152186));
#14978=CARTESIAN_POINT('Ctrl Pts',(-3.678341142527,-2.24267361704367,4.98535032516959));
#14979=CARTESIAN_POINT('Ctrl Pts',(-3.61803053121903,-2.22517487203488,
4.98164572881732));
#14980=CARTESIAN_POINT('Ctrl Pts',(-3.56416982600182,-2.23701549741557,
4.97794113246506));
#14981=CARTESIAN_POINT('Ctrl Pts',(-3.51030912078461,-2.24885612279626,
4.97423653611279));
#14982=CARTESIAN_POINT('Ctrl Pts',(-3.46289832165815,-2.29003611856643,
4.97053193976052));
#14983=CARTESIAN_POINT('Ctrl Pts',(-3.44363524974256,-2.34170922607974,
4.96682734340825));
#14984=CARTESIAN_POINT('Ctrl Pts',(-3.42437217782697,-2.39338233359304,
4.96312274705598));
#14985=CARTESIAN_POINT('Ctrl Pts',(-3.43325683312225,-2.45554855284948,
4.95941815070371));
#14986=CARTESIAN_POINT('Ctrl Pts',(-3.46622310272193,-2.4997571611377,4.95571355435145));
#14987=CARTESIAN_POINT('Ctrl Pts',(-3.49918937232162,-2.54396576942592,
4.95200895799918));
#14988=CARTESIAN_POINT('Ctrl Pts',(-3.55623725622572,-2.57021676674591,
4.94830436164691));
#14989=CARTESIAN_POINT('Ctrl Pts',(-3.61125846689758,-2.56649623530203,
4.94459976529464));
#14990=CARTESIAN_POINT('Ctrl Pts',(-3.66627967756944,-2.56277570385816,
4.94089516894238));
#14991=CARTESIAN_POINT('Ctrl Pts',(-3.71927421500904,-2.52908364365041,
4.93719057259011));
#14992=CARTESIAN_POINT('Ctrl Pts',(-3.74598882864993,-2.48083941708926,
4.93348597623784));
#14993=CARTESIAN_POINT('Ctrl Pts',(-3.7595315068913,-2.45638253943781,4.93160797204555));
#14994=CARTESIAN_POINT('Ctrl Pts',(-3.76632058370052,-2.4281859427416,4.92972996785327));
#14995=CARTESIAN_POINT('Ctrl Pts',(-3.76633014204238,-2.3999936674641,4.92785196366098));
#14996=CARTESIAN_POINT('Ctrl Pts',(-3.76657660157387,-2.39984780956506,
4.94714803633902));
#14997=CARTESIAN_POINT('Ctrl Pts',(-3.76619983273375,-2.44146810829183,
4.94993090447612));
#14998=CARTESIAN_POINT('Ctrl Pts',(-3.75039179589374,-2.48334366291991,
4.95271377261321));
#14999=CARTESIAN_POINT('Ctrl Pts',(-3.7221733933057,-2.5136723837762,4.95549664075031));
#15000=CARTESIAN_POINT('Ctrl Pts',(-3.68460862697666,-2.55404643785209,
4.95920123710258));
#15001=CARTESIAN_POINT('Ctrl Pts',(-3.62505103082171,-2.57395795638902,
4.96290583345484));
#15002=CARTESIAN_POINT('Ctrl Pts',(-3.57075747641916,-2.56429432021831,
4.96661042980711));
#15003=CARTESIAN_POINT('Ctrl Pts',(-3.51646392201662,-2.5546306840476,4.97031502615938));
#15004=CARTESIAN_POINT('Ctrl Pts',(-3.46743440936648,-2.51539189316926,
4.97401962251165));
#15005=CARTESIAN_POINT('Ctrl Pts',(-3.44610757298242,-2.46453580233588,
4.97772421886392));
#15006=CARTESIAN_POINT('Ctrl Pts',(-3.42478073659837,-2.41367971150249,
4.98142881521618));
#15007=CARTESIAN_POINT('Ctrl Pts',(-3.43115657648041,-2.35120632071406,
4.98513341156845));
#15008=CARTESIAN_POINT('Ctrl Pts',(-3.46231715328677,-2.30570693229799,
4.98883800792072));
#15009=CARTESIAN_POINT('Ctrl Pts',(-3.49347773009313,-2.26020754388192,
4.99254260427299));
#15010=CARTESIAN_POINT('Ctrl Pts',(-3.54942304382382,-2.2316821578382,4.99624720062526));
#15011=CARTESIAN_POINT('Ctrl Pts',(-3.60454940455119,-2.2331855772681,4.99995179697753));
#15012=CARTESIAN_POINT('Ctrl Pts',(-3.65967576527857,-2.23468899669801,
5.00365639332979));
#15013=CARTESIAN_POINT('Ctrl Pts',(-3.71398317300263,-2.26622122160152,
5.00736098968206));
#15014=CARTESIAN_POINT('Ctrl Pts',(-3.74261753436876,-2.31335135359861,
5.01106558603433));
#15015=CARTESIAN_POINT('Ctrl Pts',(-3.75828879455967,-2.33914513862194,
5.01309306946923));
#15016=CARTESIAN_POINT('Ctrl Pts',(-3.76627033973982,-2.36961088421597,
5.01512055290412));
#15017=CARTESIAN_POINT('Ctrl Pts',(-3.76634000649331,-2.40004261214866,
5.01714803633902));
#15018=CARTESIAN_POINT('Origin',(-3.6,-2.4,4.7));
#15019=CARTESIAN_POINT('',(-3.76673281282141,-2.40013003219325,5.08714803633902));
#15020=CARTESIAN_POINT('',(-3.7668206250807,-2.39991359866148,5.06785196366098));
#15021=CARTESIAN_POINT('',(-3.7666,-2.4,4.7));
#15022=CARTESIAN_POINT('Ctrl Pts',(-3.7668206250807,-2.39991359866148,5.06785196366098));
#15023=CARTESIAN_POINT('Ctrl Pts',(-3.76685198944486,-2.39494457920613,
5.06751845741382));
#15024=CARTESIAN_POINT('Ctrl Pts',(-3.7666492146414,-2.38997815520014,5.06718495116665));
#15025=CARTESIAN_POINT('Ctrl Pts',(-3.7662039619217,-2.38503356610626,5.06685144491949));
#15026=CARTESIAN_POINT('Ctrl Pts',(-3.76125808275068,-2.33010893762799,
5.06314684856722));
#15027=CARTESIAN_POINT('Ctrl Pts',(-3.72639327521678,-2.27787848097877,
5.05944225221495));
#15028=CARTESIAN_POINT('Ctrl Pts',(-3.67756563230702,-2.25224574125102,
5.05573765586268));
#15029=CARTESIAN_POINT('Ctrl Pts',(-3.62873798939725,-2.22661300152326,
5.05203305951042));
#15030=CARTESIAN_POINT('Ctrl Pts',(-3.56594751111163,-2.22757797871697,
5.04832846315815));
#15031=CARTESIAN_POINT('Ctrl Pts',(-3.51793060783244,-2.25469905531577,
5.04462386680588));
#15032=CARTESIAN_POINT('Ctrl Pts',(-3.46991370455325,-2.28182013191457,
5.04091927045361));
#15033=CARTESIAN_POINT('Ctrl Pts',(-3.43667037628051,-2.33509730791846,
5.03721467410135));
#15034=CARTESIAN_POINT('Ctrl Pts',(-3.43341462472151,-2.39014797674899,
5.03351007774908));
#15035=CARTESIAN_POINT('Ctrl Pts',(-3.43015887316251,-2.44519864557951,
5.02980548139681));
#15036=CARTESIAN_POINT('Ctrl Pts',(-3.45689069831725,-2.50202280723666,
5.02610088504454));
#15037=CARTESIAN_POINT('Ctrl Pts',(-3.50137612681596,-2.53461456435925,
5.02239628869227));
#15038=CARTESIAN_POINT('Ctrl Pts',(-3.54586155531466,-2.56720632148184,
5.01869169234));
#15039=CARTESIAN_POINT('Ctrl Pts',(-3.60810058715733,-2.57556567406988,
5.01498709598774));
#15040=CARTESIAN_POINT('Ctrl Pts',(-3.65960917750461,-2.5558669157941,5.01128249963547));
#15041=CARTESIAN_POINT('Ctrl Pts',(-3.71111776785188,-2.53616815751832,
5.0075779032832));
#15042=CARTESIAN_POINT('Ctrl Pts',(-3.75189591670377,-2.48841128837874,
5.00387330693093));
#15043=CARTESIAN_POINT('Ctrl Pts',(-3.7632812725096,-2.4344525109445,5.00016871057867));
#15044=CARTESIAN_POINT('Ctrl Pts',(-3.76565462941201,-2.42320442708544,
4.9993964616061));
#15045=CARTESIAN_POINT('Ctrl Pts',(-3.7667507426838,-2.41168684356181,4.99862421263354));
#15046=CARTESIAN_POINT('Ctrl Pts',(-3.76664426409402,-2.40014916296054,
4.99785196366098));
#15047=CARTESIAN_POINT('Ctrl Pts',(-3.76634000649331,-2.40004261214866,
5.01714803633902));
#15048=CARTESIAN_POINT('Ctrl Pts',(-3.76639763409716,-2.42521541658955,
5.01882514925639));
#15049=CARTESIAN_POINT('Ctrl Pts',(-3.76104161906272,-2.45036494470439,
5.02050226217376));
#15050=CARTESIAN_POINT('Ctrl Pts',(-3.75014621732021,-2.47282762178721,
5.02217937509113));
#15051=CARTESIAN_POINT('Ctrl Pts',(-3.72607922389733,-2.52244571888807,
5.0258839714434));
#15052=CARTESIAN_POINT('Ctrl Pts',(-3.67498392204337,-2.55895387399913,
5.02958856779567));
#15053=CARTESIAN_POINT('Ctrl Pts',(-3.62024436531629,-2.56564393553624,
5.03329316414794));
#15054=CARTESIAN_POINT('Ctrl Pts',(-3.5655048085892,-2.57233399707334,5.03699776050021));
#15055=CARTESIAN_POINT('Ctrl Pts',(-3.50712099698899,-2.54920596503651,
5.04070235685248));
#15056=CARTESIAN_POINT('Ctrl Pts',(-3.47181261508692,-2.50684448916664,
5.04440695320474));
#15057=CARTESIAN_POINT('Ctrl Pts',(-3.43650423318484,-2.46448301329678,
5.04811154955701));
#15058=CARTESIAN_POINT('Ctrl Pts',(-3.42427128098091,-2.4028880935939,5.05181614590928));
#15059=CARTESIAN_POINT('Ctrl Pts',(-3.44071223414431,-2.35024904491843,
5.05552074226155));
#15060=CARTESIAN_POINT('Ctrl Pts',(-3.45715318730771,-2.29760999624296,
5.05922533861381));
#15061=CARTESIAN_POINT('Ctrl Pts',(-3.50226804583846,-2.2539268185949,5.06292993496608));
#15062=CARTESIAN_POINT('Ctrl Pts',(-3.55540974746646,-2.23919126462175,
5.06663453131835));
#15063=CARTESIAN_POINT('Ctrl Pts',(-3.60855144909447,-2.2244557106486,5.07033912767062));
#15064=CARTESIAN_POINT('Ctrl Pts',(-3.66971999381974,-2.23866778035036,
5.07404372402289));
#15065=CARTESIAN_POINT('Ctrl Pts',(-3.71092123316877,-2.27532344228896,
5.07774832037516));
#15066=CARTESIAN_POINT('Ctrl Pts',(-3.74576802981578,-2.30632572323287,
5.08088155902978));
#15067=CARTESIAN_POINT('Ctrl Pts',(-3.76633165591099,-2.35338253179949,
5.0840147976844));
#15068=CARTESIAN_POINT('Ctrl Pts',(-3.76673281282141,-2.40013003219325,
5.08714803633902));
#15069=CARTESIAN_POINT('Origin',(-3.6,-2.4,4.7));
#15070=CARTESIAN_POINT('',(-3.76674783764939,-2.3998784327954,5.15714803633902));
#15071=CARTESIAN_POINT('',(-3.76638442554721,-2.39990578503699,5.13785196366098));
#15072=CARTESIAN_POINT('',(-3.7666,-2.4,4.7));
#15073=CARTESIAN_POINT('',(-3.47309291201476,-2.29206413469515,5.2));
#15074=CARTESIAN_POINT('Ctrl Pts',(-3.76674783764939,-2.3998784327954,5.15714803633902));
#15075=CARTESIAN_POINT('Ctrl Pts',(-3.7663543041176,-2.44715561431286,5.16031823516921));
#15076=CARTESIAN_POINT('Ctrl Pts',(-3.74524548348422,-2.49473161213543,
5.1634884339994));
#15077=CARTESIAN_POINT('Ctrl Pts',(-3.70967617757414,-2.52575977295725,
5.16665863282959));
#15078=CARTESIAN_POINT('Ctrl Pts',(-3.66811098624533,-2.56201832251683,
5.17036322918186));
#15079=CARTESIAN_POINT('Ctrl Pts',(-3.60679922558629,-2.57567991185357,
5.17406782553412));
#15080=CARTESIAN_POINT('Ctrl Pts',(-3.55380862744679,-2.56038491971217,
5.17777242188639));
#15081=CARTESIAN_POINT('Ctrl Pts',(-3.5008180293073,-2.54508992757078,5.18147701823866));
#15082=CARTESIAN_POINT('Ctrl Pts',(-3.45614859368735,-2.50083835395125,
5.18518161459093));
#15083=CARTESIAN_POINT('Ctrl Pts',(-3.44024450358536,-2.44813181223257,
5.1888862109432));
#15084=CARTESIAN_POINT('Ctrl Pts',(-3.42434041348337,-2.39542527051388,
5.19259080729547));
#15085=CARTESIAN_POINT('Ctrl Pts',(-3.43720166889934,-2.33426376069605,
5.19629540364773));
#15086=CARTESIAN_POINT('Ctrl Pts',(-3.47309291201476,-2.29206413469515,
5.2));
#15087=CARTESIAN_POINT('',(-3.7271475418302,-2.29187968016137,5.2));
#15088=CARTESIAN_POINT('Origin',(-3.6,-2.4,5.2));
#15089=CARTESIAN_POINT('Ctrl Pts',(-3.72714769448933,-2.29187956305504,
5.2));
#15090=CARTESIAN_POINT('Ctrl Pts',(-3.69206190113039,-2.25072743961435,
5.19636770818144));
#15091=CARTESIAN_POINT('Ctrl Pts',(-3.6350641341643,-2.22812240899828,5.19273541636289));
#15092=CARTESIAN_POINT('Ctrl Pts',(-3.58132375070445,-2.23418207790235,
5.18910312454434));
#15093=CARTESIAN_POINT('Ctrl Pts',(-3.52651360920706,-2.24036237079714,
5.18539852819207));
#15094=CARTESIAN_POINT('Ctrl Pts',(-3.47509182514536,-2.27635992272048,
5.1816939318398));
#15095=CARTESIAN_POINT('Ctrl Pts',(-3.45055836147391,-2.3257410419838,5.17798933548753));
#15096=CARTESIAN_POINT('Ctrl Pts',(-3.42602489780247,-2.37512216124712,
5.17428473913526));
#15097=CARTESIAN_POINT('Ctrl Pts',(-3.42837975452128,-2.43788684785041,
5.170580142783));
#15098=CARTESIAN_POINT('Ctrl Pts',(-3.45656193213921,-2.48529019920904,
5.16687554643073));
#15099=CARTESIAN_POINT('Ctrl Pts',(-3.48474410975714,-2.53269355056767,
5.16317095007846));
#15100=CARTESIAN_POINT('Ctrl Pts',(-3.53875360827419,-2.56473556668165,
5.15946635372619));
#15101=CARTESIAN_POINT('Ctrl Pts',(-3.59386432904901,-2.56676216280164,
5.15576175737392));
#15102=CARTESIAN_POINT('Ctrl Pts',(-3.64897504982384,-2.56878875892163,
5.15205716102165));
#15103=CARTESIAN_POINT('Ctrl Pts',(-3.70518699285644,-2.54079993504764,
5.14835256466939));
#15104=CARTESIAN_POINT('Ctrl Pts',(-3.73677861120293,-2.49559987891255,
5.14464796831712));
#15105=CARTESIAN_POINT('Ctrl Pts',(-3.75609666594378,-2.46796035917884,
5.14238263343174));
#15106=CARTESIAN_POINT('Ctrl Pts',(-3.76620859684834,-2.43388515114326,
5.14011729854636));
#15107=CARTESIAN_POINT('Ctrl Pts',(-3.76638442554721,-2.39990578503699,
5.13785196366098));
#15108=CARTESIAN_POINT('Origin',(-3.6,-2.4,5.35459252805377));
#15109=CARTESIAN_POINT('',(-3.8057227013582,-2.39988044337606,4.34540747194623));
#15110=CARTESIAN_POINT('',(-3.80516111137892,-2.40008013262119,4.33959252805377));
#15111=CARTESIAN_POINT('',(-3.805475,-2.39999999999999,5.35459252805377));
#15112=CARTESIAN_POINT('',(-3.41173724903364,-2.48232321801035,4.3));
#15113=CARTESIAN_POINT('Ctrl Pts',(-3.80516111137892,-2.40008013262119,
4.33959252805377));
#15114=CARTESIAN_POINT('Ctrl Pts',(-3.80504330063484,-2.36152007992449,
4.33750880775931));
#15115=CARTESIAN_POINT('Ctrl Pts',(-3.77605833105766,-2.25423615375421,
4.33172049111259));
#15116=CARTESIAN_POINT('Ctrl Pts',(-3.60297473301061,-2.15700944143379,
4.32222757811361));
#15117=CARTESIAN_POINT('Ctrl Pts',(-3.39749761512046,-2.26611614077921,
4.3111137890568));
#15118=CARTESIAN_POINT('Ctrl Pts',(-3.38436282049399,-2.419721374356,4.30370459635227));
#15119=CARTESIAN_POINT('Ctrl Pts',(-3.41173724903364,-2.48232321801035,
4.3));
#15120=CARTESIAN_POINT('',(-3.47764162637991,-2.56553534042572,4.3));
#15121=CARTESIAN_POINT('Origin',(-3.6,-2.4,4.3));
#15122=CARTESIAN_POINT('Ctrl Pts',(-3.8057227013582,-2.39988044337606,4.34540747194623));
#15123=CARTESIAN_POINT('Ctrl Pts',(-3.8057729696998,-2.39271640638513,4.34501772883951));
#15124=CARTESIAN_POINT('Ctrl Pts',(-3.80218373546239,-2.3175070024762,4.34092338938053));
#15125=CARTESIAN_POINT('Ctrl Pts',(-3.70962995644976,-2.18326697275372,
4.33312445356927));
#15126=CARTESIAN_POINT('Ctrl Pts',(-3.47734459894833,-2.19039236572141,
4.32201066451247));
#15127=CARTESIAN_POINT('Ctrl Pts',(-3.35820162590419,-2.3879909133699,4.31096917998938));
#15128=CARTESIAN_POINT('Ctrl Pts',(-3.42405718781536,-2.52582031335719,
4.30363229181855));
#15129=CARTESIAN_POINT('Ctrl Pts',(-3.47764149510761,-2.56553553810743,
4.3));
#15130=CARTESIAN_POINT('Origin',(-3.6,-2.4,5.35459252805377));
#15131=CARTESIAN_POINT('',(-3.80519266468163,-2.39989734570579,4.41540747194623));
#15132=CARTESIAN_POINT('',(-3.80566724789774,-2.40014978098439,4.40959252805377));
#15133=CARTESIAN_POINT('',(-3.805475,-2.39999999999999,5.35459252805377));
#15134=CARTESIAN_POINT('Ctrl Pts',(-3.80566724789774,-2.40014978098439,
4.40959252805377));
#15135=CARTESIAN_POINT('Ctrl Pts',(-3.80518614471975,-2.34148051217519,
4.40640305253959));
#15136=CARTESIAN_POINT('Ctrl Pts',(-3.74813829229662,-2.21384966330463,
4.39950898067315));
#15137=CARTESIAN_POINT('Ctrl Pts',(-3.53156901893564,-2.16697244735031,
4.38891031245443));
#15138=CARTESIAN_POINT('Ctrl Pts',(-3.36710794136624,-2.33111753922242,
4.37779652339762));
#15139=CARTESIAN_POINT('Ctrl Pts',(-3.41581894666805,-2.55829572590735,
4.36668273434083));
#15140=CARTESIAN_POINT('Ctrl Pts',(-3.63310626972243,-2.64061568298545,
4.35556894528402));
#15141=CARTESIAN_POINT('Ctrl Pts',(-3.7850442261316,-2.5285041432322,4.34653887652167));
#15142=CARTESIAN_POINT('Ctrl Pts',(-3.80525275353212,-2.43007507309885,
4.34121340411158));
#15143=CARTESIAN_POINT('Ctrl Pts',(-3.80516111137892,-2.40008013262119,
4.33959252805377));
#15144=CARTESIAN_POINT('Ctrl Pts',(-3.80519266468163,-2.39989734570579,
4.41540747194623));
#15145=CARTESIAN_POINT('Ctrl Pts',(-3.80531782889597,-2.37222562131849,
4.41391197361979));
#15146=CARTESIAN_POINT('Ctrl Pts',(-3.78721617857279,-2.2761634023784,4.40871187894108));
#15147=CARTESIAN_POINT('Ctrl Pts',(-3.64121277969171,-2.16065653443092,
4.3998071879101));
#15148=CARTESIAN_POINT('Ctrl Pts',(-3.42126523797479,-2.23556891230323,
4.38869339885329));
#15149=CARTESIAN_POINT('Ctrl Pts',(-3.36491711226222,-2.46098554747977,
4.37757960979649));
#15150=CARTESIAN_POINT('Ctrl Pts',(-3.52374009350676,-2.63058418685777,
4.36646582073969));
#15151=CARTESIAN_POINT('Ctrl Pts',(-3.74435278297668,-2.59057501347053,
4.3557417747896));
#15152=CARTESIAN_POINT('Ctrl Pts',(-3.80529515774691,-2.46081219780934,
4.34872232519178));
#15153=CARTESIAN_POINT('Ctrl Pts',(-3.8057227013582,-2.39988044337606,4.34540747194623));
#15154=CARTESIAN_POINT('Origin',(-3.6,-2.4,5.35459252805377));
#15155=CARTESIAN_POINT('',(-3.80534991328218,-2.40017652766129,4.48540747194623));
#15156=CARTESIAN_POINT('',(-3.80562878759967,-2.39983660975823,4.47959252805377));
#15157=CARTESIAN_POINT('',(-3.805475,-2.39999999999999,5.35459252805377));
#15158=CARTESIAN_POINT('Ctrl Pts',(-3.80562878759967,-2.39983660975823,
4.47959252805377));
#15159=CARTESIAN_POINT('Ctrl Pts',(-3.80572325938657,-2.3889667780224,4.47900189367213));
#15160=CARTESIAN_POINT('Ctrl Pts',(-3.79999615684062,-2.31001856287219,
4.47470666293823));
#15161=CARTESIAN_POINT('Ctrl Pts',(-3.69773850858379,-2.17766949547173,
4.46670683585206));
#15162=CARTESIAN_POINT('Ctrl Pts',(-3.46621554409366,-2.19730464027232,
4.45559304679525));
#15163=CARTESIAN_POINT('Ctrl Pts',(-3.35714698343348,-2.40246926898597,
4.44447925773846));
#15164=CARTESIAN_POINT('Ctrl Pts',(-3.47036459479899,-2.60537350263611,
4.43336546868164));
#15165=CARTESIAN_POINT('Ctrl Pts',(-3.70223885894321,-2.62029753112878,
4.42225167962485));
#15166=CARTESIAN_POINT('Ctrl Pts',(-3.80084480548257,-2.48716469502641,
4.41432736608222));
#15167=CARTESIAN_POINT('Ctrl Pts',(-3.80574494915964,-2.40962524577001,
4.41010764889186));
#15168=CARTESIAN_POINT('Ctrl Pts',(-3.80566724789774,-2.40014978098439,
4.40959252805377));
#15169=CARTESIAN_POINT('Ctrl Pts',(-3.80534991328218,-2.40017652766129,
4.48540747194623));
#15170=CARTESIAN_POINT('Ctrl Pts',(-3.8049563333145,-2.35213729171836,4.48280621840006));
#15171=CARTESIAN_POINT('Ctrl Pts',(-3.76418777806192,-2.23508077339291,
4.47650036850163));
#15172=CARTESIAN_POINT('Ctrl Pts',(-3.56918135654791,-2.15909775573836,
4.46648992225092));
#15173=CARTESIAN_POINT('Ctrl Pts',(-3.38089013692747,-2.29524052189659,
4.45537613319412));
#15174=CARTESIAN_POINT('Ctrl Pts',(-3.39315268252002,-2.52727080497827,
4.44426234413731));
#15175=CARTESIAN_POINT('Ctrl Pts',(-3.59474487821944,-2.64280871984201,
4.43314855508051));
#15176=CARTESIAN_POINT('Ctrl Pts',(-3.77337323688511,-2.5504598261374,4.42353026435015));
#15177=CARTESIAN_POINT('Ctrl Pts',(-3.80500777646484,-2.44077305290937,
4.41761656997206));
#15178=CARTESIAN_POINT('Ctrl Pts',(-3.80519266468163,-2.39989734570579,
4.41540747194623));
#15179=CARTESIAN_POINT('Origin',(-3.6,-2.4,5.35459252805377));
#15180=CARTESIAN_POINT('',(-3.80581595477291,-2.39999917227814,4.55540747194623));
#15181=CARTESIAN_POINT('',(-3.80515176250663,-2.39995310238523,4.54959252805377));
#15182=CARTESIAN_POINT('',(-3.805475,-2.39999999999999,5.35459252805377));
#15183=CARTESIAN_POINT('Ctrl Pts',(-3.80515176250663,-2.39995310238523,
4.54959252805377));
#15184=CARTESIAN_POINT('Ctrl Pts',(-3.80521587176166,-2.36854855820361,
4.54789613845241));
#15185=CARTESIAN_POINT('Ctrl Pts',(-3.78367651299531,-2.26864576859469,
4.54249515249878));
#15186=CARTESIAN_POINT('Ctrl Pts',(-3.62821111895818,-2.15877850380716,
4.53338957019289));
#15187=CARTESIAN_POINT('Ctrl Pts',(-3.4126363777684,-2.24547313898512,4.52227578113608));
#15188=CARTESIAN_POINT('Ctrl Pts',(-3.3685576844537,-2.47360796440317,4.51116199207928));
#15189=CARTESIAN_POINT('Ctrl Pts',(-3.53632076809686,-2.63436858142862,
4.50004820302248));
#15190=CARTESIAN_POINT('Ctrl Pts',(-3.75035693907624,-2.58346600089298,
4.4895250483473));
#15191=CARTESIAN_POINT('Ctrl Pts',(-3.80513071034435,-2.45714489336835,
4.4827064900244));
#15192=CARTESIAN_POINT('Ctrl Pts',(-3.80562878759967,-2.39983660975823,
4.47959252805377));
#15193=CARTESIAN_POINT('Ctrl Pts',(-3.80581595309039,-2.39999917228222,
4.55540747194623));
#15194=CARTESIAN_POINT('Ctrl Pts',(-3.80581595573579,-2.39995488126346,
4.55540505953261));
#15195=CARTESIAN_POINT('Ctrl Pts',(-3.805795885724,-2.33189557869137,4.55169805076671));
#15196=CARTESIAN_POINT('Ctrl Pts',(-3.73158417960078,-2.19586944742698,
4.54428644564855));
#15197=CARTESIAN_POINT('Ctrl Pts',(-3.49986236155564,-2.17873967321655,
4.53317265659175));
#15198=CARTESIAN_POINT('Ctrl Pts',(-3.35979765944108,-2.36413198553984,
4.52205886753494));
#15199=CARTESIAN_POINT('Ctrl Pts',(-3.43959288407154,-2.58235469793693,
4.51094507847814));
#15200=CARTESIAN_POINT('Ctrl Pts',(-3.66621056034765,-2.6336660879353,4.49983128942134));
#15201=CARTESIAN_POINT('Ctrl Pts',(-3.79336822690886,-2.50914983096546,
4.4913187539107));
#15202=CARTESIAN_POINT('Ctrl Pts',(-3.80551685342017,-2.42055275952314,
4.48651081475233));
#15203=CARTESIAN_POINT('Ctrl Pts',(-3.80534991328218,-2.40017652766129,
4.48540747194623));
#15204=CARTESIAN_POINT('Origin',(-3.6,-2.4,5.35459252805377));
#15205=CARTESIAN_POINT('',(-3.80534749847032,-2.39982399268994,4.62540747194623));
#15206=CARTESIAN_POINT('',(-3.80545680064795,-2.40018789159516,4.61959252805377));
#15207=CARTESIAN_POINT('',(-3.805475,-2.39999999999999,5.35459252805377));
#15208=CARTESIAN_POINT('Ctrl Pts',(-3.80545680064795,-2.40018789159516,
4.61959252805377));
#15209=CARTESIAN_POINT('Ctrl Pts',(-3.80498629881388,-2.34850704133116,
4.61679038323269));
#15210=CARTESIAN_POINT('Ctrl Pts',(-3.75902064354221,-2.22775548399901,
4.61028364205933));
#15211=CARTESIAN_POINT('Ctrl Pts',(-3.55620097341096,-2.16111650777606,
4.60007230453371));
#15212=CARTESIAN_POINT('Ctrl Pts',(-3.37554637252617,-2.307240921179,4.58895851547691));
#15213=CARTESIAN_POINT('Ctrl Pts',(-3.40033672233922,-2.53826877141577,
4.57784472642011));
#15214=CARTESIAN_POINT('Ctrl Pts',(-3.60788113454322,-2.64273764704216,
4.5667309373633));
#15215=CARTESIAN_POINT('Ctrl Pts',(-3.7776337191139,-2.54299330423865,4.55731353790786));
#15216=CARTESIAN_POINT('Ctrl Pts',(-3.80507586918669,-2.43713018575349,
4.55160073480468));
#15217=CARTESIAN_POINT('Ctrl Pts',(-3.80515176250663,-2.39995310238523,
4.54959252805377));
#15218=CARTESIAN_POINT('Ctrl Pts',(-3.80534749847032,-2.39982399268994,
4.62540747194623));
#15219=CARTESIAN_POINT('Ctrl Pts',(-3.8055145307928,-2.37935804813576,4.62429930431288));
#15220=CARTESIAN_POINT('Ctrl Pts',(-3.79329841632202,-2.29066951260838,
4.61948654032727));
#15221=CARTESIAN_POINT('Ctrl Pts',(-3.66590691978443,-2.16624808716256,
4.61096917998938));
#15222=CARTESIAN_POINT('Ctrl Pts',(-3.4393560992794,-2.21785386089149,4.59985539093257));
#15223=CARTESIAN_POINT('Ctrl Pts',(-3.35984446292695,-2.43618006142673,
4.58874160187577));
#15224=CARTESIAN_POINT('Ctrl Pts',(-3.50014991321196,-2.62139024142312,
4.57762781281897));
#15225=CARTESIAN_POINT('Ctrl Pts',(-3.73179898649779,-2.60396320633826,
4.56651643617578));
#15226=CARTESIAN_POINT('Ctrl Pts',(-3.80581189336919,-2.46796989528688,
4.55910965588487));
#15227=CARTESIAN_POINT('Ctrl Pts',(-3.80581595309039,-2.39999917228222,
4.55540747194623));
#15228=CARTESIAN_POINT('Origin',(-3.6,-2.4,5.35459252805377));
#15229=CARTESIAN_POINT('',(-3.80519404433776,-2.40010391087563,4.69540747194623));
#15230=CARTESIAN_POINT('',(-3.80578860319875,-2.39993212258736,4.68959252805377));
#15231=CARTESIAN_POINT('',(-3.805475,-2.39999999999999,5.35459252805377));
#15232=CARTESIAN_POINT('Ctrl Pts',(-3.80578860319875,-2.39993212258736,
4.68959252805377));
#15233=CARTESIAN_POINT('Ctrl Pts',(-3.80580467529652,-2.39619821380325,
4.68938922436523));
#15234=CARTESIAN_POINT('Ctrl Pts',(-3.8040203847709,-2.32444075317719,4.68548132432442));
#15235=CARTESIAN_POINT('Ctrl Pts',(-3.72035445765201,-2.18905336667194,
4.67786882793134));
#15236=CARTESIAN_POINT('Ctrl Pts',(-3.4880454122232,-2.18447773232253,4.66675503887454));
#15237=CARTESIAN_POINT('Ctrl Pts',(-3.35820967063793,-2.37717207376684,
4.65564124981773));
#15238=CARTESIAN_POINT('Ctrl Pts',(-3.4496873596065,-2.5907610749791,4.64452746076093));
#15239=CARTESIAN_POINT('Ctrl Pts',(-3.67874791298872,-2.62974430088435,
4.63341367170412));
#15240=CARTESIAN_POINT('Ctrl Pts',(-3.79614945789441,-2.50163131370898,
4.62510202746841));
#15241=CARTESIAN_POINT('Ctrl Pts',(-3.80560832925468,-2.41683209288794,
4.62049497958495));
#15242=CARTESIAN_POINT('Ctrl Pts',(-3.80545680064795,-2.40018789159516,
4.61959252805377));
#15243=CARTESIAN_POINT('Ctrl Pts',(-3.80519404433776,-2.40010391087563,
4.69540747194623));
#15244=CARTESIAN_POINT('Ctrl Pts',(-3.80500644622954,-2.35913959443751,
4.69319354909316));
#15245=CARTESIAN_POINT('Ctrl Pts',(-3.77326723416865,-2.24936122008858,
4.68727502988781));
#15246=CARTESIAN_POINT('Ctrl Pts',(-3.59442944460758,-2.15719833661306,
4.6776519143302));
#15247=CARTESIAN_POINT('Ctrl Pts',(-3.3929874908777,-2.27299803191391,4.6665381252734));
#15248=CARTESIAN_POINT('Ctrl Pts',(-3.38102643442896,-2.50504406890429,
4.65542433621659));
#15249=CARTESIAN_POINT('Ctrl Pts',(-3.5694943658766,-2.64094207834572,4.64431054715979));
#15250=CARTESIAN_POINT('Ctrl Pts',(-3.76430796656755,-2.56474251573525,
4.63430492573634));
#15251=CARTESIAN_POINT('Ctrl Pts',(-3.8049561429515,-2.44777555218424,4.62800390066515));
#15252=CARTESIAN_POINT('Ctrl Pts',(-3.80534749847032,-2.39982399268994,
4.62540747194623));
#15253=CARTESIAN_POINT('Origin',(-3.6,-2.4,5.35459252805377));
#15254=CARTESIAN_POINT('',(-3.80572671416466,-2.40012021867279,4.76540747194623));
#15255=CARTESIAN_POINT('',(-3.80525640542964,-2.39985490132803,4.75959252805377));
#15256=CARTESIAN_POINT('',(-3.805475,-2.39999999999999,5.35459252805377));
#15257=CARTESIAN_POINT('Ctrl Pts',(-3.80525640542964,-2.39985490132803,
4.75959252805377));
#15258=CARTESIAN_POINT('Ctrl Pts',(-3.80541421756911,-2.37565177743561,
4.7582834691455));
#15259=CARTESIAN_POINT('Ctrl Pts',(-3.7902631541036,-2.2831457592228,4.75326981388497));
#15260=CARTESIAN_POINT('Ctrl Pts',(-3.65317166084996,-2.16302647390142,
4.74455156227217));
#15261=CARTESIAN_POINT('Ctrl Pts',(-3.42974254509416,-2.22680624538361,
4.73343777321536));
#15262=CARTESIAN_POINT('Ctrl Pts',(-3.36215200866455,-2.44911222461694,
4.72232398415856));
#15263=CARTESIAN_POINT('Ctrl Pts',(-3.51226643608395,-2.62646522768789,
4.71121019510176));
#15264=CARTESIAN_POINT('Ctrl Pts',(-3.73846937161942,-2.59707960507412,
4.70029970973349));
#15265=CARTESIAN_POINT('Ctrl Pts',(-3.80551180980452,-2.46423743611441,
4.6930938207175));
#15266=CARTESIAN_POINT('Ctrl Pts',(-3.80578860319875,-2.39993212258736,
4.68959252805377));
#15267=CARTESIAN_POINT('Ctrl Pts',(-3.80572671416466,-2.40012021867279,
4.76540747194623));
#15268=CARTESIAN_POINT('Ctrl Pts',(-3.80530257178557,-2.33910193112031,
4.76208779387343));
#15269=CARTESIAN_POINT('Ctrl Pts',(-3.74420123427486,-2.20925254264417,
4.75506351944836));
#15270=CARTESIAN_POINT('Ctrl Pts',(-3.52344221265408,-2.16951662960737,
4.74433464867103));
#15271=CARTESIAN_POINT('Ctrl Pts',(-3.36483725976158,-2.33931915924769,
4.73322085961422));
#15272=CARTESIAN_POINT('Ctrl Pts',(-3.42147942993616,-2.56466355059616,
4.72210707055742));
#15273=CARTESIAN_POINT('Ctrl Pts',(-3.64152350245114,-2.63928952667227,
4.71099328150061));
#15274=CARTESIAN_POINT('Ctrl Pts',(-3.78729792557216,-2.52365598332802,
4.70209341529689));
#15275=CARTESIAN_POINT('Ctrl Pts',(-3.80532035746924,-2.42768591123397,
4.69689814544542));
#15276=CARTESIAN_POINT('Ctrl Pts',(-3.80519404433776,-2.40010391087563,
4.69540747194623));
#15277=CARTESIAN_POINT('Origin',(-3.6,-2.4,5.35459252805377));
#15278=CARTESIAN_POINT('',(-3.80555826192291,-2.39982008596012,4.83540747194623));
#15279=CARTESIAN_POINT('',(-3.80526423797111,-2.40014879660671,4.82959252805377));
#15280=CARTESIAN_POINT('',(-3.805475,-2.39999999999999,5.35459252805377));
#15281=CARTESIAN_POINT('Ctrl Pts',(-3.80526423797112,-2.40014879660671,
4.82959252805377));
#15282=CARTESIAN_POINT('Ctrl Pts',(-3.80496497000794,-2.35550570352956,
4.82717771392578));
#15283=CARTESIAN_POINT('Ctrl Pts',(-3.7687007786119,-2.24193241424781,4.82105830344552));
#15284=CARTESIAN_POINT('Ctrl Pts',(-3.58130943002562,-2.15785471265546,
4.81123429661298));
#15285=CARTESIAN_POINT('Ctrl Pts',(-3.38642338383962,-2.28437687679961,
4.8001205075562));
#15286=CARTESIAN_POINT('Ctrl Pts',(-3.38702643654876,-2.51673019686447,
4.78900671849938));
#15287=CARTESIAN_POINT('Ctrl Pts',(-3.58256660716932,-2.64223904392882,
4.77789292944258));
#15288=CARTESIAN_POINT('Ctrl Pts',(-3.76915216315368,-2.5573566497576,4.76808819929404));
#15289=CARTESIAN_POINT('Ctrl Pts',(-3.80496761407973,-2.44414587187183,
4.76198806549777));
#15290=CARTESIAN_POINT('Ctrl Pts',(-3.80525640542964,-2.39985490132803,
4.75959252805377));
#15291=CARTESIAN_POINT('Ctrl Pts',(-3.80555826192291,-2.39982008596012,
4.83540747194623));
#15292=CARTESIAN_POINT('Ctrl Pts',(-3.80567994930423,-2.38654227868304,
4.83468663500597));
#15293=CARTESIAN_POINT('Ctrl Pts',(-3.79845786380229,-2.30515766788849,
4.83026120171345));
#15294=CARTESIAN_POINT('Ctrl Pts',(-3.68988494304833,-2.17438001896094,
4.82213117206866));
#15295=CARTESIAN_POINT('Ctrl Pts',(-3.45919253805822,-2.20211888040452,
4.81101738301185));
#15296=CARTESIAN_POINT('Ctrl Pts',(-3.35738279984868,-2.41098057473832,
4.79990359395505));
#15297=CARTESIAN_POINT('Ctrl Pts',(-3.47764333640382,-2.60979162448597,
4.78878980489824));
#15298=CARTESIAN_POINT('Ctrl Pts',(-3.7098983147675,-2.61657802114276,4.77767601584144));
#15299=CARTESIAN_POINT('Ctrl Pts',(-3.80223426786157,-2.48231400602396,
4.76988190485744));
#15300=CARTESIAN_POINT('Ctrl Pts',(-3.80577589367883,-2.40719531865107,
4.7657923902257));
#15301=CARTESIAN_POINT('Ctrl Pts',(-3.80572671416466,-2.40012021867279,
4.76540747194623));
#15302=CARTESIAN_POINT('Origin',(-3.6,-2.4,5.35459252805377));
#15303=CARTESIAN_POINT('',(-3.80514217248594,-2.39999218980904,4.90540747194623));
#15304=CARTESIAN_POINT('',(-3.80579332868662,-2.40006173798069,4.89959252805377));
#15305=CARTESIAN_POINT('',(-3.805475,-2.39999999999999,5.35459252805377));
#15306=CARTESIAN_POINT('Ctrl Pts',(-3.80579332868662,-2.40006173798069,
4.89959252805377));
#15307=CARTESIAN_POINT('Ctrl Pts',(-3.80553739175956,-2.33540634391997,
4.89607195870605));
#15308=CARTESIAN_POINT('Ctrl Pts',(-3.73784442753819,-2.20225412798971,
4.88884679300607));
#15309=CARTESIAN_POINT('Ctrl Pts',(-3.511092084609,-2.17399322981363,4.87791703095382));
#15310=CARTESIAN_POINT('Ctrl Pts',(-3.36190028176488,-2.35212305601353,
4.86680324189701));
#15311=CARTESIAN_POINT('Ctrl Pts',(-3.43064385125587,-2.57407519200526,
4.85568945284021));
#15312=CARTESIAN_POINT('Ctrl Pts',(-3.6544010243217,-2.63669433060785,4.84457566378341));
#15313=CARTESIAN_POINT('Ctrl Pts',(-3.79056542018395,-2.51613221267343,
4.83587668885459));
#15314=CARTESIAN_POINT('Ctrl Pts',(-3.80542408070796,-2.42399322720708,
4.83088231027805));
#15315=CARTESIAN_POINT('Ctrl Pts',(-3.80526423797112,-2.40014879660671,
4.82959252805377));
#15316=CARTESIAN_POINT('Ctrl Pts',(-3.80514217248594,-2.39999218980904,
4.90540747194623));
#15317=CARTESIAN_POINT('Ctrl Pts',(-3.80515363847659,-2.36617331522009,
4.90358087978625));
#15318=CARTESIAN_POINT('Ctrl Pts',(-3.78123591841218,-2.26378007899297,
4.898049691274));
#15319=CARTESIAN_POINT('Ctrl Pts',(-3.61973808033182,-2.15793784472475,
4.88881390640949));
#15320=CARTESIAN_POINT('Ctrl Pts',(-3.4073347883606,-2.25213588990288,4.87770011735268));
#15321=CARTESIAN_POINT('Ctrl Pts',(-3.37128014957741,-2.48167563194308,
4.86658632829587));
#15322=CARTESIAN_POINT('Ctrl Pts',(-3.54457538374435,-2.63645674180255,
4.85547253923907));
#15323=CARTESIAN_POINT('Ctrl Pts',(-3.75407113935919,-2.57880494205606,
4.84507958712253));
#15324=CARTESIAN_POINT('Ctrl Pts',(-3.8050545615032,-2.45478089640322,4.83839123135824));
#15325=CARTESIAN_POINT('Ctrl Pts',(-3.80555826192291,-2.39982008596012,
4.83540747194623));
#15326=CARTESIAN_POINT('Origin',(-3.6,-2.4,5.35459252805377));
#15327=CARTESIAN_POINT('',(-3.80552959282545,-2.40018396914357,4.97540747194623));
#15328=CARTESIAN_POINT('',(-3.80544614170703,-2.39981229694107,4.96959252805377));
#15329=CARTESIAN_POINT('',(-3.805475,-2.39999999999999,5.35459252805377));
#15330=CARTESIAN_POINT('Ctrl Pts',(-3.80544614170703,-2.39981229694107,
4.96959252805377));
#15331=CARTESIAN_POINT('Ctrl Pts',(-3.80560005255251,-2.38281031937819,
4.9686707998386));
#15332=CARTESIAN_POINT('Ctrl Pts',(-3.79589308932397,-2.29764759199308,
4.96404447527115));
#15333=CARTESIAN_POINT('Ctrl Pts',(-3.67755429765177,-2.16985003043886,
4.95571355435145));
#15334=CARTESIAN_POINT('Ctrl Pts',(-3.44869918397279,-2.21002173633656,
4.94459976529464));
#15335=CARTESIAN_POINT('Ctrl Pts',(-3.3583314230664,-2.42408270152555,4.93348597623784));
#15336=CARTESIAN_POINT('Ctrl Pts',(-3.48916565133794,-2.61610049686178,
4.92237218718103));
#15337=CARTESIAN_POINT('Ctrl Pts',(-3.7214478158856,-2.61031905668909,4.91125839812423));
#15338=CARTESIAN_POINT('Ctrl Pts',(-3.80419976839027,-2.4748431306509,4.90366517841514));
#15339=CARTESIAN_POINT('Ctrl Pts',(-3.8058067070074,-2.4034414011323,4.89977655505832));
#15340=CARTESIAN_POINT('Ctrl Pts',(-3.80579332868662,-2.40006173798069,
4.89959252805377));
#15341=CARTESIAN_POINT('Ctrl Pts',(-3.80552959282545,-2.40018396914357,
4.97540747194623));
#15342=CARTESIAN_POINT('Ctrl Pts',(-3.80503093302249,-2.34615078230832,
4.97247512456653));
#15343=CARTESIAN_POINT('Ctrl Pts',(-3.75549941719541,-2.22304560401132,
4.96583818083455));
#15344=CARTESIAN_POINT('Ctrl Pts',(-3.54785414492032,-2.16279863265717,
4.9554966407503));
#15345=CARTESIAN_POINT('Ctrl Pts',(-3.37243276525931,-2.31516585290104,
4.94438285169351));
#15346=CARTESIAN_POINT('Ctrl Pts',(-3.40530625649813,-2.54518272988275,
4.9332690626367));
#15347=CARTESIAN_POINT('Ctrl Pts',(-3.61638513906469,-2.64231220781178,
4.9221552735799));
#15348=CARTESIAN_POINT('Ctrl Pts',(-3.78023982132068,-2.53813917250258,
4.91286807668307));
#15349=CARTESIAN_POINT('Ctrl Pts',(-3.80513038376869,-2.43476294468685,
4.90728547613852));
#15350=CARTESIAN_POINT('Ctrl Pts',(-3.80514217248594,-2.39999218980904,
4.90540747194623));
#15351=CARTESIAN_POINT('Origin',(-3.6,-2.4,5.35459252805377));
#15352=CARTESIAN_POINT('',(-3.80574710647333,-2.39989343748479,5.04540747194623));
#15353=CARTESIAN_POINT('',(-3.80515433874078,-2.40005255540964,5.03959252805377));
#15354=CARTESIAN_POINT('',(-3.805475,-2.39999999999999,5.35459252805377));
#15355=CARTESIAN_POINT('Ctrl Pts',(-3.80515433874078,-2.40005255540964,
5.03959252805377));
#15356=CARTESIAN_POINT('Ctrl Pts',(-3.80506841571452,-2.36251978652027,
5.03756504461887));
#15357=CARTESIAN_POINT('Ctrl Pts',(-3.77723760351786,-2.25628892207963,
5.0318329648317));
#15358=CARTESIAN_POINT('Ctrl Pts',(-3.60662102802227,-2.15722471599323,
5.02239628869228));
#15359=CARTESIAN_POINT('Ctrl Pts',(-3.39962168818772,-2.262769500459,5.01128249963546));
#15360=CARTESIAN_POINT('Ctrl Pts',(-3.37603088927244,-2.49392292132789,
5.00016871057867));
#15361=CARTESIAN_POINT('Ctrl Pts',(-3.55744155755193,-2.63910762521254,
4.98905492152185));
#15362=CARTESIAN_POINT('Ctrl Pts',(-3.75953036700652,-2.57154453779223,
4.97886286068023));
#15363=CARTESIAN_POINT('Ctrl Pts',(-3.80498145636834,-2.45114441507362,
4.97237539619086));
#15364=CARTESIAN_POINT('Ctrl Pts',(-3.80544614170703,-2.39981229694107,
4.96959252805377));
#15365=CARTESIAN_POINT('Ctrl Pts',(-3.80574710647333,-2.39989343748479,
5.04540747194623));
#15366=CARTESIAN_POINT('Ctrl Pts',(-3.80578578950289,-2.39376493044645,
5.04507396569907));
#15367=CARTESIAN_POINT('Ctrl Pts',(-3.80275768152815,-2.31959956136467,
5.04103586309964));
#15368=CARTESIAN_POINT('Ctrl Pts',(-3.71288602579316,-2.18496415245566,
5.03329316414794));
#15369=CARTESIAN_POINT('Ctrl Pts',(-3.4805593716682,-2.1885345970333,5.02217937509112));
#15370=CARTESIAN_POINT('Ctrl Pts',(-3.35755805936012,-2.38566174720256,
5.01106558603434));
#15371=CARTESIAN_POINT('Ctrl Pts',(-3.45646661470834,-2.59591285074103,
4.99995179697752));
#15372=CARTESIAN_POINT('Ctrl Pts',(-3.68675290044432,-2.62684270619768,
4.98883800792072));
#15373=CARTESIAN_POINT('Ctrl Pts',(-3.79782383930996,-2.49676322878239,
4.98065656624362));
#15374=CARTESIAN_POINT('Ctrl Pts',(-3.80566091748472,-2.41441389064144,
4.9761797209188));
#15375=CARTESIAN_POINT('Ctrl Pts',(-3.80552959282545,-2.40018396914357,
4.97540747194623));
#15376=CARTESIAN_POINT('Origin',(-3.6,-2.4,5.35459252805377));
#15377=CARTESIAN_POINT('',(-3.80520912268496,-2.39988380060309,5.11540747194623));
#15378=CARTESIAN_POINT('',(-3.8056388038084,-2.40016037433918,5.10959252805377));
#15379=CARTESIAN_POINT('',(-3.805475,-2.39999999999999,5.35459252805377));
#15380=CARTESIAN_POINT('Ctrl Pts',(-3.8056388038084,-2.40016037433918,5.10959252805377));
#15381=CARTESIAN_POINT('Ctrl Pts',(-3.80514403960571,-2.34250465619148,
5.10645928939915));
#15382=CARTESIAN_POINT('Ctrl Pts',(-3.74979516025411,-2.21584695448232,
5.09962145439226));
#15383=CARTESIAN_POINT('Ctrl Pts',(-3.53510505567384,-2.16596525884485,
5.0890790230331));
#15384=CARTESIAN_POINT('Ctrl Pts',(-3.36817872512274,-2.32759432716241,
5.07796523397629));
#15385=CARTESIAN_POINT('Ctrl Pts',(-3.41344101541272,-2.5554973786501,5.06685144491949));
#15386=CARTESIAN_POINT('Ctrl Pts',(-3.62946287054873,-2.64107179130501,
5.05573765586269));
#15387=CARTESIAN_POINT('Ctrl Pts',(-3.78402795903722,-2.53063333570257,
5.04665135024078));
#15388=CARTESIAN_POINT('Ctrl Pts',(-3.80522541336203,-2.43109926604885,
5.04126964097114));
#15389=CARTESIAN_POINT('Ctrl Pts',(-3.80515433874078,-2.40005255540964,
5.03959252805377));
#15390=CARTESIAN_POINT('Ctrl Pts',(-3.80520912268496,-2.39988380060309,
5.11540747194623));
#15391=CARTESIAN_POINT('Ctrl Pts',(-3.80534690105405,-2.37325776244818,
5.11396821047934));
#15392=CARTESIAN_POINT('Ctrl Pts',(-3.78816006360229,-2.27826799235566,
5.10882435266019));
#15393=CARTESIAN_POINT('Ctrl Pts',(-3.64483147519039,-2.16130911215383,
5.09997589848876));
#15394=CARTESIAN_POINT('Ctrl Pts',(-3.42377645640768,-2.23288040078699,
5.08886210943196));
#15395=CARTESIAN_POINT('Ctrl Pts',(-3.36401956629289,-2.45741970591997,
5.07774832037515));
#15396=CARTESIAN_POINT('Ctrl Pts',(-3.52025888222192,-2.62940132794335,
5.06663453131835));
#15397=CARTESIAN_POINT('Ctrl Pts',(-3.74260711073009,-2.59254976529191,
5.05585424850871));
#15398=CARTESIAN_POINT('Ctrl Pts',(-3.8053560973714,-2.46184055125472,5.04877856205134));
#15399=CARTESIAN_POINT('Ctrl Pts',(-3.80574710647333,-2.39989343748479,
5.04540747194623));
#15400=CARTESIAN_POINT('Origin',(-3.6,-2.4,5.35459252805377));
#15401=CARTESIAN_POINT('',(-3.80526708169851,-2.40022955265959,5.18540747194623));
#15402=CARTESIAN_POINT('',(-3.80565733457988,-2.39985006589819,5.17959252805377));
#15403=CARTESIAN_POINT('',(-3.805475,-2.39999999999999,5.35459252805377));
#15404=CARTESIAN_POINT('',(-3.65301702171886,-2.59851743256717,5.2));
#15405=CARTESIAN_POINT('Ctrl Pts',(-3.65301702171886,-2.59851743256717,
5.2));
#15406=CARTESIAN_POINT('Ctrl Pts',(-3.71902879097456,-2.58088801151799,
5.19629540364773));
#15407=CARTESIAN_POINT('Ctrl Pts',(-3.79249438127854,-2.51127182149751,
5.19143122762981));
#15408=CARTESIAN_POINT('Ctrl Pts',(-3.80542872863858,-2.42165306802236,
5.18656705161189));
#15409=CARTESIAN_POINT('Ctrl Pts',(-3.80526708169851,-2.40022955265959,
5.18540747194623));
#15410=CARTESIAN_POINT('',(-3.54686845990025,-2.59887322544328,5.2));
#15411=CARTESIAN_POINT('Origin',(-3.6,-2.4,5.2));
#15412=CARTESIAN_POINT('Ctrl Pts',(-3.54686838721289,-2.59887345127292,
5.2));
#15413=CARTESIAN_POINT('Ctrl Pts',(-3.61132827149734,-2.61600531405712,
5.19636770818144));
#15414=CARTESIAN_POINT('Ctrl Pts',(-3.74930830903252,-2.58406706978518,
5.18956521753271));
#15415=CARTESIAN_POINT('Ctrl Pts',(-3.80517197262043,-2.45815906273072,
5.18276272688396));
#15416=CARTESIAN_POINT('Ctrl Pts',(-3.80565733457988,-2.39985006589818,
5.17959252805377));
#15417=CARTESIAN_POINT('Origin',(-3.6,2.4,4.7));
#15418=CARTESIAN_POINT('',(-3.76675586981256,2.39987855699196,4.38714803633902));
#15419=CARTESIAN_POINT('',(-3.76680083090633,2.40009693666208,4.36785196366098));
#15420=CARTESIAN_POINT('',(-3.7666,2.4,4.7));
#15421=CARTESIAN_POINT('',(-3.76351293272515,2.3680769545372,4.3));
#15422=CARTESIAN_POINT('Ctrl Pts',(-3.76680083090633,2.40009693666208,4.36785196366098));
#15423=CARTESIAN_POINT('Ctrl Pts',(-3.76684158871352,2.40590556800081,4.36746222055426));
#15424=CARTESIAN_POINT('Ctrl Pts',(-3.76656456795221,2.41171030753034,4.36707247744754));
#15425=CARTESIAN_POINT('Ctrl Pts',(-3.76595693377405,2.41748025837345,4.36668273434082));
#15426=CARTESIAN_POINT('Ctrl Pts',(-3.76018123352143,2.47232494575256,4.36297813798855));
#15427=CARTESIAN_POINT('Ctrl Pts',(-3.72453483477909,2.52402649885475,4.35927354163629));
#15428=CARTESIAN_POINT('Ctrl Pts',(-3.67532197505843,2.54891439179576,4.35556894528402));
#15429=CARTESIAN_POINT('Ctrl Pts',(-3.62610911533777,2.57380228473677,4.35186434893175));
#15430=CARTESIAN_POINT('Ctrl Pts',(-3.56332979463879,2.5718765175166,4.34815975257948));
#15431=CARTESIAN_POINT('Ctrl Pts',(-3.51573443689162,2.5440364869014,4.34445515622722));
#15432=CARTESIAN_POINT('Ctrl Pts',(-3.46813907914445,2.5161964562862,4.34075055987495));
#15433=CARTESIAN_POINT('Ctrl Pts',(-3.43572768434908,2.46244216227597,4.33704596352268));
#15434=CARTESIAN_POINT('Ctrl Pts',(-3.43329507915076,2.40733835292718,4.33334136717041));
#15435=CARTESIAN_POINT('Ctrl Pts',(-3.43086247395245,2.35223454357839,4.32963677081815));
#15436=CARTESIAN_POINT('Ctrl Pts',(-3.45840865835118,2.29578121889103,4.32593217446588));
#15437=CARTESIAN_POINT('Ctrl Pts',(-3.50340586780517,2.26388777182752,4.32222757811361));
#15438=CARTESIAN_POINT('Ctrl Pts',(-3.54840307725917,2.23199432476401,4.31852298176134));
#15439=CARTESIAN_POINT('Ctrl Pts',(-3.61085131176843,2.22466075532434,4.31481838540907));
#15440=CARTESIAN_POINT('Ctrl Pts',(-3.66197498261058,2.24508842770105,4.3111137890568));
#15441=CARTESIAN_POINT('Ctrl Pts',(-3.71309865345273,2.26551610007776,4.30740919270453));
#15442=CARTESIAN_POINT('Ctrl Pts',(-3.75289776062778,2.31370501427083,4.30370459635227));
#15443=CARTESIAN_POINT('Ctrl Pts',(-3.76351293272515,2.3680769545372,4.3));
#15444=CARTESIAN_POINT('',(-3.60525668225574,2.5668198662348,4.3));
#15445=CARTESIAN_POINT('Origin',(-3.6,2.4,4.3));
#15446=CARTESIAN_POINT('',(-3.76634548976639,2.39993502697971,4.31714803633902));
#15447=CARTESIAN_POINT('Ctrl Pts',(-3.60525667864057,2.56682005840211,4.3));
#15448=CARTESIAN_POINT('Ctrl Pts',(-3.65930634748376,2.56504681426963,4.30363229181856));
#15449=CARTESIAN_POINT('Ctrl Pts',(-3.71251717627762,2.53457816039784,4.30726458363711));
#15450=CARTESIAN_POINT('Ctrl Pts',(-3.74128611123357,2.48878409483897,4.31089687545566));
#15451=CARTESIAN_POINT('Ctrl Pts',(-3.75778985504382,2.46251362194275,4.31298059575011));
#15452=CARTESIAN_POINT('Ctrl Pts',(-3.76624996614321,2.43119967804664,4.31506431604457));
#15453=CARTESIAN_POINT('Ctrl Pts',(-3.76634548976639,2.39993502697971,4.31714803633902));
#15454=CARTESIAN_POINT('',(-3.7666,2.4,4.2));
#15455=CARTESIAN_POINT('',(-3.7666,2.4,4.7));
#15456=CARTESIAN_POINT('Origin',(-3.6,2.4,4.2));
#15457=CARTESIAN_POINT('Ctrl Pts',(-3.76634548976639,2.39993502697971,4.31714803633902));
#15458=CARTESIAN_POINT('Ctrl Pts',(-3.7664197953026,2.37561500451544,4.31876891239683));
#15459=CARTESIAN_POINT('Ctrl Pts',(-3.76143276332865,2.35132480870382,4.32038978845465));
#15460=CARTESIAN_POINT('Ctrl Pts',(-3.75123332497294,2.32946153149726,4.32201066451247));
#15461=CARTESIAN_POINT('Ctrl Pts',(-3.72792197926853,2.27949187675561,4.32571526086474));
#15462=CARTESIAN_POINT('Ctrl Pts',(-3.67738233884271,2.24219983197054,4.329419857217));
#15463=CARTESIAN_POINT('Ctrl Pts',(-3.62274960712982,2.23467803877973,4.33312445356927));
#15464=CARTESIAN_POINT('Ctrl Pts',(-3.56811687541693,2.22715624558892,4.33682904992154));
#15465=CARTESIAN_POINT('Ctrl Pts',(-3.50939105241698,2.24940470399237,4.34053364627381));
#15466=CARTESIAN_POINT('Ctrl Pts',(-3.473445625673,2.29122843734541,4.34423824262608));
#15467=CARTESIAN_POINT('Ctrl Pts',(-3.43750019892903,2.33305217069845,4.34794283897834));
#15468=CARTESIAN_POINT('Ctrl Pts',(-3.42433516844104,2.39445117900107,4.35164743533061));
#15469=CARTESIAN_POINT('Ctrl Pts',(-3.43997694242044,2.44733227209049,4.35535203168288));
#15470=CARTESIAN_POINT('Ctrl Pts',(-3.45561871639985,2.50021336517992,4.35905662803515));
#15471=CARTESIAN_POINT('Ctrl Pts',(-3.50006729484665,2.54457654305613,4.36276122438742));
#15472=CARTESIAN_POINT('Ctrl Pts',(-3.55297985590111,2.56011554237715,4.36646582073968));
#15473=CARTESIAN_POINT('Ctrl Pts',(-3.60589241695558,2.57565454169817,4.37017041709195));
#15474=CARTESIAN_POINT('Ctrl Pts',(-3.6672689606177,2.562369362464,4.37387501344422));
#15475=CARTESIAN_POINT('Ctrl Pts',(-3.70902050221487,2.52634164219194,4.37757960979649));
#15476=CARTESIAN_POINT('Ctrl Pts',(-3.74496652897209,2.49532354447962,4.38076908531067));
#15477=CARTESIAN_POINT('Ctrl Pts',(-3.76636578927508,2.4474478468568,4.38395856082485));
#15478=CARTESIAN_POINT('Ctrl Pts',(-3.76675586981256,2.39987855699196,4.38714803633902));
#15479=CARTESIAN_POINT('Origin',(-3.6,2.4,4.7));
#15480=CARTESIAN_POINT('',(-3.76672468602162,2.4001324774977,4.45714803633902));
#15481=CARTESIAN_POINT('',(-3.7663710759754,2.40008323252274,4.43785196366098));
#15482=CARTESIAN_POINT('',(-3.7666,2.4,4.7));
#15483=CARTESIAN_POINT('Ctrl Pts',(-3.7663710759754,2.40008323252274,4.43785196366098));
#15484=CARTESIAN_POINT('Ctrl Pts',(-3.76647255964094,2.42251958309795,4.43635646533454));
#15485=CARTESIAN_POINT('Ctrl Pts',(-3.76225162287627,2.44491933914913,4.43486096700809));
#15486=CARTESIAN_POINT('Ctrl Pts',(-3.75352689637225,2.46540054190021,4.43336546868165));
#15487=CARTESIAN_POINT('Ctrl Pts',(-3.73191430783919,2.516135863806,4.42966087232938));
#15488=CARTESIAN_POINT('Ctrl Pts',(-3.6826649015976,2.55509827647583,4.42595627597711));
#15489=CARTESIAN_POINT('Ctrl Pts',(-3.62831779967194,2.56445627090432,4.42225167962485));
#15490=CARTESIAN_POINT('Ctrl Pts',(-3.57397069774627,2.57381426533281,4.41854708327258));
#15491=CARTESIAN_POINT('Ctrl Pts',(-3.51452590013653,2.55356784151996,4.41484248692031));
#15492=CARTESIAN_POINT('Ctrl Pts',(-3.47718895189484,2.51298317028118,4.41113789056804));
#15493=CARTESIAN_POINT('Ctrl Pts',(-3.43985200365314,2.4723984990424,4.40743329421577));
#15494=CARTESIAN_POINT('Ctrl Pts',(-3.42462290477948,2.41147558037768,4.40372869786351));
#15495=CARTESIAN_POINT('Ctrl Pts',(-3.43847074534366,2.35809557252044,4.40002410151124));
#15496=CARTESIAN_POINT('Ctrl Pts',(-3.45231858590785,2.30471556466319,4.39631950515897));
#15497=CARTESIAN_POINT('Ctrl Pts',(-3.49524336590988,2.25887846761341,4.3926149088067));
#15498=CARTESIAN_POINT('Ctrl Pts',(-3.54760150451765,2.24156301194163,4.38891031245443));
#15499=CARTESIAN_POINT('Ctrl Pts',(-3.59995964312543,2.22424755626985,4.38520571610216));
#15500=CARTESIAN_POINT('Ctrl Pts',(-3.66175114033895,2.23545374197608,4.3815011197499));
#15501=CARTESIAN_POINT('Ctrl Pts',(-3.70469438806425,2.2700507456572,4.37779652339763));
#15502=CARTESIAN_POINT('Ctrl Pts',(-3.74311977927038,2.30100796178371,4.37448167015208));
#15503=CARTESIAN_POINT('Ctrl Pts',(-3.76645417654063,2.35069321376496,4.37116681690653));
#15504=CARTESIAN_POINT('Ctrl Pts',(-3.76680083090633,2.40009693666208,4.36785196366098));
#15505=CARTESIAN_POINT('Ctrl Pts',(-3.76675586981256,2.39987855699196,4.38714803633902));
#15506=CARTESIAN_POINT('Ctrl Pts',(-3.76681887033176,2.39219581029783,4.38766315717711));
#15507=CARTESIAN_POINT('Ctrl Pts',(-3.76633386046459,2.38452105604489,4.3881782780152));
#15508=CARTESIAN_POINT('Ctrl Pts',(-3.76527361543791,2.37692660254772,4.38869339885329));
#15509=CARTESIAN_POINT('Ctrl Pts',(-3.75764864753156,2.32230954448549,4.39239799520556));
#15510=CARTESIAN_POINT('Ctrl Pts',(-3.72027217218665,2.27184568967097,4.39610259155783));
#15511=CARTESIAN_POINT('Ctrl Pts',(-3.67024982973388,2.2486305064859,4.3998071879101));
#15512=CARTESIAN_POINT('Ctrl Pts',(-3.62022748728111,2.22541532330082,4.40351178426237));
#15513=CARTESIAN_POINT('Ctrl Pts',(-3.55755927772049,2.22944881174518,4.40721638061463));
#15514=CARTESIAN_POINT('Ctrl Pts',(-3.51092562033288,2.25888482364762,4.4109209769669));
#15515=CARTESIAN_POINT('Ctrl Pts',(-3.46429196294527,2.28832083555005,4.41462557331917));
#15516=CARTESIAN_POINT('Ctrl Pts',(-3.43369285773067,2.34315937091056,4.41833016967144));
#15517=CARTESIAN_POINT('Ctrl Pts',(-3.43313217976425,2.39830336261017,4.42203476602371));
#15518=CARTESIAN_POINT('Ctrl Pts',(-3.43257150179783,2.45344735430978,4.42573936237597));
#15519=CARTESIAN_POINT('Ctrl Pts',(-3.46204925107959,2.5088968023485,4.42944395872824));
#15520=CARTESIAN_POINT('Ctrl Pts',(-3.5080747579799,2.53927490269551,4.43314855508051));
#15521=CARTESIAN_POINT('Ctrl Pts',(-3.55410026488021,2.56965300304252,4.43685315143278));
#15522=CARTESIAN_POINT('Ctrl Pts',(-3.61667352939907,2.57495975569782,4.44055774778505));
#15523=CARTESIAN_POINT('Ctrl Pts',(-3.66715754746926,2.55276652004746,4.44426234413731));
#15524=CARTESIAN_POINT('Ctrl Pts',(-3.71764156553946,2.53057328439709,4.44796694048958));
#15525=CARTESIAN_POINT('Ctrl Pts',(-3.756036337161,2.48088006044104,4.45167153684185));
#15526=CARTESIAN_POINT('Ctrl Pts',(-3.76477027476388,2.4264292215015,4.45537613319412));
#15527=CARTESIAN_POINT('Ctrl Pts',(-3.7661627513915,2.41774796866627,4.45596676757575));
#15528=CARTESIAN_POINT('Ctrl Pts',(-3.76680128414385,2.40894578279607,4.45655740195739));
#15529=CARTESIAN_POINT('Ctrl Pts',(-3.76672468602162,2.4001324774977,4.45714803633902));
#15530=CARTESIAN_POINT('Origin',(-3.6,2.4,4.7));
#15531=CARTESIAN_POINT('',(-3.76633791206845,2.40003802478337,4.52714803633902));
#15532=CARTESIAN_POINT('',(-3.76649857382306,2.39985687062932,4.50785196366098));
#15533=CARTESIAN_POINT('',(-3.7666,2.4,4.7));
#15534=CARTESIAN_POINT('Ctrl Pts',(-3.76649857382306,2.39985687062932,4.50785196366098));
#15535=CARTESIAN_POINT('Ctrl Pts',(-3.76617945752874,2.43880728528579,4.50525071011481));
#15536=CARTESIAN_POINT('Ctrl Pts',(-3.75254366540545,2.47795898788161,4.50264945656864));
#15537=CARTESIAN_POINT('Ctrl Pts',(-3.72758425733276,2.50756395676541,4.50004820302248));
#15538=CARTESIAN_POINT('Ctrl Pts',(-3.6920381137294,2.54972611350612,4.49634360667021));
#15539=CARTESIAN_POINT('Ctrl Pts',(-3.63352511396685,2.57252533344874,4.49263901031794));
#15540=CARTESIAN_POINT('Ctrl Pts',(-3.57882406188105,2.56552742213501,4.48893441396567));
#15541=CARTESIAN_POINT('Ctrl Pts',(-3.52412300979526,2.55852951082128,4.4852298176134));
#15542=CARTESIAN_POINT('Ctrl Pts',(-3.47323390538621,2.52173446825121,4.48152522126114));
#15543=CARTESIAN_POINT('Ctrl Pts',(-3.44944644044618,2.47198175864633,4.47782062490887));
#15544=CARTESIAN_POINT('Ctrl Pts',(-3.42565897550616,2.42222904904145,4.4741160285566));
#15545=CARTESIAN_POINT('Ctrl Pts',(-3.42897315003517,2.35951867240177,4.47041143220433));
#15546=CARTESIAN_POINT('Ctrl Pts',(-3.45787220405951,2.31255037948392,4.46670683585206));
#15547=CARTESIAN_POINT('Ctrl Pts',(-3.48677125808385,2.26558208656607,4.46300223949979));
#15548=CARTESIAN_POINT('Ctrl Pts',(-3.54125519160353,2.23435587737005,4.45929764314752));
#15549=CARTESIAN_POINT('Ctrl Pts',(-3.59638914193523,2.23316262102818,4.45559304679526));
#15550=CARTESIAN_POINT('Ctrl Pts',(-3.65152309226694,2.23196936468632,4.45188845044299));
#15551=CARTESIAN_POINT('Ctrl Pts',(-3.70730705941068,2.26080906119861,4.44818385409072));
#15552=CARTESIAN_POINT('Ctrl Pts',(-3.73821115757027,2.30648302502563,4.44447925773845));
#15553=CARTESIAN_POINT('Ctrl Pts',(-3.75663966522468,2.33371899184293,4.44227015971263));
#15554=CARTESIAN_POINT('Ctrl Pts',(-3.76622116784026,2.36694103711801,4.4400610616868));
#15555=CARTESIAN_POINT('Ctrl Pts',(-3.7663710759754,2.40008323252274,4.43785196366098));
#15556=CARTESIAN_POINT('Ctrl Pts',(-3.76672468602162,2.4001324774977,4.45714803633902));
#15557=CARTESIAN_POINT('Ctrl Pts',(-3.76632084288778,2.35366668006347,4.46026199830966));
#15558=CARTESIAN_POINT('Ctrl Pts',(-3.74603890809821,2.30689180212375,4.46337596028029));
#15559=CARTESIAN_POINT('Ctrl Pts',(-3.71156689963546,2.27590095059859,4.46648992225092));
#15560=CARTESIAN_POINT('Ctrl Pts',(-3.67055648331992,2.23903197255825,4.47019451860319));
#15561=CARTESIAN_POINT('Ctrl Pts',(-3.60946254710462,2.2245024704006,4.47389911495546));
#15562=CARTESIAN_POINT('Ctrl Pts',(-3.55624507667009,2.23896195008268,4.47760371130773));
#15563=CARTESIAN_POINT('Ctrl Pts',(-3.50302760623556,2.25342142976477,4.48130830766));
#15564=CARTESIAN_POINT('Ctrl Pts',(-3.45768660158179,2.29686989128659,4.48501290401227));
#15565=CARTESIAN_POINT('Ctrl Pts',(-3.4409726309165,2.34942290140806,4.48871750036453));
#15566=CARTESIAN_POINT('Ctrl Pts',(-3.4242586602512,2.40197591152952,4.4924220967168));
#15567=CARTESIAN_POINT('Ctrl Pts',(-3.43617172357437,2.46363347025063,4.49612669306907));
#15568=CARTESIAN_POINT('Ctrl Pts',(-3.47125973974121,2.50617764542895,4.49983128942133));
#15569=CARTESIAN_POINT('Ctrl Pts',(-3.50634775590806,2.54872182060726,4.5035358857736));
#15570=CARTESIAN_POINT('Ctrl Pts',(-3.56461072491859,2.57215261224279,4.50724048212587));
#15571=CARTESIAN_POINT('Ctrl Pts',(-3.61938426871317,2.56574678606726,4.51094507847814));
#15572=CARTESIAN_POINT('Ctrl Pts',(-3.67415781250775,2.55934095989172,4.51464967483041));
#15573=CARTESIAN_POINT('Ctrl Pts',(-3.72544193108638,2.52309851590513,4.51835427118267));
#15574=CARTESIAN_POINT('Ctrl Pts',(-3.7497661567401,2.47360601391412,4.52205886753494));
#15575=CARTESIAN_POINT('Ctrl Pts',(-3.7609045803459,2.45094266337894,4.5237552571363));
#15576=CARTESIAN_POINT('Ctrl Pts',(-3.76638989212213,2.42550096131782,4.52545164673766));
#15577=CARTESIAN_POINT('Ctrl Pts',(-3.76633791206845,2.40003802478337,4.52714803633902));
#15578=CARTESIAN_POINT('Origin',(-3.6,2.4,4.7));
#15579=CARTESIAN_POINT('',(-3.76658523827666,2.39984765670423,4.59714803633902));
#15580=CARTESIAN_POINT('',(-3.76687644222506,2.40000067112036,4.57785196366098));
#15581=CARTESIAN_POINT('',(-3.7666,2.4,4.7));
#15582=CARTESIAN_POINT('Ctrl Pts',(-3.76687644086079,2.40000067111705,4.57785196366098));
#15583=CARTESIAN_POINT('Ctrl Pts',(-3.76687973678962,2.45518344204594,4.57414495489509));
#15584=CARTESIAN_POINT('Ctrl Pts',(-3.73679497953693,2.51036312381259,4.57043794612919));
#15585=CARTESIAN_POINT('Ctrl Pts',(-3.69041339694851,2.54026106127768,4.5667309373633));
#15586=CARTESIAN_POINT('Ctrl Pts',(-3.64406199814677,2.57013954203352,4.56302634101103));
#15587=CARTESIAN_POINT('Ctrl Pts',(-3.58143498975323,2.57476917303812,4.55932174465876));
#15588=CARTESIAN_POINT('Ctrl Pts',(-3.53119397724287,2.55203117737673,4.55561714830649));
#15589=CARTESIAN_POINT('Ctrl Pts',(-3.4809529647325,2.52929318171533,4.55191255195423));
#15590=CARTESIAN_POINT('Ctrl Pts',(-3.44309794810529,2.47918755938795,4.54820795560196));
#15591=CARTESIAN_POINT('Ctrl Pts',(-3.43495349044459,2.42464543263837,4.54450335924969));
#15592=CARTESIAN_POINT('Ctrl Pts',(-3.42680903278389,2.37010330588879,4.54079876289742));
#15593=CARTESIAN_POINT('Ctrl Pts',(-3.44837513408969,2.31112467471701,4.53709416654516));
#15594=CARTESIAN_POINT('Ctrl Pts',(-3.48978194566841,2.27470144397531,4.53338957019289));
#15595=CARTESIAN_POINT('Ctrl Pts',(-3.53118875724712,2.23827821323361,4.52968497384062));
#15596=CARTESIAN_POINT('Ctrl Pts',(-3.59243627909875,2.22441038292198,4.52598037748835));
#15597=CARTESIAN_POINT('Ctrl Pts',(-3.64549423583691,2.23944464448895,4.52227578113608));
#15598=CARTESIAN_POINT('Ctrl Pts',(-3.69855219257508,2.25447890605592,4.51857118478381));
#15599=CARTESIAN_POINT('Ctrl Pts',(-3.74342058419978,2.29841525950148,4.51486658843154));
#15600=CARTESIAN_POINT('Ctrl Pts',(-3.75956513629004,2.35114598299368,4.51116199207928));
#15601=CARTESIAN_POINT('Ctrl Pts',(-3.76437348076611,2.36685081528665,4.51005864927318));
#15602=CARTESIAN_POINT('Ctrl Pts',(-3.76663392958958,2.3833357360905,4.50895530646708));
#15603=CARTESIAN_POINT('Ctrl Pts',(-3.76649857382306,2.39985687062932,4.50785196366098));
#15604=CARTESIAN_POINT('Ctrl Pts',(-3.76633791206845,2.40003802478337,4.52714803633902));
#15605=CARTESIAN_POINT('Ctrl Pts',(-3.76627637744537,2.36989468919261,4.52915624308993));
#15606=CARTESIAN_POINT('Ctrl Pts',(-3.758454818996,2.33972159536913,4.53116444984084));
#15607=CARTESIAN_POINT('Ctrl Pts',(-3.74306538301875,2.31409282238037,4.53317265659175));
#15608=CARTESIAN_POINT('Ctrl Pts',(-3.71467605091489,2.26681469283306,4.53687725294402));
#15609=CARTESIAN_POINT('Ctrl Pts',(-3.66053305397837,2.23500099373388,4.54058184929628));
#15610=CARTESIAN_POINT('Ctrl Pts',(-3.6054152417587,2.23321144482349,4.54428644564855));
#15611=CARTESIAN_POINT('Ctrl Pts',(-3.55029742953903,2.23142189591311,4.54799104200082));
#15612=CARTESIAN_POINT('Ctrl Pts',(-3.49420480203621,2.25965649719153,4.55169563835309));
#15613=CARTESIAN_POINT('Ctrl Pts',(-3.46280846829882,2.30499352330658,4.55540023470536));
#15614=CARTESIAN_POINT('Ctrl Pts',(-3.43141213456143,2.35033054942163,4.55910483105762));
#15615=CARTESIAN_POINT('Ctrl Pts',(-3.42471209458945,2.41277000037331,4.56280942740989));
#15616=CARTESIAN_POINT('Ctrl Pts',(-3.44577465966535,2.46373610736585,4.56651402376216));
#15617=CARTESIAN_POINT('Ctrl Pts',(-3.46683722474125,2.51470221435838,4.57021862011443));
#15618=CARTESIAN_POINT('Ctrl Pts',(-3.51566239486502,2.55419497739177,4.5739232164667));
#15619=CARTESIAN_POINT('Ctrl Pts',(-3.56990505407324,2.56414030953056,4.57762781281897));
#15620=CARTESIAN_POINT('Ctrl Pts',(-3.62414771328146,2.57408564166935,4.58133240917123));
#15621=CARTESIAN_POINT('Ctrl Pts',(-3.68380786157412,2.55448354291355,4.5850370055235));
#15622=CARTESIAN_POINT('Ctrl Pts',(-3.72158169378842,2.51430502490722,4.58874160187577));
#15623=CARTESIAN_POINT('Ctrl Pts',(-3.75015369954742,2.4839141225134,4.59154374669685));
#15624=CARTESIAN_POINT('Ctrl Pts',(-3.76620375341029,2.44175070750818,4.59434589151794));
#15625=CARTESIAN_POINT('Ctrl Pts',(-3.76658523827666,2.39984765670423,4.59714803633902));
#15626=CARTESIAN_POINT('Origin',(-3.6,2.4,4.7));
#15627=CARTESIAN_POINT('',(-3.76685426518066,2.40005503529171,4.66714803633902));
#15628=CARTESIAN_POINT('',(-3.76649661588353,2.40014270746765,4.64785196366098));
#15629=CARTESIAN_POINT('',(-3.7666,2.4,4.7));
#15630=CARTESIAN_POINT('Ctrl Pts',(-3.76649661588353,2.40014270746765,4.64785196366098));
#15631=CARTESIAN_POINT('Ctrl Pts',(-3.76663204639349,2.41673658143502,4.64674379602763));
#15632=CARTESIAN_POINT('Ctrl Pts',(-3.76435138934107,2.43329406659146,4.64563562839428));
#15633=CARTESIAN_POINT('Ctrl Pts',(-3.75950152904524,2.44906128711078,4.64452746076093));
#15634=CARTESIAN_POINT('Ctrl Pts',(-3.74328848128947,2.50177099082653,4.64082286440866));
#15635=CARTESIAN_POINT('Ctrl Pts',(-3.69836304459695,2.54564901270383,4.63711826805639));
#15636=CARTESIAN_POINT('Ctrl Pts',(-3.64528559981485,2.5606143272255,4.63341367170412));
#15637=CARTESIAN_POINT('Ctrl Pts',(-3.59220815503275,2.57557964174716,4.62970907535186));
#15638=CARTESIAN_POINT('Ctrl Pts',(-3.53097870216106,2.56163224891319,4.62600447899959));
#15639=CARTESIAN_POINT('Ctrl Pts',(-3.48961924750057,2.52515525214062,4.62229988264732));
#15640=CARTESIAN_POINT('Ctrl Pts',(-3.44825979284008,2.48867825536805,4.61859528629505));
#15641=CARTESIAN_POINT('Ctrl Pts',(-3.4267703363908,2.42967165465689,4.61489068994278));
#15642=CARTESIAN_POINT('Ctrl Pts',(-3.43498564975134,2.37514015541382,4.61118609359051));
#15643=CARTESIAN_POINT('Ctrl Pts',(-3.44320096311188,2.32060865617075,4.60748149723825));
#15644=CARTESIAN_POINT('Ctrl Pts',(-3.48112104628225,2.27055225839578,4.60377690088598));
#15645=CARTESIAN_POINT('Ctrl Pts',(-3.53139155817582,2.2478795563676,4.60007230453371));
#15646=CARTESIAN_POINT('Ctrl Pts',(-3.58166207006939,2.22520685433943,4.59636770818145));
#15647=CARTESIAN_POINT('Ctrl Pts',(-3.64428301068616,2.22991784805805,4.59266311182918));
#15648=CARTESIAN_POINT('Ctrl Pts',(-3.69059555147242,2.25985652453919,4.58895851547691));
#15649=CARTESIAN_POINT('Ctrl Pts',(-3.73687793377613,2.28977570511195,4.58525633153827));
#15650=CARTESIAN_POINT('Ctrl Pts',(-3.76687314922176,2.34488972287695,4.58155414759963));
#15651=CARTESIAN_POINT('Ctrl Pts',(-3.76687644086079,2.40000067111705,4.57785196366098));
#15652=CARTESIAN_POINT('Ctrl Pts',(-3.76658523827666,2.39984765670423,4.59714803633902));
#15653=CARTESIAN_POINT('Ctrl Pts',(-3.76670809830844,2.38635246827757,4.5980504878702));
#15654=CARTESIAN_POINT('Ctrl Pts',(-3.76520579898216,2.37288428508147,4.59895293940139));
#15655=CARTESIAN_POINT('Ctrl Pts',(-3.76197323034856,2.35984505467766,4.59985539093257));
#15656=CARTESIAN_POINT('Ctrl Pts',(-3.74870341855848,2.30631853971129,4.60355998728484));
#15657=CARTESIAN_POINT('Ctrl Pts',(-3.70627627884239,2.26002044703541,4.60726458363711));
#15658=CARTESIAN_POINT('Ctrl Pts',(-3.65410883226945,2.24213936129044,4.61096917998938));
#15659=CARTESIAN_POINT('Ctrl Pts',(-3.60194138569651,2.22425827554546,4.61467377634165));
#15660=CARTESIAN_POINT('Ctrl Pts',(-3.54003363226672,2.23479419673139,4.61837837269391));
#15661=CARTESIAN_POINT('Ctrl Pts',(-3.49671800637814,2.26892530077511,4.62208296904618));
#15662=CARTESIAN_POINT('Ctrl Pts',(-3.45340238048956,2.30305640481884,4.62578756539845));
#15663=CARTESIAN_POINT('Ctrl Pts',(-3.42867888214219,2.36078269172036,4.62949216175072));
#15664=CARTESIAN_POINT('Ctrl Pts',(-3.43386236054643,2.4156853989487,4.63319675810298));
#15665=CARTESIAN_POINT('Ctrl Pts',(-3.43904583895067,2.47058810617705,4.63690135445525));
#15666=CARTESIAN_POINT('Ctrl Pts',(-3.47413629410653,2.52266723373221,4.64060595080752));
#15667=CARTESIAN_POINT('Ctrl Pts',(-3.52307438023553,2.54808847357993,4.64431054715979));
#15668=CARTESIAN_POINT('Ctrl Pts',(-3.57201246636453,2.57350971342765,4.64801514351206));
#15669=CARTESIAN_POINT('Ctrl Pts',(-3.63479818346667,2.57227306556792,4.65171973986433));
#15670=CARTESIAN_POINT('Ctrl Pts',(-3.68269729209092,2.54494448890598,4.65542433621659));
#15671=CARTESIAN_POINT('Ctrl Pts',(-3.73059640071517,2.51761591224403,4.65912893256886));
#15672=CARTESIAN_POINT('Ctrl Pts',(-3.76360890086153,2.46419540677987,4.66283352892113));
#15673=CARTESIAN_POINT('Ctrl Pts',(-3.76662643464441,2.40913116975406,4.6665381252734));
#15674=CARTESIAN_POINT('Ctrl Pts',(-3.76679203318471,2.406109312194,4.66674142896194));
#15675=CARTESIAN_POINT('Ctrl Pts',(-3.76686729650514,2.4030825042416,4.66694473265048));
#15676=CARTESIAN_POINT('Ctrl Pts',(-3.76685426518066,2.40005503529171,4.66714803633902));
#15677=CARTESIAN_POINT('Origin',(-3.6,2.4,4.7));
#15678=CARTESIAN_POINT('',(-3.76642275699063,2.40011764661364,4.73714803633902));
#15679=CARTESIAN_POINT('',(-3.76637219462709,2.39991574862477,4.71785196366098));
#15680=CARTESIAN_POINT('',(-3.7666,2.4,4.7));
#15681=CARTESIAN_POINT('Ctrl Pts',(-3.76637219462709,2.39991574862477,4.71785196366098));
#15682=CARTESIAN_POINT('Ctrl Pts',(-3.76622008929152,2.43312978877493,4.7156380408079));
#15683=CARTESIAN_POINT('Ctrl Pts',(-3.75659374130514,2.46642503349729,4.71342411795483));
#15684=CARTESIAN_POINT('Ctrl Pts',(-3.73808953093009,2.49369647329664,4.71121019510175));
#15685=CARTESIAN_POINT('Ctrl Pts',(-3.70712610771876,2.53933025690454,4.70750559874949));
#15686=CARTESIAN_POINT('Ctrl Pts',(-3.65130473898255,2.56809743365675,4.70380100239722));
#15687=CARTESIAN_POINT('Ctrl Pts',(-3.59617239065227,2.56683254199167,4.70009640604495));
#15688=CARTESIAN_POINT('Ctrl Pts',(-3.541040042322,2.56556765032658,4.69639180969268));
#15689=CARTESIAN_POINT('Ctrl Pts',(-3.48659671439765,2.53427069024418,4.69268721334041));
#15690=CARTESIAN_POINT('Ctrl Pts',(-3.45775870461848,2.48726489299201,4.68898261698815));
#15691=CARTESIAN_POINT('Ctrl Pts',(-3.4289206948393,2.44025909573984,4.68527802063588));
#15692=CARTESIAN_POINT('Ctrl Pts',(-3.4256880032053,2.3775444613179,4.68157342428361));
#15693=CARTESIAN_POINT('Ctrl Pts',(-3.44954008937339,2.32782269778556,4.67786882793134));
#15694=CARTESIAN_POINT('Ctrl Pts',(-3.47339217554148,2.27810093425323,4.67416423157907));
#15695=CARTESIAN_POINT('Ctrl Pts',(-3.52432903951166,2.2413720416105,4.67045963522681));
#15696=CARTESIAN_POINT('Ctrl Pts',(-3.57903913665629,2.23444520584228,4.66675503887454));
#15697=CARTESIAN_POINT('Ctrl Pts',(-3.63374923380092,2.22751837007406,4.66305044252227));
#15698=CARTESIAN_POINT('Ctrl Pts',(-3.69223256411999,2.25039359118035,4.65934584617));
#15699=CARTESIAN_POINT('Ctrl Pts',(-3.72772389987002,2.29260189451059,4.65564124981773));
#15700=CARTESIAN_POINT('Ctrl Pts',(-3.75259860001318,2.32218429445987,4.65304482109882));
#15701=CARTESIAN_POINT('Ctrl Pts',(-3.766179303182,2.36126338124449,4.6504483923799));
#15702=CARTESIAN_POINT('Ctrl Pts',(-3.76649661588353,2.40014270746765,4.64785196366098));
#15703=CARTESIAN_POINT('Ctrl Pts',(-3.76685426518066,2.40005503529171,4.66714803633902));
#15704=CARTESIAN_POINT('Ctrl Pts',(-3.76662983993221,2.34791601656576,4.67064932900275));
#15705=CARTESIAN_POINT('Ctrl Pts',(-3.7402175145738,2.29558094816933,4.67415062166648));
#15706=CARTESIAN_POINT('Ctrl Pts',(-3.69804051189557,2.26495998737175,4.6776519143302));
#15707=CARTESIAN_POINT('Ctrl Pts',(-3.65341448794446,2.23256101060272,4.68135651068247));
#15708=CARTESIAN_POINT('Ctrl Pts',(-3.59113987262282,2.22447102565214,4.68506110703474));
#15709=CARTESIAN_POINT('Ctrl Pts',(-3.53971699675369,2.24439246000598,4.68876570338701));
#15710=CARTESIAN_POINT('Ctrl Pts',(-3.48829412088457,2.26431389435981,4.69247029973927));
#15711=CARTESIAN_POINT('Ctrl Pts',(-3.44772298446796,2.31224674801807,4.69617489609154));
#15712=CARTESIAN_POINT('Ctrl Pts',(-3.43657119813891,2.36625427870627,4.69987949244381));
#15713=CARTESIAN_POINT('Ctrl Pts',(-3.42541941180987,2.42026180939447,4.70358408879608));
#15714=CARTESIAN_POINT('Ctrl Pts',(-3.44368697556839,2.48034401711262,4.70728868514835));
#15715=CARTESIAN_POINT('Ctrl Pts',(-3.48301363527625,2.51900393880922,4.71099328150062));
#15716=CARTESIAN_POINT('Ctrl Pts',(-3.52234029498412,2.55766386050582,4.71469787785288));
#15717=CARTESIAN_POINT('Ctrl Pts',(-3.58272605064134,2.57490149618086,4.71840247420515));
#15718=CARTESIAN_POINT('Ctrl Pts',(-3.63653501876085,2.56282794412363,4.72210707055742));
#15719=CARTESIAN_POINT('Ctrl Pts',(-3.69034398688037,2.5507543920664,4.72581166690969));
#15720=CARTESIAN_POINT('Ctrl Pts',(-3.73757616746218,2.50936965227689,4.72951626326196));
#15721=CARTESIAN_POINT('Ctrl Pts',(-3.75661548523835,2.45761368558721,4.73322085961422));
#15722=CARTESIAN_POINT('Ctrl Pts',(-3.76334323265594,2.43932515890074,4.73452991852249));
#15723=CARTESIAN_POINT('Ctrl Pts',(-3.76655071173719,2.4197416412828,4.73583897743076));
#15724=CARTESIAN_POINT('Ctrl Pts',(-3.76642275699063,2.40011764661364,4.73714803633902));
#15725=CARTESIAN_POINT('Origin',(-3.6,2.4,4.7));
#15726=CARTESIAN_POINT('',(-3.76642910764821,2.39987935508533,4.80714803633902));
#15727=CARTESIAN_POINT('',(-3.76680408556428,2.39990252619421,4.78785196366098));
#15728=CARTESIAN_POINT('',(-3.7666,2.4,4.7));
#15729=CARTESIAN_POINT('Ctrl Pts',(-3.76680408556428,2.39990252619421,4.78785196366098));
#15730=CARTESIAN_POINT('Ctrl Pts',(-3.76646018913848,2.44937641051311,4.78453228558818));
#15731=CARTESIAN_POINT('Ctrl Pts',(-3.74304696564969,2.49913297683607,4.78121260751538));
#15732=CARTESIAN_POINT('Ctrl Pts',(-3.70452480260444,2.53008579208055,4.77789292944258));
#15733=CARTESIAN_POINT('Ctrl Pts',(-3.66153597610701,2.56462760123568,4.77418833309031));
#15734=CARTESIAN_POINT('Ctrl Pts',(-3.59973129998187,2.5757522439241,4.77048373673804));
#15735=CARTESIAN_POINT('Ctrl Pts',(-3.54739603471406,2.55836846433844,4.76677914038578));
#15736=CARTESIAN_POINT('Ctrl Pts',(-3.49506076944624,2.54098468475278,4.76307454403351));
#15737=CARTESIAN_POINT('Ctrl Pts',(-3.45219491503573,2.49509248289304,4.75936994768124));
#15738=CARTESIAN_POINT('Ctrl Pts',(-3.43841627281944,2.44169468516681,4.75566535132897));
#15739=CARTESIAN_POINT('Ctrl Pts',(-3.42463763060315,2.38829688744059,4.7519607549767));
#15740=CARTESIAN_POINT('Ctrl Pts',(-3.43994620058106,2.32739349384788,4.74825615862443));
#15741=CARTESIAN_POINT('Ctrl Pts',(-3.4773359288973,2.28685728781211,4.74455156227217));
#15742=CARTESIAN_POINT('Ctrl Pts',(-3.51472565721353,2.24632108177635,4.7408469659199));
#15743=CARTESIAN_POINT('Ctrl Pts',(-3.57419654386808,2.22615206329753,4.73714236956763));
#15744=CARTESIAN_POINT('Ctrl Pts',(-3.62853140036063,2.23558069804861,4.73343777321536));
#15745=CARTESIAN_POINT('Ctrl Pts',(-3.68286625685319,2.24500933279969,4.7297331768631));
#15746=CARTESIAN_POINT('Ctrl Pts',(-3.73206508318374,2.28403562078066,4.72602858051083));
#15747=CARTESIAN_POINT('Ctrl Pts',(-3.7536117575058,2.33479896000292,4.72232398415856));
#15748=CARTESIAN_POINT('Ctrl Pts',(-3.76228181312143,2.35522535934946,4.72083331065937));
#15749=CARTESIAN_POINT('Ctrl Pts',(-3.76647460984564,2.37755214666628,4.71934263716017));
#15750=CARTESIAN_POINT('Ctrl Pts',(-3.76637219462709,2.39991574862477,4.71785196366098));
#15751=CARTESIAN_POINT('Ctrl Pts',(-3.76642275699063,2.40011764661364,4.73714803633902));
#15752=CARTESIAN_POINT('Ctrl Pts',(-3.76618860374924,2.36420634137441,4.73954357378302));
#15753=CARTESIAN_POINT('Ctrl Pts',(-3.75478479252022,2.32815948710566,4.74193911122702));
#15754=CARTESIAN_POINT('Ctrl Pts',(-3.73334402193678,2.29966496724918,4.74433464867103));
#15755=CARTESIAN_POINT('Ctrl Pts',(-3.70018678588852,2.25559940919069,4.74803924502329));
#15756=CARTESIAN_POINT('Ctrl Pts',(-3.64302585882149,2.22959548666357,4.75174384137557));
#15757=CARTESIAN_POINT('Ctrl Pts',(-3.58802126313241,2.23355404226464,4.75544843772783));
#15758=CARTESIAN_POINT('Ctrl Pts',(-3.53301666744333,2.2375125978657,4.7591530340801));
#15759=CARTESIAN_POINT('Ctrl Pts',(-3.48016840313221,2.27143363159494,4.76285763043237));
#15760=CARTESIAN_POINT('Ctrl Pts',(-3.45366277803107,2.31979299002082,4.76656222678463));
#15761=CARTESIAN_POINT('Ctrl Pts',(-3.42715715292992,2.36815234844671,4.7702668231369));
#15762=CARTESIAN_POINT('Ctrl Pts',(-3.42699416703876,2.43095003156924,4.77397141948917));
#15763=CARTESIAN_POINT('Ctrl Pts',(-3.45324841177486,2.47944632362031,4.77767601584144));
#15764=CARTESIAN_POINT('Ctrl Pts',(-3.47950265651095,2.52794261567138,4.78138061219371));
#15765=CARTESIAN_POINT('Ctrl Pts',(-3.53217413187432,2.56213751665099,4.78508520854598));
#15766=CARTESIAN_POINT('Ctrl Pts',(-3.58715743849732,2.56638153622754,4.78878980489824));
#15767=CARTESIAN_POINT('Ctrl Pts',(-3.64214074512033,2.57062555580409,4.79249440125051));
#15768=CARTESIAN_POINT('Ctrl Pts',(-3.69943588300298,2.54491869397758,4.79619899760278));
#15769=CARTESIAN_POINT('Ctrl Pts',(-3.73282140740775,2.50102584183074,4.79990359395505));
#15770=CARTESIAN_POINT('Ctrl Pts',(-3.754583518131,2.4724146061108,4.80231840808304));
#15771=CARTESIAN_POINT('Ctrl Pts',(-3.76618645992471,2.43607616275589,4.80473322221103));
#15772=CARTESIAN_POINT('Ctrl Pts',(-3.76642910764821,2.39987935508533,4.80714803633902));
#15773=CARTESIAN_POINT('Origin',(-3.6,2.4,4.7));
#15774=CARTESIAN_POINT('',(-3.76685809662611,2.39994994258553,4.87714803633902));
#15775=CARTESIAN_POINT('',(-3.7666675037778,2.40014587506062,4.85785196366098));
#15776=CARTESIAN_POINT('',(-3.7666,2.4,4.7));
#15777=CARTESIAN_POINT('Ctrl Pts',(-3.7666675037778,2.40014587506062,4.85785196366098));
#15778=CARTESIAN_POINT('Ctrl Pts',(-3.76676616841865,2.41091157707528,4.85713112672072));
#15779=CARTESIAN_POINT('Ctrl Pts',(-3.76581236284584,2.4216598706667,4.85641028978047));
#15780=CARTESIAN_POINT('Ctrl Pts',(-3.76374257225157,2.43218878210118,4.85568945284021));
#15781=CARTESIAN_POINT('Ctrl Pts',(-3.7531053001346,2.48630000298229,4.85198485648794));
#15782=CARTESIAN_POINT('Ctrl Pts',(-3.71299219510172,2.53461681652064,4.84828026013567));
#15783=CARTESIAN_POINT('Ctrl Pts',(-3.66176124712798,2.5550267590254,4.8445756637834));
#15784=CARTESIAN_POINT('Ctrl Pts',(-3.61053029915424,2.57543670153016,4.84087106743113));
#15785=CARTESIAN_POINT('Ctrl Pts',(-3.54818150823965,2.56793977300133,4.83716647107887));
#15786=CARTESIAN_POINT('Ctrl Pts',(-3.50324915208796,2.53596698529063,4.8334618747266));
#15787=CARTESIAN_POINT('Ctrl Pts',(-3.45831679593627,2.50399419757992,4.82975727837433));
#15788=CARTESIAN_POINT('Ctrl Pts',(-3.43080087454749,2.44754555068734,4.82605268202206));
#15789=CARTESIAN_POINT('Ctrl Pts',(-3.43329420537107,2.39245508794886,4.8223480856698));
#15790=CARTESIAN_POINT('Ctrl Pts',(-3.43578753619466,2.33736462521039,4.81864348931753));
#15791=CARTESIAN_POINT('Ctrl Pts',(-3.46829011923061,2.28363234662601,4.81493889296526));
#15792=CARTESIAN_POINT('Ctrl Pts',(-3.51592696305034,2.25584913417262,4.81123429661299));
#15793=CARTESIAN_POINT('Ctrl Pts',(-3.56356380687008,2.22806592171924,4.80752970026072));
#15794=CARTESIAN_POINT('Ctrl Pts',(-3.62633491147359,2.22623177539684,4.80382510390846));
#15795=CARTESIAN_POINT('Ctrl Pts',(-3.67551272490272,2.25118610267019,4.80012050755619));
#15796=CARTESIAN_POINT('Ctrl Pts',(-3.72469053833185,2.27614042994354,4.79641591120392));
#15797=CARTESIAN_POINT('Ctrl Pts',(-3.76027506058658,2.32788323081264,4.79271131485165));
#15798=CARTESIAN_POINT('Ctrl Pts',(-3.76598083327909,2.38273411905811,4.78900671849938));
#15799=CARTESIAN_POINT('Ctrl Pts',(-3.76657367957029,2.38843328504628,4.78862180021992));
#15800=CARTESIAN_POINT('Ctrl Pts',(-3.76684396052131,2.39416600535905,4.78823688194045));
#15801=CARTESIAN_POINT('Ctrl Pts',(-3.76680408556428,2.39990252619421,4.78785196366098));
#15802=CARTESIAN_POINT('Ctrl Pts',(-3.76642910764821,2.39987935508533,4.80714803633902));
#15803=CARTESIAN_POINT('Ctrl Pts',(-3.76655870881167,2.38054619044631,4.8084378185633));
#15804=CARTESIAN_POINT('Ctrl Pts',(-3.76344748981416,2.36125343108011,4.80972760078758));
#15805=CARTESIAN_POINT('Ctrl Pts',(-3.75691243582065,2.3432000486953,4.81101738301185));
#15806=CARTESIAN_POINT('Ctrl Pts',(-3.73814202890189,2.29134595017387,4.81472197936412));
#15807=CARTESIAN_POINT('Ctrl Pts',(-3.6911253041375,2.24971659559817,4.81842657571639));
#15808=CARTESIAN_POINT('Ctrl Pts',(-3.63737973221885,2.2373638951443,4.82213117206866));
#15809=CARTESIAN_POINT('Ctrl Pts',(-3.58363416030021,2.22501119469043,4.82583576842093));
#15810=CARTESIAN_POINT('Ctrl Pts',(-3.52315974122731,2.24193514835838,4.82954036477319));
#15811=CARTESIAN_POINT('Ctrl Pts',(-3.48363293580215,2.28039041278662,4.83324496112546));
#15812=CARTESIAN_POINT('Ctrl Pts',(-3.44410613037699,2.31884567721486,4.83694955747773));
#15813=CARTESIAN_POINT('Ctrl Pts',(-3.42552693859956,2.3788322524034,4.84065415383));
#15814=CARTESIAN_POINT('Ctrl Pts',(-3.436398232938,2.43289694207027,4.84435875018227));
#15815=CARTESIAN_POINT('Ctrl Pts',(-3.44726952727644,2.48696163173715,4.84806334653453));
#15816=CARTESIAN_POINT('Ctrl Pts',(-3.48759130773074,2.53510443588236,4.8517679428868));
#15817=CARTESIAN_POINT('Ctrl Pts',(-3.53891008283594,2.5552925272004,4.85547253923907));
#15818=CARTESIAN_POINT('Ctrl Pts',(-3.59022885794113,2.57548061851844,4.85917713559134));
#15819=CARTESIAN_POINT('Ctrl Pts',(-3.65254462769722,2.56771399700931,4.86288173194361));
#15820=CARTESIAN_POINT('Ctrl Pts',(-3.6973382267209,2.53554710104677,4.86658632829587));
#15821=CARTESIAN_POINT('Ctrl Pts',(-3.73990668943618,2.50497810589362,4.87010689764359));
#15822=CARTESIAN_POINT('Ctrl Pts',(-3.76665058188897,2.4523728080809,4.8736274669913));
#15823=CARTESIAN_POINT('Ctrl Pts',(-3.76685809662611,2.39994994258553,4.87714803633902));
#15824=CARTESIAN_POINT('Origin',(-3.6,2.4,4.7));
#15825=CARTESIAN_POINT('',(-3.76657659596252,2.40015219042981,4.94714803633902));
#15826=CARTESIAN_POINT('',(-3.76633013671136,2.4000063325357,4.92785196366098));
#15827=CARTESIAN_POINT('',(-3.7666,2.4,4.7));
#15828=CARTESIAN_POINT('Ctrl Pts',(-3.76633013671136,2.4000063325357,4.92785196366098));
#15829=CARTESIAN_POINT('Ctrl Pts',(-3.76633943338483,2.42742681836579,4.926025371501));
#15830=CARTESIAN_POINT('Ctrl Pts',(-3.75993532163491,2.454843216144,4.92419877934102));
#15831=CARTESIAN_POINT('Ctrl Pts',(-3.74709395519472,2.478810633836,4.92237218718103));
#15832=CARTESIAN_POINT('Ctrl Pts',(-3.72104978380566,2.52742006625356,4.91866759082877));
#15833=CARTESIAN_POINT('Ctrl Pts',(-3.66852675119931,2.56184254018683,4.9149629944765));
#15834=CARTESIAN_POINT('Ctrl Pts',(-3.61356232107187,2.56632441524918,4.91125839812423));
#15835=CARTESIAN_POINT('Ctrl Pts',(-3.55859789094443,2.57080629031153,4.90755380177196));
#15836=CARTESIAN_POINT('Ctrl Pts',(-3.5011920632959,2.54534756650297,4.90384920541969));
#15837=CARTESIAN_POINT('Ctrl Pts',(-3.46761694066379,2.50159957313644,4.90014460906742));
#15838=CARTESIAN_POINT('Ctrl Pts',(-3.43404181803167,2.45785157976992,4.89644001271516));
#15839=CARTESIAN_POINT('Ctrl Pts',(-3.42429740041597,2.39581431684543,4.89273541636289));
#15840=CARTESIAN_POINT('Ctrl Pts',(-3.44284327579263,2.34387948951498,4.88903082001062));
#15841=CARTESIAN_POINT('Ctrl Pts',(-3.46138915116929,2.29194466218454,4.88532622365835));
#15842=CARTESIAN_POINT('Ctrl Pts',(-3.50822531953831,2.25011227044814,4.88162162730609));
#15843=CARTESIAN_POINT('Ctrl Pts',(-3.56191694286671,2.23752714559004,4.87791703095382));
#15844=CARTESIAN_POINT('Ctrl Pts',(-3.61560856619511,2.22494202073194,4.87421243460155));
#15845=CARTESIAN_POINT('Ctrl Pts',(-3.6761556444829,2.24160416275214,4.87050783824928));
#15846=CARTESIAN_POINT('Ctrl Pts',(-3.71584846402625,2.27988804787417,4.86680324189701));
#15847=CARTESIAN_POINT('Ctrl Pts',(-3.7478178913646,2.31072268995097,4.863819482485));
#15848=CARTESIAN_POINT('Ctrl Pts',(-3.76625910135787,2.35558341867251,4.86083572307299));
#15849=CARTESIAN_POINT('Ctrl Pts',(-3.7666675037778,2.40014587506062,4.85785196366098));
#15850=CARTESIAN_POINT('Ctrl Pts',(-3.76685809662611,2.39994994258553,4.87714803633902));
#15851=CARTESIAN_POINT('Ctrl Pts',(-3.76686894382487,2.39720969748472,4.87733206334357));
#15852=CARTESIAN_POINT('Ctrl Pts',(-3.76680728418873,2.39446995085397,4.87751609034812));
#15853=CARTESIAN_POINT('Ctrl Pts',(-3.76667158779769,2.39173387609673,4.87770011735268));
#15854=CARTESIAN_POINT('Ctrl Pts',(-3.76393992155949,2.33665471752516,4.88140471370494));
#15855=CARTESIAN_POINT('Ctrl Pts',(-3.73120516079181,2.28306357079796,4.88510931005722));
#15856=CARTESIAN_POINT('Ctrl Pts',(-3.68344855437882,2.25548672809881,4.88881390640948));
#15857=CARTESIAN_POINT('Ctrl Pts',(-3.63569194796583,2.22790988539967,4.89251850276175));
#15858=CARTESIAN_POINT('Ctrl Pts',(-3.57291349590753,2.22634734672859,4.89622309911402));
#15859=CARTESIAN_POINT('Ctrl Pts',(-3.52384411276617,2.25151421676554,4.89992769546629));
#15860=CARTESIAN_POINT('Ctrl Pts',(-3.47477472962482,2.27668108680249,4.90363229181855));
#15861=CARTESIAN_POINT('Ctrl Pts',(-3.43941441540042,2.32857736554749,4.90733688817082));
#15862=CARTESIAN_POINT('Ctrl Pts',(-3.43394601840489,2.38345242676704,4.91104148452309));
#15863=CARTESIAN_POINT('Ctrl Pts',(-3.42847762140937,2.4383274879866,4.91474608087536));
#15864=CARTESIAN_POINT('Ctrl Pts',(-3.45290114164273,2.49618133168073,4.91845067722763));
#15865=CARTESIAN_POINT('Ctrl Pts',(-3.49603901657836,2.530536818217,4.9221552735799));
#15866=CARTESIAN_POINT('Ctrl Pts',(-3.539176891514,2.56489230475327,4.92585986993216));
#15867=CARTESIAN_POINT('Ctrl Pts',(-3.60102912115191,2.5757494341317,4.92956446628443));
#15868=CARTESIAN_POINT('Ctrl Pts',(-3.65328868187437,2.55813937955255,4.9332690626367));
#15869=CARTESIAN_POINT('Ctrl Pts',(-3.70554824259683,2.54052932497339,4.93697365898897));
#15870=CARTESIAN_POINT('Ctrl Pts',(-3.74821513440384,2.49445208643666,4.94067825534123));
#15871=CARTESIAN_POINT('Ctrl Pts',(-3.76176261231807,2.4409951733855,4.9443828516935));
#15872=CARTESIAN_POINT('Ctrl Pts',(-3.76513331494005,2.42769473782655,4.94530457990868));
#15873=CARTESIAN_POINT('Ctrl Pts',(-3.7667013875235,2.41393746536136,4.94622630812385));
#15874=CARTESIAN_POINT('Ctrl Pts',(-3.76657659596252,2.40015219042981,4.94714803633902));
#15875=CARTESIAN_POINT('Origin',(-3.6,2.4,4.7));
#15876=CARTESIAN_POINT('',(-3.76634000089015,2.39995738785102,5.01714803633902));
#15877=CARTESIAN_POINT('',(-3.76664425875303,2.39985083704439,4.99785196366098));
#15878=CARTESIAN_POINT('',(-3.7666,2.4,4.7));
#15879=CARTESIAN_POINT('Ctrl Pts',(-3.76664425875303,2.39985083704439,4.99785196366098));
#15880=CARTESIAN_POINT('Ctrl Pts',(-3.76623994328637,2.44366117230771,4.99491961628127));
#15881=CARTESIAN_POINT('Ctrl Pts',(-3.74849621432459,2.48776127465667,4.99198726890157));
#15882=CARTESIAN_POINT('Ctrl Pts',(-3.71750016303509,2.5184966637895,4.98905492152186));
#15883=CARTESIAN_POINT('Ctrl Pts',(-3.67834114001603,2.55732637791376,4.98535032516959));
#15884=CARTESIAN_POINT('Ctrl Pts',(-3.61803053064114,2.57482512236184,4.98164572881732));
#15885=CARTESIAN_POINT('Ctrl Pts',(-3.56416982715023,2.56298449736068,4.97794113246505));
#15886=CARTESIAN_POINT('Ctrl Pts',(-3.51030912365932,2.55114387235952,4.97423653611279));
#15887=CARTESIAN_POINT('Ctrl Pts',(-3.46289832605237,2.50996387790913,4.97053193976052));
#15888=CARTESIAN_POINT('Ctrl Pts',(-3.44363525475417,2.45829077205198,4.96682734340825));
#15889=CARTESIAN_POINT('Ctrl Pts',(-3.42437218345597,2.40661766619482,4.96312274705598));
#15890=CARTESIAN_POINT('Ctrl Pts',(-3.4332568384665,2.34445144893089,4.95941815070372));
#15891=CARTESIAN_POINT('Ctrl Pts',(-3.4662231070096,2.30024284205961,4.95571355435145));
#15892=CARTESIAN_POINT('Ctrl Pts',(-3.4991893755527,2.25603423518832,4.95200895799918));
#15893=CARTESIAN_POINT('Ctrl Pts',(-3.55623725762836,2.22978323870968,4.94830436164691));
#15894=CARTESIAN_POINT('Ctrl Pts',(-3.61125846653673,2.23350377003431,4.94459976529464));
#15895=CARTESIAN_POINT('Ctrl Pts',(-3.66627967544511,2.23722430135893,4.94089516894237));
#15896=CARTESIAN_POINT('Ctrl Pts',(-3.71927421118621,2.27091636048683,4.9371905725901));
#15897=CARTESIAN_POINT('Ctrl Pts',(-3.74598882397087,2.31916058550171,4.93348597623784));
#15898=CARTESIAN_POINT('Ctrl Pts',(-3.75953150177818,2.3436174623693,4.93160797204555));
#15899=CARTESIAN_POINT('Ctrl Pts',(-3.76632057836981,2.37181405816179,4.92972996785327));
#15900=CARTESIAN_POINT('Ctrl Pts',(-3.76633013671136,2.4000063325357,4.92785196366098));
#15901=CARTESIAN_POINT('Ctrl Pts',(-3.76657659596252,2.40015219042981,4.94714803633902));
#15902=CARTESIAN_POINT('Ctrl Pts',(-3.76619982713509,2.35853189310505,4.94993090447612));
#15903=CARTESIAN_POINT('Ctrl Pts',(-3.7503917908276,2.31665633988757,4.95271377261321));
#15904=CARTESIAN_POINT('Ctrl Pts',(-3.72217338919013,2.28632762005297,4.95549664075031));
#15905=CARTESIAN_POINT('Ctrl Pts',(-3.68460862412651,2.24595356733716,4.95920123710258));
#15906=CARTESIAN_POINT('Ctrl Pts',(-3.62505102997782,2.22604204947114,4.96290583345484));
#15907=CARTESIAN_POINT('Ctrl Pts',(-3.57075747740423,2.23570568531624,4.96661042980711));
#15908=CARTESIAN_POINT('Ctrl Pts',(-3.51646392483064,2.24536932116134,4.97031502615938));
#15909=CARTESIAN_POINT('Ctrl Pts',(-3.46743441383215,2.28460811071757,4.97401962251165));
#15910=CARTESIAN_POINT('Ctrl Pts',(-3.44610757816651,2.33546419983794,4.97772421886392));
#15911=CARTESIAN_POINT('Ctrl Pts',(-3.42478074250087,2.38632028895831,4.98142881521618));
#15912=CARTESIAN_POINT('Ctrl Pts',(-3.43115658216808,2.44879367764282,4.98513341156845));
#15913=CARTESIAN_POINT('Ctrl Pts',(-3.46231715792478,2.49429306452592,4.98883800792072));
#15914=CARTESIAN_POINT('Ctrl Pts',(-3.49347773368148,2.53979245140902,4.99254260427299));
#15915=CARTESIAN_POINT('Ctrl Pts',(-3.54942304552767,2.56831783649071,4.99624720062526));
#15916=CARTESIAN_POINT('Ctrl Pts',(-3.60454940439799,2.56681441711196,4.99995179697753));
#15917=CARTESIAN_POINT('Ctrl Pts',(-3.6596757632683,2.5653109977332,5.00365639332979));
#15918=CARTESIAN_POINT('Ctrl Pts',(-3.71398316916273,2.533778773894,5.00736098968206));
#15919=CARTESIAN_POINT('Ctrl Pts',(-3.7426175295644,2.48664864348361,5.01106558603433));
#15920=CARTESIAN_POINT('Ctrl Pts',(-3.75828878922747,2.46085485932866,5.01309306946923));
#15921=CARTESIAN_POINT('Ctrl Pts',(-3.76627033413891,2.43038911475947,5.01512055290412));
#15922=CARTESIAN_POINT('Ctrl Pts',(-3.76634000089015,2.39995738785102,5.01714803633902));
#15923=CARTESIAN_POINT('Origin',(-3.6,2.4,4.7));
#15924=CARTESIAN_POINT('',(-3.76673280722786,2.39986996770474,5.08714803633902));
#15925=CARTESIAN_POINT('',(-3.76682061973634,2.40008640134019,5.06785196366098));
#15926=CARTESIAN_POINT('',(-3.7666,2.4,4.7));
#15927=CARTESIAN_POINT('Ctrl Pts',(-3.76682061973634,2.40008640134019,5.06785196366098));
#15928=CARTESIAN_POINT('Ctrl Pts',(-3.76685198409984,2.40505542063702,5.06751845741382));
#15929=CARTESIAN_POINT('Ctrl Pts',(-3.76664920930319,2.41002184448446,5.06718495116665));
#15930=CARTESIAN_POINT('Ctrl Pts',(-3.76620395659798,2.41496643342036,5.06685144491949));
#15931=CARTESIAN_POINT('Ctrl Pts',(-3.76125807758801,2.46989106014367,5.06314684856722));
#15932=CARTESIAN_POINT('Ctrl Pts',(-3.7263932711654,2.5221215151067,5.05944225221495));
#15933=CARTESIAN_POINT('Ctrl Pts',(-3.67756562981921,2.54775425401002,5.05573765586269));
#15934=CARTESIAN_POINT('Ctrl Pts',(-3.62873798847301,2.57338699291335,5.05203305951042));
#15935=CARTESIAN_POINT('Ctrl Pts',(-3.56594751220322,2.57242201575698,5.04832846315815));
#15936=CARTESIAN_POINT('Ctrl Pts',(-3.51793061046379,2.54530094002895,5.04462386680588));
#15937=CARTESIAN_POINT('Ctrl Pts',(-3.46991370872435,2.51817986430092,5.04091927045361));
#15938=CARTESIAN_POINT('Ctrl Pts',(-3.43667038151527,2.46490269000124,5.03721467410135));
#15939=CARTESIAN_POINT('Ctrl Pts',(-3.4334146300602,2.40985202293434,5.03351007774908));
#15940=CARTESIAN_POINT('Ctrl Pts',(-3.43015887860513,2.35480135586744,5.02980548139681));
#15941=CARTESIAN_POINT('Ctrl Pts',(-3.45689070290407,2.29797719603331,5.02610088504454));
#15942=CARTESIAN_POINT('Ctrl Pts',(-3.50137612997721,2.26538543995573,5.02239628869227));
#15943=CARTESIAN_POINT('Ctrl Pts',(-3.54586155705034,2.23279368387816,5.01869169234));
#15944=CARTESIAN_POINT('Ctrl Pts',(-3.60810058689768,2.22443433155712,5.01498709598773));
#15945=CARTESIAN_POINT('Ctrl Pts',(-3.65960917559394,2.24413308920132,5.01128249963547));
#15946=CARTESIAN_POINT('Ctrl Pts',(-3.7111177642902,2.26383184684551,5.0075779032832));
#15947=CARTESIAN_POINT('Ctrl Pts',(-3.75189591183539,2.31158871445493,5.00387330693093));
#15948=CARTESIAN_POINT('Ctrl Pts',(-3.76328126727638,2.36554749015986,5.00016871057866));
#15949=CARTESIAN_POINT('Ctrl Pts',(-3.76565462410273,2.37679557365843,4.9993964616061));
#15950=CARTESIAN_POINT('Ctrl Pts',(-3.76675073733939,2.38831315681292,4.99862421263354));
#15951=CARTESIAN_POINT('Ctrl Pts',(-3.76664425875303,2.39985083704439,4.99785196366098));
#15952=CARTESIAN_POINT('Ctrl Pts',(-3.76634000089015,2.39995738785102,5.01714803633902));
#15953=CARTESIAN_POINT('Ctrl Pts',(-3.76639762849214,2.37478458425737,5.01882514925639));
#15954=CARTESIAN_POINT('Ctrl Pts',(-3.76104161363815,2.34963505698934,5.02050226217376));
#15955=CARTESIAN_POINT('Ctrl Pts',(-3.75014621226255,2.32717238066401,5.02217937509113));
#15956=CARTESIAN_POINT('Ctrl Pts',(-3.72607921965016,2.27755428523638,5.0258839714434));
#15957=CARTESIAN_POINT('Ctrl Pts',(-3.67498391951647,2.2410461313627,5.02958856779567));
#15958=CARTESIAN_POINT('Ctrl Pts',(-3.62024436463387,2.23435607004762,5.03329316414794));
#15959=CARTESIAN_POINT('Ctrl Pts',(-3.56550480975127,2.22766600873255,5.03699776050021));
#15960=CARTESIAN_POINT('Ctrl Pts',(-3.50712100011975,2.25079403997609,5.04070235685247));
#15961=CARTESIAN_POINT('Ctrl Pts',(-3.47181261940603,2.29315551442515,5.04440695320474));
#15962=CARTESIAN_POINT('Ctrl Pts',(-3.43650423869231,2.33551698887421,5.04811154955701));
#15963=CARTESIAN_POINT('Ctrl Pts',(-3.42427128689639,2.39711190652879,5.05181614590928));
#15964=CARTESIAN_POINT('Ctrl Pts',(-3.44071223950815,2.44975095341954,5.05552074226154));
#15965=CARTESIAN_POINT('Ctrl Pts',(-3.45715319211991,2.50239000031029,5.05922533861381));
#15966=CARTESIAN_POINT('Ctrl Pts',(-3.50226804913935,2.54607317643722,5.06292993496608));
#15967=CARTESIAN_POINT('Ctrl Pts',(-3.55540974897266,2.56080872993518,5.06663453131835));
#15968=CARTESIAN_POINT('Ctrl Pts',(-3.60855144880598,2.57554428343315,5.07033912767062));
#15969=CARTESIAN_POINT('Ctrl Pts',(-3.66971999145316,2.56133221430215,5.07404372402289));
#15970=CARTESIAN_POINT('Ctrl Pts',(-3.71092122942369,2.52467655355957,5.07774832037516));
#15971=CARTESIAN_POINT('Ctrl Pts',(-3.74576802490479,2.49367427362722,5.08088155902978));
#15972=CARTESIAN_POINT('Ctrl Pts',(-3.76633165033452,2.44661746651941,5.0840147976844));
#15973=CARTESIAN_POINT('Ctrl Pts',(-3.76673280722786,2.39986996770474,5.08714803633902));
#15974=CARTESIAN_POINT('Origin',(-3.6,2.4,4.7));
#15975=CARTESIAN_POINT('',(-3.76674783252531,2.40012156540224,5.15714803633902));
#15976=CARTESIAN_POINT('',(-3.76638442018051,2.4000942147675,5.13785196366098));
#15977=CARTESIAN_POINT('',(-3.7666,2.4,4.7));
#15978=CARTESIAN_POINT('',(-3.47309291201476,2.50793586530485,5.2));
#15979=CARTESIAN_POINT('Ctrl Pts',(-3.76674783252531,2.40012156540224,5.15714803633902));
#15980=CARTESIAN_POINT('Ctrl Pts',(-3.76635429688688,2.35284438834095,5.16031823516921));
#15981=CARTESIAN_POINT('Ctrl Pts',(-3.74524547308137,2.30526839815283,5.1634884339994));
#15982=CARTESIAN_POINT('Ctrl Pts',(-3.70967617106781,2.27424023606977,5.16665863282959));
#15983=CARTESIAN_POINT('Ctrl Pts',(-3.66811098429235,2.23798168503636,5.17036322918186));
#15984=CARTESIAN_POINT('Ctrl Pts',(-3.60679923783928,2.22432008207827,5.17406782553412));
#15985=CARTESIAN_POINT('Ctrl Pts',(-3.55380863333633,2.23961508023379,5.17777242188639));
#15986=CARTESIAN_POINT('Ctrl Pts',(-3.50081802883339,2.2549100783893,5.18147701823866));
#15987=CARTESIAN_POINT('Ctrl Pts',(-3.45614856628056,2.29916167765842,5.18518161459093));
#15988=CARTESIAN_POINT('Ctrl Pts',(-3.44024447629705,2.35186821788708,5.1888862109432));
#15989=CARTESIAN_POINT('Ctrl Pts',(-3.42434038631354,2.40457475811575,5.19259080729547));
#15990=CARTESIAN_POINT('Ctrl Pts',(-3.43720166889934,2.46573623930395,5.19629540364773));
#15991=CARTESIAN_POINT('Ctrl Pts',(-3.47309291201476,2.50793586530485,5.2));
#15992=CARTESIAN_POINT('',(-3.72714753727462,2.50812032359617,5.2));
#15993=CARTESIAN_POINT('Origin',(-3.6,2.4,5.2));
#15994=CARTESIAN_POINT('Ctrl Pts',(-3.72714768981588,2.50812044061668,5.2));
#15995=CARTESIAN_POINT('Ctrl Pts',(-3.69206189497277,2.54927257104909,5.19636770818145));
#15996=CARTESIAN_POINT('Ctrl Pts',(-3.63506413165932,2.57187758396405,5.19273541636289));
#15997=CARTESIAN_POINT('Ctrl Pts',(-3.58132375091077,2.56581791151438,5.18910312454434));
#15998=CARTESIAN_POINT('Ctrl Pts',(-3.52651361217864,2.55963761500343,5.18539852819207));
#15999=CARTESIAN_POINT('Ctrl Pts',(-3.475091829903,2.5236400741886,5.1816939318398));
#16000=CARTESIAN_POINT('Ctrl Pts',(-3.45055836676857,2.47425895866487,5.17798933548753));
#16001=CARTESIAN_POINT('Ctrl Pts',(-3.42602490363414,2.42487784314114,5.17428473913526));
#16002=CARTESIAN_POINT('Ctrl Pts',(-3.42837975964092,2.3621131529085,5.17058014278299));
#16003=CARTESIAN_POINT('Ctrl Pts',(-3.4565619363393,2.31470980183002,5.16687554643073));
#16004=CARTESIAN_POINT('Ctrl Pts',(-3.48474411303769,2.26730645075154,5.16317095007846));
#16005=CARTESIAN_POINT('Ctrl Pts',(-3.53875361042767,2.23526443882722,5.15946635372619));
#16006=CARTESIAN_POINT('Ctrl Pts',(-3.59386432951576,2.23323784347702,5.15576175737392));
#16007=CARTESIAN_POINT('Ctrl Pts',(-3.64897504860385,2.23121124812682,5.15205716102166));
#16008=CARTESIAN_POINT('Ctrl Pts',(-3.70518698939006,2.25920006935074,5.14835256466939));
#16009=CARTESIAN_POINT('Ctrl Pts',(-3.73677860664843,2.30440012364175,5.14464796831712));
#16010=CARTESIAN_POINT('Ctrl Pts',(-3.75609666072391,2.3320396422478,5.14238263343174));
#16011=CARTESIAN_POINT('Ctrl Pts',(-3.76620859139621,2.36611484945711,5.14011729854636));
#16012=CARTESIAN_POINT('Ctrl Pts',(-3.76638442018051,2.4000942147675,5.13785196366098));
#16013=CARTESIAN_POINT('Origin',(-3.6,2.4,5.35459252805377));
#16014=CARTESIAN_POINT('',(-3.80572269346025,2.40011955618633,4.34540747194623));
#16015=CARTESIAN_POINT('',(-3.8051611014991,2.39991986595833,4.33959252805377));
#16016=CARTESIAN_POINT('',(-3.805475,2.40000000000001,5.35459252805377));
#16017=CARTESIAN_POINT('',(-3.41173724903364,2.31767678198965,4.3));
#16018=CARTESIAN_POINT('Ctrl Pts',(-3.8051611014991,2.39991986595833,4.33959252805377));
#16019=CARTESIAN_POINT('Ctrl Pts',(-3.80504328807488,2.43847991504582,4.33750880775932));
#16020=CARTESIAN_POINT('Ctrl Pts',(-3.77605831390311,2.54576383181508,4.33172049111259));
#16021=CARTESIAN_POINT('Ctrl Pts',(-3.60297477126067,2.64299057240655,4.32222757811361));
#16022=CARTESIAN_POINT('Ctrl Pts',(-3.39749753058122,2.53388381093044,4.3111137890568));
#16023=CARTESIAN_POINT('Ctrl Pts',(-3.38436282049399,2.380278625644,4.30370459635227));
#16024=CARTESIAN_POINT('Ctrl Pts',(-3.41173724903364,2.31767678198965,4.3));
#16025=CARTESIAN_POINT('',(-3.47764162137361,2.23446466486417,4.3));
#16026=CARTESIAN_POINT('Origin',(-3.6,2.4,4.3));
#16027=CARTESIAN_POINT('Ctrl Pts',(-3.80572269346025,2.40011955618633,4.34540747194623));
#16028=CARTESIAN_POINT('Ctrl Pts',(-3.80577296183019,2.40728359294699,4.34501772883951));
#16029=CARTESIAN_POINT('Ctrl Pts',(-3.80218372831243,2.48249299452007,4.34092338938053));
#16030=CARTESIAN_POINT('Ctrl Pts',(-3.70962996035205,2.61673302206395,4.33312445356927));
#16031=CARTESIAN_POINT('Ctrl Pts',(-3.47734458963256,2.60960762555316,4.32201066451247));
#16032=CARTESIAN_POINT('Ctrl Pts',(-3.35820165688085,2.41200908723629,4.31096917998938));
#16033=CARTESIAN_POINT('Ctrl Pts',(-3.42405717417692,2.27417969332383,4.30363229181855));
#16034=CARTESIAN_POINT('Ctrl Pts',(-3.477641490197,2.23446446733471,4.3));
#16035=CARTESIAN_POINT('Origin',(-3.6,2.4,5.35459252805377));
#16036=CARTESIAN_POINT('',(-3.8051926580795,2.40010265427736,4.41540747194623));
#16037=CARTESIAN_POINT('',(-3.80566724099481,2.39985021907517,4.40959252805377));
#16038=CARTESIAN_POINT('',(-3.805475,2.40000000000001,5.35459252805377));
#16039=CARTESIAN_POINT('Ctrl Pts',(-3.80566724099481,2.39985021907517,4.40959252805377));
#16040=CARTESIAN_POINT('Ctrl Pts',(-3.80518613776288,2.45851948579172,4.40640305253959));
#16041=CARTESIAN_POINT('Ctrl Pts',(-3.74813828696622,2.58615032985374,4.39950898067314));
#16042=CARTESIAN_POINT('Ctrl Pts',(-3.53156902199863,2.63302754596983,4.38891031245443));
#16043=CARTESIAN_POINT('Ctrl Pts',(-3.36710794775451,2.46888245639993,4.37779652339763));
#16044=CARTESIAN_POINT('Ctrl Pts',(-3.41581895566904,2.24170428297288,4.36668273434082));
#16045=CARTESIAN_POINT('Ctrl Pts',(-3.63310626324856,2.15938431915927,4.35556894528402));
#16046=CARTESIAN_POINT('Ctrl Pts',(-3.78504422722635,2.27149586782626,4.34653887652167));
#16047=CARTESIAN_POINT('Ctrl Pts',(-3.80525274573711,2.36992492828818,4.34121340411158));
#16048=CARTESIAN_POINT('Ctrl Pts',(-3.8051611014991,2.39991986595833,4.33959252805377));
#16049=CARTESIAN_POINT('Ctrl Pts',(-3.8051926580795,2.40010265427736,4.41540747194623));
#16050=CARTESIAN_POINT('Ctrl Pts',(-3.80531782228225,2.42777437777342,4.41391197361979));
#16051=CARTESIAN_POINT('Ctrl Pts',(-3.78721617252902,2.52383659362796,4.40871187894108));
#16052=CARTESIAN_POINT('Ctrl Pts',(-3.64121277856108,2.63934345799643,4.3998071879101));
#16053=CARTESIAN_POINT('Ctrl Pts',(-3.4212652433475,2.56443108225311,4.38869339885329));
#16054=CARTESIAN_POINT('Ctrl Pts',(-3.36491712045917,2.33901445477475,4.3775796097965));
#16055=CARTESIAN_POINT('Ctrl Pts',(-3.52374009472539,2.16941582002738,4.36646582073968));
#16056=CARTESIAN_POINT('Ctrl Pts',(-3.7443527804805,2.20942499341216,4.3557417747896));
#16057=CARTESIAN_POINT('Ctrl Pts',(-3.80529514960796,2.33918780371163,4.34872232519178));
#16058=CARTESIAN_POINT('Ctrl Pts',(-3.80572269346025,2.40011955618633,4.34540747194623));
#16059=CARTESIAN_POINT('Origin',(-3.6,2.4,5.35459252805377));
#16060=CARTESIAN_POINT('',(-3.80534990670044,2.39982347234431,4.48540747194623));
#16061=CARTESIAN_POINT('',(-3.80562878067403,2.40016339023914,4.47959252805377));
#16062=CARTESIAN_POINT('',(-3.805475,2.40000000000001,5.35459252805377));
#16063=CARTESIAN_POINT('Ctrl Pts',(-3.80562878067403,2.40016339023914,4.47959252805377));
#16064=CARTESIAN_POINT('Ctrl Pts',(-3.80572325245773,2.41103322160878,4.47900189367213));
#16065=CARTESIAN_POINT('Ctrl Pts',(-3.79999615010417,2.4899814340984,4.47470666293823));
#16066=CARTESIAN_POINT('Ctrl Pts',(-3.69773850528383,2.62233049702197,4.46670683585206));
#16067=CARTESIAN_POINT('Ctrl Pts',(-3.46621554861493,2.60269535293104,4.45559304679526));
#16068=CARTESIAN_POINT('Ctrl Pts',(-3.35714699158608,2.39753073103871,4.44447925773845));
#16069=CARTESIAN_POINT('Ctrl Pts',(-3.47036459922058,2.19462650439043,4.43336546868165));
#16070=CARTESIAN_POINT('Ctrl Pts',(-3.70223885539349,2.17970247609322,4.42225167962484));
#16071=CARTESIAN_POINT('Ctrl Pts',(-3.80084479883202,2.31283530811152,4.41432736608222));
#16072=CARTESIAN_POINT('Ctrl Pts',(-3.80574494226542,2.39037475462753,4.41010764889186));
#16073=CARTESIAN_POINT('Ctrl Pts',(-3.80566724099481,2.39985021907517,4.40959252805377));
#16074=CARTESIAN_POINT('Ctrl Pts',(-3.80534990670044,2.39982347234431,4.48540747194623));
#16075=CARTESIAN_POINT('Ctrl Pts',(-3.804956326745,2.4478627067473,4.48280621840006));
#16076=CARTESIAN_POINT('Ctrl Pts',(-3.76418777279803,2.56491922132028,4.47650036850163));
#16077=CARTESIAN_POINT('Ctrl Pts',(-3.56918135753979,2.64090223654315,4.46648992225092));
#16078=CARTESIAN_POINT('Ctrl Pts',(-3.38089014394226,2.50475947474088,4.45537613319412));
#16079=CARTESIAN_POINT('Ctrl Pts',(-3.3931526891646,2.27272919910994,4.44426234413731));
#16080=CARTESIAN_POINT('Ctrl Pts',(-3.59474487835949,2.15719128792351,4.43314855508051));
#16081=CARTESIAN_POINT('Ctrl Pts',(-3.77337323137102,2.2495401787091,4.42353026435015));
#16082=CARTESIAN_POINT('Ctrl Pts',(-3.80500776987982,2.35922694839029,4.41761656997206));
#16083=CARTESIAN_POINT('Ctrl Pts',(-3.8051926580795,2.40010265427736,4.41540747194623));
#16084=CARTESIAN_POINT('Origin',(-3.6,2.4,5.35459252805377));
#16085=CARTESIAN_POINT('',(-3.80581594817644,2.40000082772184,4.55540747194624));
#16086=CARTESIAN_POINT('',(-3.80515175559583,2.40004689761323,4.54959252805377));
#16087=CARTESIAN_POINT('',(-3.805475,2.40000000000001,5.35459252805377));
#16088=CARTESIAN_POINT('Ctrl Pts',(-3.80515175559583,2.40004689761323,4.54959252805377));
#16089=CARTESIAN_POINT('Ctrl Pts',(-3.80521586484871,2.43145144073697,4.54789613845241));
#16090=CARTESIAN_POINT('Ctrl Pts',(-3.78367650680796,2.53135422698056,4.54249515249878));
#16091=CARTESIAN_POINT('Ctrl Pts',(-3.62821111800771,2.64122148806661,4.53338957019289));
#16092=CARTESIAN_POINT('Ctrl Pts',(-3.41263638408026,2.55452685581013,4.52227578113608));
#16093=CARTESIAN_POINT('Ctrl Pts',(-3.36855769224962,2.32639203807509,4.51116199207928));
#16094=CARTESIAN_POINT('Ctrl Pts',(-3.536320770243,2.1656314264689,4.50004820302247));
#16095=CARTESIAN_POINT('Ctrl Pts',(-3.75035693400944,2.21653400528296,4.48952504834731));
#16096=CARTESIAN_POINT('Ctrl Pts',(-3.80513070343558,2.34285510855967,4.4827064900244));
#16097=CARTESIAN_POINT('Ctrl Pts',(-3.80562878067403,2.40016339023914,4.47959252805377));
#16098=CARTESIAN_POINT('Ctrl Pts',(-3.80581594649383,2.40000082771776,4.55540747194623));
#16099=CARTESIAN_POINT('Ctrl Pts',(-3.80581594913922,2.4000451187351,4.55540505953261));
#16100=CARTESIAN_POINT('Ctrl Pts',(-3.80579587912807,2.46810441912583,4.55169805076672));
#16101=CARTESIAN_POINT('Ctrl Pts',(-3.73158417538336,2.60413054603043,4.54428644564855));
#16102=CARTESIAN_POINT('Ctrl Pts',(-3.49986236476522,2.62126031969194,4.53317265659175));
#16103=CARTESIAN_POINT('Ctrl Pts',(-3.35979766713961,2.43586801331045,4.52205886753494));
#16104=CARTESIAN_POINT('Ctrl Pts',(-3.43959288921302,2.2176453079079,4.51094507847814));
#16105=CARTESIAN_POINT('Ctrl Pts',(-3.66621055822496,2.16633391955349,4.49983128942134));
#16106=CARTESIAN_POINT('Ctrl Pts',(-3.79336822071197,2.29085017253336,4.4913187539107));
#16107=CARTESIAN_POINT('Ctrl Pts',(-3.80551684683325,2.37944724113564,4.48651081475233));
#16108=CARTESIAN_POINT('Ctrl Pts',(-3.80534990670044,2.39982347234431,4.48540747194623));
#16109=CARTESIAN_POINT('Origin',(-3.6,2.4,5.35459252805377));
#16110=CARTESIAN_POINT('',(-3.80534749188876,2.40017600730441,4.62540747194623));
#16111=CARTESIAN_POINT('',(-3.80545679372687,2.39981210841117,4.61959252805377));
#16112=CARTESIAN_POINT('',(-3.805475,2.40000000000001,5.35459252805377));
#16113=CARTESIAN_POINT('Ctrl Pts',(-3.80545679372687,2.39981210841117,4.61959252805377));
#16114=CARTESIAN_POINT('Ctrl Pts',(-3.80498629190864,2.45149295693423,4.61679038323268));
#16115=CARTESIAN_POINT('Ctrl Pts',(-3.75902063818539,2.5722445101987,4.61028364205933));
#16116=CARTESIAN_POINT('Ctrl Pts',(-3.55620097488638,2.63888348417682,4.60007230453371));
#16117=CARTESIAN_POINT('Ctrl Pts',(-3.3755463800872,2.4927590756963,4.58895851547691));
#16118=CARTESIAN_POINT('Ctrl Pts',(-3.40033672906513,2.26173123324197,4.5778447264201));
#16119=CARTESIAN_POINT('Ctrl Pts',(-3.60788113427776,2.15726236113484,4.5667309373633));
#16120=CARTESIAN_POINT('Ctrl Pts',(-3.77763371313004,2.25700670057819,4.55731353790785));
#16121=CARTESIAN_POINT('Ctrl Pts',(-3.80507586227844,2.36286981549731,4.55160073480468));
#16122=CARTESIAN_POINT('Ctrl Pts',(-3.80515175559583,2.40004689761323,4.54959252805377));
#16123=CARTESIAN_POINT('Ctrl Pts',(-3.80534749188876,2.40017600730441,4.62540747194623));
#16124=CARTESIAN_POINT('Ctrl Pts',(-3.80551452420589,2.42064195120264,4.62429930431288));
#16125=CARTESIAN_POINT('Ctrl Pts',(-3.79329841012664,2.50933048388748,4.61948654032726));
#16126=CARTESIAN_POINT('Ctrl Pts',(-3.66590691767206,2.63375190534549,4.61096917998937));
#16127=CARTESIAN_POINT('Ctrl Pts',(-3.43935610442817,2.58214613327058,4.59985539093257));
#16128=CARTESIAN_POINT('Ctrl Pts',(-3.35984447062414,2.36381993973287,4.58874160187577));
#16129=CARTESIAN_POINT('Ctrl Pts',(-3.50014991641224,2.17860976567263,4.57762781281897));
#16130=CARTESIAN_POINT('Ctrl Pts',(-3.73179898227351,2.19603680019893,4.56651643617579));
#16131=CARTESIAN_POINT('Ctrl Pts',(-3.80581188677276,2.33203010689162,4.55910965588488));
#16132=CARTESIAN_POINT('Ctrl Pts',(-3.80581594649383,2.40000082771776,4.55540747194623));
#16133=CARTESIAN_POINT('Origin',(-3.6,2.4,5.35459252805377));
#16134=CARTESIAN_POINT('',(-3.80519403776112,2.3998960891277,4.69540747194623));
#16135=CARTESIAN_POINT('',(-3.80578859626649,2.40006787741036,4.68959252805377));
#16136=CARTESIAN_POINT('',(-3.805475,2.40000000000001,5.35459252805377));
#16137=CARTESIAN_POINT('Ctrl Pts',(-3.80578859626649,2.40006787741036,4.68959252805377));
#16138=CARTESIAN_POINT('Ctrl Pts',(-3.80580466836371,2.40380178606869,4.68938922436523));
#16139=CARTESIAN_POINT('Ctrl Pts',(-3.8040203778982,2.4755592442775,4.68548132432442));
#16140=CARTESIAN_POINT('Ctrl Pts',(-3.7203544535977,2.61094662622203,4.67786882793133));
#16141=CARTESIAN_POINT('Ctrl Pts',(-3.48804541599454,2.61552226041731,4.66675503887454));
#16142=CARTESIAN_POINT('Ctrl Pts',(-3.35820967878295,2.42282792546417,4.65564124981773));
#16143=CARTESIAN_POINT('Ctrl Pts',(-3.44968736466998,2.20923893144694,4.64452746076093));
#16144=CARTESIAN_POINT('Ctrl Pts',(-3.67874791033599,2.17025570685489,4.63341367170413));
#16145=CARTESIAN_POINT('Ctrl Pts',(-3.79614945128685,2.2983686897146,4.62510202746841));
#16146=CARTESIAN_POINT('Ctrl Pts',(-3.80560832232849,2.38316790767908,4.62049497958495));
#16147=CARTESIAN_POINT('Ctrl Pts',(-3.80545679372687,2.39981210841117,4.61959252805377));
#16148=CARTESIAN_POINT('Ctrl Pts',(-3.80519403776112,2.3998960891277,4.69540747194623));
#16149=CARTESIAN_POINT('Ctrl Pts',(-3.80500643965891,2.44086040425288,4.69319354909316));
#16150=CARTESIAN_POINT('Ctrl Pts',(-3.77326722861529,2.55063877508332,4.68727502988781));
#16151=CARTESIAN_POINT('Ctrl Pts',(-3.59442944478611,2.64280165560495,4.6776519143302));
#16152=CARTESIAN_POINT('Ctrl Pts',(-3.39298749751263,2.52700196401557,4.6665381252734));
#16153=CARTESIAN_POINT('Ctrl Pts',(-3.38102644144724,2.29495593446246,4.65542433621659));
#16154=CARTESIAN_POINT('Ctrl Pts',(-3.56949436685434,2.15905792937668,4.64431054715979));
#16155=CARTESIAN_POINT('Ctrl Pts',(-3.76430796130134,2.23525748954489,4.63430492573634));
#16156=CARTESIAN_POINT('Ctrl Pts',(-3.80495613638248,2.352224449347,4.62800390066515));
#16157=CARTESIAN_POINT('Ctrl Pts',(-3.80534749188876,2.40017600730441,4.62540747194623));
#16158=CARTESIAN_POINT('Origin',(-3.6,2.4,5.35459252805377));
#16159=CARTESIAN_POINT('',(-3.80572670757095,2.39987978133106,4.76540747194623));
#16160=CARTESIAN_POINT('',(-3.8052563985153,2.4001450986671,4.75959252805377));
#16161=CARTESIAN_POINT('',(-3.805475,2.40000000000001,5.35459252805377));
#16162=CARTESIAN_POINT('Ctrl Pts',(-3.8052563985153,2.4001450986671,4.75959252805377));
#16163=CARTESIAN_POINT('Ctrl Pts',(-3.80541421064946,2.4243482217442,4.7582834691455));
#16164=CARTESIAN_POINT('Ctrl Pts',(-3.79026314769432,2.51685423684082,4.75326981388497));
#16165=CARTESIAN_POINT('Ctrl Pts',(-3.65317165905879,2.6369735181158,4.74455156227217));
#16166=CARTESIAN_POINT('Ctrl Pts',(-3.42974255082951,2.57319374878213,4.73343777321536));
#16167=CARTESIAN_POINT('Ctrl Pts',(-3.36215201667677,2.35088777703746,4.72232398415856));
#16168=CARTESIAN_POINT('Ctrl Pts',(-3.51226643903938,2.1735347799409,4.71121019510176));
#16169=CARTESIAN_POINT('Ctrl Pts',(-3.73846936695489,2.20292040156477,4.70029970973349));
#16170=CARTESIAN_POINT('Ctrl Pts',(-3.80551180288158,2.33576256604952,4.6930938207175));
#16171=CARTESIAN_POINT('Ctrl Pts',(-3.80578859626649,2.40006787741036,4.68959252805377));
#16172=CARTESIAN_POINT('Ctrl Pts',(-3.80572670757095,2.39987978133106,4.76540747194623));
#16173=CARTESIAN_POINT('Ctrl Pts',(-3.80530256520545,2.46089806692785,4.76208779387343));
#16174=CARTESIAN_POINT('Ctrl Pts',(-3.74420122965308,2.59074745124221,4.75506351944836));
#16175=CARTESIAN_POINT('Ctrl Pts',(-3.52344221510783,2.63048336300545,4.74433464867103));
#16176=CARTESIAN_POINT('Ctrl Pts',(-3.36483726729874,2.46068083880743,4.73322085961422));
#16177=CARTESIAN_POINT('Ctrl Pts',(-3.42147943565789,2.23533645468145,4.72210707055742));
#16178=CARTESIAN_POINT('Ctrl Pts',(-3.64152350112028,2.16071048099716,4.71099328150062));
#16179=CARTESIAN_POINT('Ctrl Pts',(-3.7872979195691,2.27634402063526,4.70209341529689));
#16180=CARTESIAN_POINT('Ctrl Pts',(-3.80532035088855,2.37231408965339,4.69689814544543));
#16181=CARTESIAN_POINT('Ctrl Pts',(-3.80519403776112,2.3998960891277,4.69540747194623));
#16182=CARTESIAN_POINT('Origin',(-3.6,2.4,5.35459252805377));
#16183=CARTESIAN_POINT('',(-3.80555825533459,2.40017991403412,4.83540747194623));
#16184=CARTESIAN_POINT('',(-3.80526423105652,2.39985120339831,4.82959252805377));
#16185=CARTESIAN_POINT('',(-3.805475,2.40000000000001,5.35459252805377));
#16186=CARTESIAN_POINT('Ctrl Pts',(-3.80526423105652,2.39985120339831,4.82959252805377));
#16187=CARTESIAN_POINT('Ctrl Pts',(-3.80496496310342,2.44449429497159,4.82717771392578));
#16188=CARTESIAN_POINT('Ctrl Pts',(-3.76870077292898,2.55806758042747,4.82105830344552));
#16189=CARTESIAN_POINT('Ctrl Pts',(-3.58130943065524,2.64214527918755,4.81123429661299));
#16190=CARTESIAN_POINT('Ctrl Pts',(-3.38642339103422,2.51562311930547,4.80012050755619));
#16191=CARTESIAN_POINT('Ctrl Pts',(-3.38702644372307,2.28326980706774,4.78900671849939));
#16192=CARTESIAN_POINT('Ctrl Pts',(-3.58256660775658,2.15776096423133,4.77789292944257));
#16193=CARTESIAN_POINT('Ctrl Pts',(-3.76915215745557,2.24264335554317,4.76808819929404));
#16194=CARTESIAN_POINT('Ctrl Pts',(-3.80496760717513,2.35585412961529,4.76198806549777));
#16195=CARTESIAN_POINT('Ctrl Pts',(-3.8052563985153,2.4001450986671,4.75959252805377));
#16196=CARTESIAN_POINT('Ctrl Pts',(-3.80555825533459,2.40017991403412,4.83540747194623));
#16197=CARTESIAN_POINT('Ctrl Pts',(-3.80567994271202,2.41345772088563,4.83468663500598));
#16198=CARTESIAN_POINT('Ctrl Pts',(-3.79845785744155,2.49484232907173,4.83026120171345));
#16199=CARTESIAN_POINT('Ctrl Pts',(-3.68988494016744,2.62561997380774,4.82213117206865));
#16200=CARTESIAN_POINT('Ctrl Pts',(-3.45919254257122,2.59788111325323,4.81101738301186));
#16201=CARTESIAN_POINT('Ctrl Pts',(-3.35738280762477,2.38901942561361,4.79990359395505));
#16202=CARTESIAN_POINT('Ctrl Pts',(-3.47764334032546,2.19020838223802,4.78878980489825));
#16203=CARTESIAN_POINT('Ctrl Pts',(-3.70989831124516,2.18342198579874,4.77767601584144));
#16204=CARTESIAN_POINT('Ctrl Pts',(-3.8022342613798,2.31768599661427,4.76988190485744));
#16205=CARTESIAN_POINT('Ctrl Pts',(-3.80577588708354,2.39280468157954,4.7657923902257));
#16206=CARTESIAN_POINT('Ctrl Pts',(-3.80572670757095,2.39987978133106,4.76540747194623));
#16207=CARTESIAN_POINT('Origin',(-3.6,2.4,5.35459252805377));
#16208=CARTESIAN_POINT('',(-3.80514216591097,2.40000781019071,4.90540747194623));
#16209=CARTESIAN_POINT('',(-3.8057933217542,2.39993826202139,4.89959252805377));
#16210=CARTESIAN_POINT('',(-3.805475,2.40000000000001,5.35459252805377));
#16211=CARTESIAN_POINT('Ctrl Pts',(-3.8057933217542,2.39993826202139,4.89959252805377));
#16212=CARTESIAN_POINT('Ctrl Pts',(-3.80553738483576,2.46459365390411,4.89607195870605));
#16213=CARTESIAN_POINT('Ctrl Pts',(-3.73784442289473,2.59774586534896,4.88884679300607));
#16214=CARTESIAN_POINT('Ctrl Pts',(-3.51109208760397,2.62600676257303,4.87791703095382));
#16215=CARTESIAN_POINT('Ctrl Pts',(-3.36190028978558,2.44787694237367,4.86680324189701));
#16216=CARTESIAN_POINT('Ctrl Pts',(-3.43064385696086,2.2259248138587,4.85568945284022));
#16217=CARTESIAN_POINT('Ctrl Pts',(-3.65440102248913,2.16330567736551,4.8445756637834));
#16218=CARTESIAN_POINT('Ctrl Pts',(-3.7905654137645,2.28386779123864,4.83587668885459));
#16219=CARTESIAN_POINT('Ctrl Pts',(-3.80542407378798,2.37600677360117,4.83088231027805));
#16220=CARTESIAN_POINT('Ctrl Pts',(-3.80526423105652,2.39985120339831,4.82959252805377));
#16221=CARTESIAN_POINT('Ctrl Pts',(-3.80514216591096,2.40000781019071,4.90540747194623));
#16222=CARTESIAN_POINT('Ctrl Pts',(-3.80515363190124,2.43382668369574,4.90358087978625));
#16223=CARTESIAN_POINT('Ctrl Pts',(-3.78123591260341,2.53621991664107,4.898049691274));
#16224=CARTESIAN_POINT('Ctrl Pts',(-3.6197380796992,2.64206214751696,4.88881390640948));
#16225=CARTESIAN_POINT('Ctrl Pts',(-3.40733479453568,2.54786410535795,4.87770011735268));
#16226=CARTESIAN_POINT('Ctrl Pts',(-3.37128015690807,2.3183243706747,4.86658632829587));
#16227=CARTESIAN_POINT('Ctrl Pts',(-3.54457538552076,2.16354326577609,4.85547253923908));
#16228=CARTESIAN_POINT('Ctrl Pts',(-3.75407113442107,2.22119506367479,4.84507958712252));
#16229=CARTESIAN_POINT('Ctrl Pts',(-3.80505455493103,2.34521910535256,4.83839123135824));
#16230=CARTESIAN_POINT('Ctrl Pts',(-3.80555825533459,2.40017991403412,4.83540747194623));
#16231=CARTESIAN_POINT('Origin',(-3.6,2.4,5.35459252805377));
#16232=CARTESIAN_POINT('',(-3.80552958623817,2.39981603086253,4.97540747194623));
#16233=CARTESIAN_POINT('',(-3.8054461347863,2.4001877030526,4.96959252805377));
#16234=CARTESIAN_POINT('',(-3.805475,2.40000000000001,5.35459252805377));
#16235=CARTESIAN_POINT('Ctrl Pts',(-3.80544613478631,2.4001877030526,4.96959252805377));
#16236=CARTESIAN_POINT('Ctrl Pts',(-3.8056000456266,2.41718968004276,4.9686707998386));
#16237=CARTESIAN_POINT('Ctrl Pts',(-3.79589308272504,2.50235240455911,4.96404447527116));
#16238=CARTESIAN_POINT('Ctrl Pts',(-3.67755429503925,2.63014996180817,4.95571355435145));
#16239=CARTESIAN_POINT('Ctrl Pts',(-3.44869918906956,2.58997825726379,4.94459976529464));
#16240=CARTESIAN_POINT('Ctrl Pts',(-3.35833143120733,2.37591729928569,4.93348597623784));
#16241=CARTESIAN_POINT('Ctrl Pts',(-3.48916565507154,2.18389951041786,4.92237218718103));
#16242=CARTESIAN_POINT('Ctrl Pts',(-3.72144781179447,2.18968095039579,4.91125839812423));
#16243=CARTESIAN_POINT('Ctrl Pts',(-3.80419976151153,2.32515687187029,4.90366517841514));
#16244=CARTESIAN_POINT('Ctrl Pts',(-3.80580670007452,2.39655859898363,4.89977655505832));
#16245=CARTESIAN_POINT('Ctrl Pts',(-3.8057933217542,2.39993826202139,4.89959252805377));
#16246=CARTESIAN_POINT('Ctrl Pts',(-3.80552958623817,2.39981603086253,4.97540747194623));
#16247=CARTESIAN_POINT('Ctrl Pts',(-3.80503092645118,2.45384921596595,4.97247512456653));
#16248=CARTESIAN_POINT('Ctrl Pts',(-3.75549941221135,2.57695439031686,4.96583818083456));
#16249=CARTESIAN_POINT('Ctrl Pts',(-3.54785414659174,2.63720135974049,4.9554966407503));
#16250=CARTESIAN_POINT('Ctrl Pts',(-3.37243277255298,2.48483414437987,4.94438285169351));
#16251=CARTESIAN_POINT('Ctrl Pts',(-3.40530626273826,2.25481727477052,4.9332690626367));
#16252=CARTESIAN_POINT('Ctrl Pts',(-3.61638513853951,2.15768779995451,4.9221552735799));
#16253=CARTESIAN_POINT('Ctrl Pts',(-3.78023981554385,2.2618608319249,4.91286807668307));
#16254=CARTESIAN_POINT('Ctrl Pts',(-3.80513037719409,2.36523705642733,4.90728547613852));
#16255=CARTESIAN_POINT('Ctrl Pts',(-3.80514216591096,2.40000781019071,4.90540747194623));
#16256=CARTESIAN_POINT('Origin',(-3.6,2.4,5.35459252805377));
#16257=CARTESIAN_POINT('',(-3.8057470998819,2.40010656251728,5.04540747194623));
#16258=CARTESIAN_POINT('',(-3.80515433183015,2.39994744458997,5.03959252805377));
#16259=CARTESIAN_POINT('',(-3.805475,2.40000000000001,5.35459252805377));
#16260=CARTESIAN_POINT('Ctrl Pts',(-3.80515433183015,2.39994744458997,5.03959252805377));
#16261=CARTESIAN_POINT('Ctrl Pts',(-3.80506840880667,2.4374802122161,5.03756504461887));
#16262=CARTESIAN_POINT('Ctrl Pts',(-3.77723759754696,2.54371107308321,5.03183296483171));
#16263=CARTESIAN_POINT('Ctrl Pts',(-3.60662102779949,2.64277527582587,5.02239628869227));
#16264=CARTESIAN_POINT('Ctrl Pts',(-3.39962169493761,2.53723049491962,5.01128249963547));
#16265=CARTESIAN_POINT('Ctrl Pts',(-3.3760308968172,2.30607708183528,5.00016871057867));
#16266=CARTESIAN_POINT('Ctrl Pts',(-3.55744155898554,2.16089238284251,4.98905492152186));
#16267=CARTESIAN_POINT('Ctrl Pts',(-3.75953036163254,2.22845546798632,4.97886286068023));
#16268=CARTESIAN_POINT('Ctrl Pts',(-3.80498144946327,2.34885558664921,4.97237539619086));
#16269=CARTESIAN_POINT('Ctrl Pts',(-3.80544613478631,2.4001877030526,4.96959252805377));
#16270=CARTESIAN_POINT('Ctrl Pts',(-3.8057470998819,2.40010656251728,5.04540747194623));
#16271=CARTESIAN_POINT('Ctrl Pts',(-3.80578578291066,2.40623506936011,5.04507396569907));
#16272=CARTESIAN_POINT('Ctrl Pts',(-3.80275767503742,2.48040043607423,5.04103586309964));
#16273=CARTESIAN_POINT('Ctrl Pts',(-3.71288602216703,2.61503584063672,5.03329316414794));
#16274=CARTESIAN_POINT('Ctrl Pts',(-3.48055937550073,2.61146539619723,5.02217937509113));
#16275=CARTESIAN_POINT('Ctrl Pts',(-3.35755806712823,2.4143382523336,5.01106558603433));
#16276=CARTESIAN_POINT('Ctrl Pts',(-3.45646661930996,2.20408715554039,4.99995179697752));
#16277=CARTESIAN_POINT('Ctrl Pts',(-3.68675289766315,2.17315730107164,4.98883800792072));
#16278=CARTESIAN_POINT('Ctrl Pts',(-3.79782383296962,2.3032367743191,4.98065656624362));
#16279=CARTESIAN_POINT('Ctrl Pts',(-3.80566091089323,2.38558610982074,4.97617972091879));
#16280=CARTESIAN_POINT('Ctrl Pts',(-3.80552958623817,2.39981603086253,4.97540747194623));
#16281=CARTESIAN_POINT('Origin',(-3.6,2.4,5.35459252805377));
#16282=CARTESIAN_POINT('',(-3.80520911606596,2.40011619915578,5.11540747194623));
#16283=CARTESIAN_POINT('',(-3.80563879690963,2.399839625535,5.10959252805377));
#16284=CARTESIAN_POINT('',(-3.805475,2.40000000000001,5.35459252805377));
#16285=CARTESIAN_POINT('Ctrl Pts',(-3.80563879690963,2.399839625535,5.10959252805377));
#16286=CARTESIAN_POINT('Ctrl Pts',(-3.805144032728,2.45749534173516,5.10645928939914));
#16287=CARTESIAN_POINT('Ctrl Pts',(-3.74979515516761,2.58415303951777,5.09962145439226));
#16288=CARTESIAN_POINT('Ctrl Pts',(-3.53510505788101,2.63403473315196,5.0890790230331));
#16289=CARTESIAN_POINT('Ctrl Pts',(-3.36817873292179,2.47240567046266,5.07796523397629));
#16290=CARTESIAN_POINT('Ctrl Pts',(-3.41344102170209,2.24450262655374,5.06685144491949));
#16291=CARTESIAN_POINT('Ctrl Pts',(-3.6294628695539,2.15892821683407,5.05573765586269));
#16292=CARTESIAN_POINT('Ctrl Pts',(-3.78402795283848,2.2693666686934,5.04665135024078));
#16293=CARTESIAN_POINT('Ctrl Pts',(-3.80522540644911,2.36890073499569,5.04126964097114));
#16294=CARTESIAN_POINT('Ctrl Pts',(-3.80515433183015,2.39994744458997,5.03959252805377));
#16295=CARTESIAN_POINT('Ctrl Pts',(-3.80520911606596,2.40011619915578,5.11540747194623));
#16296=CARTESIAN_POINT('Ctrl Pts',(-3.80534689450199,2.42674223668704,5.11396821047934));
#16297=CARTESIAN_POINT('Ctrl Pts',(-3.7881600578547,2.52173200460476,5.10882435266019));
#16298=CARTESIAN_POINT('Ctrl Pts',(-3.64483147349944,2.63869087951471,5.09997589848877));
#16299=CARTESIAN_POINT('Ctrl Pts',(-3.42377646220466,2.56711959422357,5.08886210943196));
#16300=CARTESIAN_POINT('Ctrl Pts',(-3.36401957377094,2.34258029572384,5.07774832037515));
#16301=CARTESIAN_POINT('Ctrl Pts',(-3.52025888482579,2.17059867951396,5.06663453131835));
#16302=CARTESIAN_POINT('Ctrl Pts',(-3.7426071061349,2.20745024082863,5.05585424850871));
#16303=CARTESIAN_POINT('Ctrl Pts',(-3.80535609078813,2.33815945072363,5.04877856205134));
#16304=CARTESIAN_POINT('Ctrl Pts',(-3.8057470998819,2.40010656251728,5.04540747194623));
#16305=CARTESIAN_POINT('Origin',(-3.6,2.4,5.35459252805377));
#16306=CARTESIAN_POINT('',(-3.80526708520764,2.39977040928181,5.18540747194623));
#16307=CARTESIAN_POINT('',(-3.80565732826014,2.40014993187889,5.17959252805377));
#16308=CARTESIAN_POINT('',(-3.805475,2.40000000000001,5.35459252805377));
#16309=CARTESIAN_POINT('',(-3.65301702171886,2.20148256743283,5.2));
#16310=CARTESIAN_POINT('Ctrl Pts',(-3.65301702171886,2.20148256743283,5.2));
#16311=CARTESIAN_POINT('Ctrl Pts',(-3.71902879097456,2.21911198848201,5.19629540364773));
#16312=CARTESIAN_POINT('Ctrl Pts',(-3.79249439061758,2.28872811842027,5.19143122762981));
#16313=CARTESIAN_POINT('Ctrl Pts',(-3.80542873353734,2.378346888084,5.18656705161189));
#16314=CARTESIAN_POINT('Ctrl Pts',(-3.80526708520764,2.39977040928181,5.18540747194623));
#16315=CARTESIAN_POINT('',(-3.54686846753247,2.20112677390461,5.2));
#16316=CARTESIAN_POINT('Origin',(-3.6,2.4,5.2));
#16317=CARTESIAN_POINT('Ctrl Pts',(-3.54686839490754,2.2011265482535,5.2));
#16318=CARTESIAN_POINT('Ctrl Pts',(-3.61132828593009,2.18399467910883,5.19636770818144));
#16319=CARTESIAN_POINT('Ctrl Pts',(-3.74930829171963,2.21593295369214,5.1895652175327));
#16320=CARTESIAN_POINT('Ctrl Pts',(-3.80517196370246,2.34184094054235,5.18276272688396));
#16321=CARTESIAN_POINT('Ctrl Pts',(-3.80565732826014,2.40014993187889,5.17959252805377));
#16322=CARTESIAN_POINT('Origin',(-3.,1.8,5.2));
#16323=CARTESIAN_POINT('',(-3.,2.,0.8));
#16324=CARTESIAN_POINT('',(-3.2,1.8,0.8));
#16325=CARTESIAN_POINT('Origin',(-3.,1.8,0.8));
#16326=CARTESIAN_POINT('',(-3.,2.,5.2));
#16327=CARTESIAN_POINT('',(-3.,2.,5.2));
#16328=CARTESIAN_POINT('',(-3.2,1.8,5.2));
#16329=CARTESIAN_POINT('Origin',(-3.,1.8,5.2));
#16330=CARTESIAN_POINT('',(-3.2,1.8,5.2));
#16331=CARTESIAN_POINT('Origin',(-3.2,2.,5.2));
#16332=CARTESIAN_POINT('',(3.,2.,0.8));
#16333=CARTESIAN_POINT('',(3.2,2.,0.8));
#16334=CARTESIAN_POINT('',(3.,2.,5.2));
#16335=CARTESIAN_POINT('',(3.,2.,5.2));
#16336=CARTESIAN_POINT('',(-1.6,2.,5.2));
#16337=CARTESIAN_POINT('Origin',(3.,1.8,5.2));
#16338=CARTESIAN_POINT('',(3.2,1.8,0.8));
#16339=CARTESIAN_POINT('Origin',(3.,1.8,0.8));
#16340=CARTESIAN_POINT('',(3.2,1.8,5.2));
#16341=CARTESIAN_POINT('',(3.2,1.8,5.2));
#16342=CARTESIAN_POINT('Origin',(3.,1.8,5.2));
#16343=CARTESIAN_POINT('Origin',(3.2,2.,5.2));
#16344=CARTESIAN_POINT('',(3.2,-1.8,0.8));
#16345=CARTESIAN_POINT('',(3.2,-2.,0.8));
#16346=CARTESIAN_POINT('',(3.2,-1.8,5.2));
#16347=CARTESIAN_POINT('',(3.2,-1.8,5.2));
#16348=CARTESIAN_POINT('',(3.2,1.,5.2));
#16349=CARTESIAN_POINT('Origin',(-3.,-1.8,5.2));
#16350=CARTESIAN_POINT('',(-3.2,-1.8,0.8));
#16351=CARTESIAN_POINT('',(-3.,-2.,0.8));
#16352=CARTESIAN_POINT('Origin',(-3.,-1.8,0.8));
#16353=CARTESIAN_POINT('',(-3.2,-1.8,5.2));
#16354=CARTESIAN_POINT('',(-3.2,-1.8,5.2));
#16355=CARTESIAN_POINT('',(-3.,-2.,5.2));
#16356=CARTESIAN_POINT('Origin',(-3.,-1.8,5.2));
#16357=CARTESIAN_POINT('',(-3.,-2.,5.2));
#16358=CARTESIAN_POINT('Origin',(0.,0.,0.8));
#16359=CARTESIAN_POINT('',(-3.2,2.,0.8));
#16360=CARTESIAN_POINT('',(3.,-2.,0.8));
#16361=CARTESIAN_POINT('',(-3.2,-2.,0.8));
#16362=CARTESIAN_POINT('Origin',(3.,-1.8,0.8));
#16363=CARTESIAN_POINT('',(-0.8,-9.79717439317883E-17,0.8));
#16364=CARTESIAN_POINT('Origin',(0.,0.,0.8));
#16365=CARTESIAN_POINT('',(2.65,1.,0.8));
#16366=CARTESIAN_POINT('Origin',(2.4,1.,0.8));
#16367=CARTESIAN_POINT('',(-2.15,1.,0.8));
#16368=CARTESIAN_POINT('Origin',(-2.4,1.,0.8));
#16369=CARTESIAN_POINT('Origin',(3.2,-2.,5.2));
#16370=CARTESIAN_POINT('',(3.,-2.,5.2));
#16371=CARTESIAN_POINT('',(1.6,-2.,5.2));
#16372=CARTESIAN_POINT('',(3.,-2.,5.2));
#16373=CARTESIAN_POINT('',(7.34788079488412E-17,-2.,2.8));
#16374=CARTESIAN_POINT('Origin',(0.,-2.,2.2));
#16375=CARTESIAN_POINT('Origin',(3.,-1.8,5.2));
#16376=CARTESIAN_POINT('Origin',(3.,-1.8,5.2));
#16377=CARTESIAN_POINT('Origin',(0.,-2.4,2.2));
#16378=CARTESIAN_POINT('',(7.34788079488412E-17,-2.8,2.8));
#16379=CARTESIAN_POINT('Origin',(0.,-2.8,2.2));
#16380=CARTESIAN_POINT('',(7.34788079488412E-17,-2.4,2.8));
#16381=CARTESIAN_POINT('Origin',(-2.4,1.,0.4));
#16382=CARTESIAN_POINT('',(-2.,1.,0.4));
#16383=CARTESIAN_POINT('Origin',(-2.4,1.,0.4));
#16384=CARTESIAN_POINT('',(-2.15,1.,0.4));
#16385=CARTESIAN_POINT('Origin',(-2.4,1.,0.4));
#16386=CARTESIAN_POINT('Origin',(-2.4,1.,0.2));
#16387=CARTESIAN_POINT('',(-2.,1.,0.));
#16388=CARTESIAN_POINT('Origin',(-2.4,1.,0.));
#16389=CARTESIAN_POINT('',(-2.,1.,0.2));
#16390=CARTESIAN_POINT('Origin',(-2.4,1.,0.4));
#16391=CARTESIAN_POINT('',(-2.15,1.,0.4));
#16392=CARTESIAN_POINT('Origin',(2.4,1.,0.4));
#16393=CARTESIAN_POINT('',(2.8,1.,0.4));
#16394=CARTESIAN_POINT('Origin',(2.4,1.,0.4));
#16395=CARTESIAN_POINT('',(2.65,1.,0.4));
#16396=CARTESIAN_POINT('Origin',(2.4,1.,0.4));
#16397=CARTESIAN_POINT('Origin',(2.4,1.,0.2));
#16398=CARTESIAN_POINT('',(2.8,1.,0.));
#16399=CARTESIAN_POINT('Origin',(2.4,1.,0.));
#16400=CARTESIAN_POINT('',(2.8,1.,0.2));
#16401=CARTESIAN_POINT('Origin',(2.4,1.,0.4));
#16402=CARTESIAN_POINT('',(2.65,1.,0.4));
#16403=CARTESIAN_POINT('Origin',(-3.6,2.4,4.3));
#16404=CARTESIAN_POINT('Ctrl Pts',(-3.76351293272515,2.3680769545372,4.3));
#16405=CARTESIAN_POINT('Ctrl Pts',(-3.76286871316717,2.35978063266222,4.3));
#16406=CARTESIAN_POINT('Ctrl Pts',(-3.76155560899202,2.35157023575845,4.3));
#16407=CARTESIAN_POINT('Ctrl Pts',(-3.75963220387653,2.34349709858594,4.3));
#16408=CARTESIAN_POINT('Ctrl Pts',(-3.75857027766629,2.33903985975814,4.3));
#16409=CARTESIAN_POINT('Ctrl Pts',(-3.75732203034493,2.33462439532847,4.3));
#16410=CARTESIAN_POINT('Ctrl Pts',(-3.75589532649161,2.33025917511629,4.3));
#16411=CARTESIAN_POINT('Ctrl Pts',(-3.75435560971578,2.32554817445892,4.3));
#16412=CARTESIAN_POINT('Ctrl Pts',(-3.75261043848503,2.32090359735875,4.3));
#16413=CARTESIAN_POINT('Ctrl Pts',(-3.75067344213558,2.31634215529567,4.3));
#16414=CARTESIAN_POINT('Ctrl Pts',(-3.74745267041618,2.30875754441053,4.3));
#16415=CARTESIAN_POINT('Ctrl Pts',(-3.74370039609997,2.30139711771457,4.3));
#16416=CARTESIAN_POINT('Ctrl Pts',(-3.73945961576596,2.29430909563144,4.3));
#16417=CARTESIAN_POINT('Ctrl Pts',(-3.73760645031824,2.29121172284092,4.3));
#16418=CARTESIAN_POINT('Ctrl Pts',(-3.73566013813008,2.28816728583911,4.3));
#16419=CARTESIAN_POINT('Ctrl Pts',(-3.73363014813367,2.28518827452246,4.3));
#16420=CARTESIAN_POINT('Ctrl Pts',(-3.72675415090804,2.27509774521709,4.3));
#16421=CARTESIAN_POINT('Ctrl Pts',(-3.71890632139719,2.26572975853371,4.3));
#16422=CARTESIAN_POINT('Ctrl Pts',(-3.71022045861654,2.25723279915054,4.3));
#16423=CARTESIAN_POINT('Ctrl Pts',(-3.7059906475113,2.25309497956169,4.3));
#16424=CARTESIAN_POINT('Ctrl Pts',(-3.70156132140551,2.2491639079058,4.3));
#16425=CARTESIAN_POINT('Ctrl Pts',(-3.6969439956845,2.24545878490313,4.3));
#16426=CARTESIAN_POINT('Ctrl Pts',(-3.69303802929494,2.24232448448942,4.3));
#16427=CARTESIAN_POINT('Ctrl Pts',(-3.68899297342194,2.23934940616711,4.3));
#16428=CARTESIAN_POINT('Ctrl Pts',(-3.68484121061819,2.23656266363051,4.3));
#16429=CARTESIAN_POINT('Ctrl Pts',(-3.67976592507208,2.23315603498015,4.3));
#16430=CARTESIAN_POINT('Ctrl Pts',(-3.6745257104219,2.23002554470273,4.3));
#16431=CARTESIAN_POINT('Ctrl Pts',(-3.66913582629221,2.22718930926681,4.3));
#16432=CARTESIAN_POINT('Ctrl Pts',(-3.6615627323528,2.22320423706977,4.3));
#16433=CARTESIAN_POINT('Ctrl Pts',(-3.65369447955584,2.21979946771843,4.3));
#16434=CARTESIAN_POINT('Ctrl Pts',(-3.64559786041243,2.21695927257373,4.3));
#16435=CARTESIAN_POINT('Ctrl Pts',(-3.6396877011334,2.21488606085518,4.3));
#16436=CARTESIAN_POINT('Ctrl Pts',(-3.63365563048822,2.21311388420288,4.3));
#16437=CARTESIAN_POINT('Ctrl Pts',(-3.62752539225901,2.21164027047228,4.3));
#16438=CARTESIAN_POINT('Ctrl Pts',(-3.62399744472375,2.21079220686783,4.3));
#16439=CARTESIAN_POINT('Ctrl Pts',(-3.62044147481098,2.2100443281221,4.3));
#16440=CARTESIAN_POINT('Ctrl Pts',(-3.61687028704666,2.20939689951074,4.3));
#16441=CARTESIAN_POINT('Ctrl Pts',(-3.605353381675,2.20730897399576,4.3));
#16442=CARTESIAN_POINT('Ctrl Pts',(-3.59365536798806,2.20625732317521,4.3));
#16443=CARTESIAN_POINT('Ctrl Pts',(-3.58193303067035,2.20620865478203,4.3));
#16444=CARTESIAN_POINT('Ctrl Pts',(-3.57526869322992,2.20618098601718,4.3));
#16445=CARTESIAN_POINT('Ctrl Pts',(-3.56859610554753,2.20647808326505,4.3));
#16446=CARTESIAN_POINT('Ctrl Pts',(-3.5619424077193,2.20709864598645,4.3));
#16447=CARTESIAN_POINT('Ctrl Pts',(-3.55784552037318,2.20748074562885,4.3));
#16448=CARTESIAN_POINT('Ctrl Pts',(-3.55375372321261,2.20798587206127,4.3));
#16449=CARTESIAN_POINT('Ctrl Pts',(-3.54967985340644,2.20861337807665,4.3));
#16450=CARTESIAN_POINT('Ctrl Pts',(-3.53642392777045,2.21065521384261,4.3));
#16451=CARTESIAN_POINT('Ctrl Pts',(-3.52344437883893,2.21397442298982,4.3));
#16452=CARTESIAN_POINT('Ctrl Pts',(-3.51095539964347,2.2185383760968,4.3));
#16453=CARTESIAN_POINT('Ctrl Pts',(-3.50062245090115,2.22231443279277,4.3));
#16454=CARTESIAN_POINT('Ctrl Pts',(-3.49062431451358,2.22694342333832,4.3));
#16455=CARTESIAN_POINT('Ctrl Pts',(-3.48108410337466,2.23243384161104,4.3));
#16456=CARTESIAN_POINT('Ctrl Pts',(-3.47992982403391,2.23309813260964,4.3));
#16457=CARTESIAN_POINT('Ctrl Pts',(-3.47878225959784,2.23377506397182,4.3));
#16458=CARTESIAN_POINT('Ctrl Pts',(-3.47764149019701,2.2344644673347,4.3));
#16459=CARTESIAN_POINT('Ctrl Pts',(-3.41173724903364,2.31767678198965,4.3));
#16460=CARTESIAN_POINT('Ctrl Pts',(-3.40908132667977,2.32572936887695,4.3));
#16461=CARTESIAN_POINT('Ctrl Pts',(-3.40697195743913,2.3339396046188,4.3));
#16462=CARTESIAN_POINT('Ctrl Pts',(-3.40539675516275,2.34225613248928,4.3));
#16463=CARTESIAN_POINT('Ctrl Pts',(-3.40421042715,2.34851953759571,4.3));
#16464=CARTESIAN_POINT('Ctrl Pts',(-3.40332726918042,2.35484328996956,4.3));
#16465=CARTESIAN_POINT('Ctrl Pts',(-3.40274510142185,2.36120518228067,4.3));
#16466=CARTESIAN_POINT('Ctrl Pts',(-3.40230911384944,2.36596962679656,4.3));
#16467=CARTESIAN_POINT('Ctrl Pts',(-3.40204239822336,2.37075409356134,4.3));
#16468=CARTESIAN_POINT('Ctrl Pts',(-3.40194406709946,2.37553699140669,4.3));
#16469=CARTESIAN_POINT('Ctrl Pts',(-3.40173837831389,2.38554184450123,4.3));
#16470=CARTESIAN_POINT('Ctrl Pts',(-3.40226689742789,2.39555478383888,4.3));
#16471=CARTESIAN_POINT('Ctrl Pts',(-3.40352192589958,2.40548747856692,4.3));
#16472=CARTESIAN_POINT('Ctrl Pts',(-3.40417748512669,2.41067578291694,4.3));
#16473=CARTESIAN_POINT('Ctrl Pts',(-3.40503255607762,2.41584510393915,4.3));
#16474=CARTESIAN_POINT('Ctrl Pts',(-3.40608151604784,2.42095776789691,4.3));
#16475=CARTESIAN_POINT('Ctrl Pts',(-3.40864845689543,2.4334691184973,4.3));
#16476=CARTESIAN_POINT('Ctrl Pts',(-3.41237570095201,2.44567367466126,4.3));
#16477=CARTESIAN_POINT('Ctrl Pts',(-3.41724958122609,2.45738288213971,4.3));
#16478=CARTESIAN_POINT('Ctrl Pts',(-3.41948715125122,2.46275851104282,4.3));
#16479=CARTESIAN_POINT('Ctrl Pts',(-3.42196701213329,2.46802938689262,4.3));
#16480=CARTESIAN_POINT('Ctrl Pts',(-3.4246907645117,2.47317480637784,4.3));
#16481=CARTESIAN_POINT('Ctrl Pts',(-3.42647139059006,2.47653857328711,4.3));
#16482=CARTESIAN_POINT('Ctrl Pts',(-3.42835735887431,2.47985042338477,4.3));
#16483=CARTESIAN_POINT('Ctrl Pts',(-3.43034607421528,2.48309853180527,4.3));
#16484=CARTESIAN_POINT('Ctrl Pts',(-3.4346184872232,2.49007653432835,4.3));
#16485=CARTESIAN_POINT('Ctrl Pts',(-3.43934735204432,2.49673388406761,4.3));
#16486=CARTESIAN_POINT('Ctrl Pts',(-3.44453054699271,2.50301823813816,4.3));
#16487=CARTESIAN_POINT('Ctrl Pts',(-3.45023589251222,2.50993567259632,4.3));
#16488=CARTESIAN_POINT('Ctrl Pts',(-3.45649190823175,2.51640147868906,4.3));
#16489=CARTESIAN_POINT('Ctrl Pts',(-3.46322632730094,2.52238265672963,4.3));
#16490=CARTESIAN_POINT('Ctrl Pts',(-3.46747028515846,2.52615193026038,4.3));
#16491=CARTESIAN_POINT('Ctrl Pts',(-3.47190440586361,2.52972849539073,4.3));
#16492=CARTESIAN_POINT('Ctrl Pts',(-3.4765114687556,2.53310132051434,4.3));
#16493=CARTESIAN_POINT('Ctrl Pts',(-3.47932494356125,2.53516106198772,4.3));
#16494=CARTESIAN_POINT('Ctrl Pts',(-3.48219950761294,2.53714209816472,4.3));
#16495=CARTESIAN_POINT('Ctrl Pts',(-3.48512412807744,2.53903826687632,4.3));
#16496=CARTESIAN_POINT('Ctrl Pts',(-3.49373597317477,2.5446217302422,4.3));
#16497=CARTESIAN_POINT('Ctrl Pts',(-3.50279826970664,2.54948377957132,4.3));
#16498=CARTESIAN_POINT('Ctrl Pts',(-3.51220207894208,2.55357333967367,4.3));
#16499=CARTESIAN_POINT('Ctrl Pts',(-3.5210279439966,2.5574115614721,4.3));
#16500=CARTESIAN_POINT('Ctrl Pts',(-3.53015530415702,2.56056927246177,4.3));
#16501=CARTESIAN_POINT('Ctrl Pts',(-3.53949459164804,2.56298239916129,4.3));
#16502=CARTESIAN_POINT('Ctrl Pts',(-3.54298202528158,2.5638834977967,4.3));
#16503=CARTESIAN_POINT('Ctrl Pts',(-3.54649047145145,2.5646782882288,4.3));
#16504=CARTESIAN_POINT('Ctrl Pts',(-3.55001192980026,2.5653638227639,4.3));
#16505=CARTESIAN_POINT('Ctrl Pts',(-3.56109314401874,2.567521041247,4.3));
#16506=CARTESIAN_POINT('Ctrl Pts',(-3.57231422450356,2.56860269457927,4.3));
#16507=CARTESIAN_POINT('Ctrl Pts',(-3.58352456323646,2.56851224856759,4.3));
#16508=CARTESIAN_POINT('Ctrl Pts',(-3.58970650036672,2.56846237214805,4.3));
#16509=CARTESIAN_POINT('Ctrl Pts',(-3.59588506606642,2.56805522595141,4.3));
#16510=CARTESIAN_POINT('Ctrl Pts',(-3.60203269728429,2.56726809931874,4.3));
#16511=CARTESIAN_POINT('Ctrl Pts',(-3.60310836212971,2.56713037400346,4.3));
#16512=CARTESIAN_POINT('Ctrl Pts',(-3.60418307356748,2.56698100334876,4.3));
#16513=CARTESIAN_POINT('Ctrl Pts',(-3.60525667864057,2.56682005840211,4.3));
#16514=CARTESIAN_POINT('Origin',(-3.6,2.4,5.35459252805377));
#16515=CARTESIAN_POINT('Ctrl Pts',(-3.80565732826014,2.40014993187889,5.17959252805377));
#16516=CARTESIAN_POINT('Ctrl Pts',(-3.80573914572043,2.40997902530624,5.17905813053169));
#16517=CARTESIAN_POINT('Ctrl Pts',(-3.80062938236564,2.48786313470717,5.17481913665734));
#16518=CARTESIAN_POINT('Ctrl Pts',(-3.70109553522054,2.62084298334156,5.16687554643073));
#16519=CARTESIAN_POINT('Ctrl Pts',(-3.46929950811782,2.60468896536386,5.15576175737392));
#16520=CARTESIAN_POINT('Ctrl Pts',(-3.35713783891219,2.401213058351,5.14464796831712));
#16521=CARTESIAN_POINT('Ctrl Pts',(-3.46726930372222,2.19661072251331,5.13353417926031));
#16522=CARTESIAN_POINT('Ctrl Pts',(-3.69889135748228,2.17818094124235,5.12242039020352));
#16523=CARTESIAN_POINT('Ctrl Pts',(-3.80021577778504,2.31073764355723,5.11443983980133));
#16524=CARTESIAN_POINT('Ctrl Pts',(-3.80572901899447,2.38932589169745,5.11016388575141));
#16525=CARTESIAN_POINT('Ctrl Pts',(-3.80563879690963,2.399839625535,5.10959252805377));
#16526=CARTESIAN_POINT('Ctrl Pts',(-3.80526708520764,2.39977040928181,5.18540747194623));
#16527=CARTESIAN_POINT('Ctrl Pts',(-3.80491230346332,2.4467902221928,5.18286245525962));
#16528=CARTESIAN_POINT('Ctrl Pts',(-3.76565540874154,2.56295294620881,5.17661284222074));
#16529=CARTESIAN_POINT('Ctrl Pts',(-3.57278676575927,2.64128531597693,5.16665863282959));
#16530=CARTESIAN_POINT('Ctrl Pts',(-3.38252462806861,2.5080933346037,5.15554484377278));
#16531=CARTESIAN_POINT('Ctrl Pts',(-3.39123766596766,2.27586209704876,5.14443105471597));
#16532=CARTESIAN_POINT('Ctrl Pts',(-3.59107442724388,2.15730569128375,5.13331726565918));
#16533=CARTESIAN_POINT('Ctrl Pts',(-3.77212564275939,2.247453977085,5.12364273806926));
#16534=CARTESIAN_POINT('Ctrl Pts',(-3.80499225880634,2.35820797534334,5.11767280683161));
#16535=CARTESIAN_POINT('Ctrl Pts',(-3.80520911606596,2.40011619915578,5.11540747194623));
#16536=CARTESIAN_POINT('Ctrl Pts',(-3.47309291201476,2.50793586530485,5.2));
#16537=CARTESIAN_POINT('Ctrl Pts',(-3.43720166889934,2.46573623930395,5.19629540364773));
#16538=CARTESIAN_POINT('Ctrl Pts',(-3.41147910372774,2.34341327692754,5.1888862109432));
#16539=CARTESIAN_POINT('Ctrl Pts',(-3.54548749138621,2.21065847912018,5.17777242188639));
#16540=CARTESIAN_POINT('Ctrl Pts',(-3.72942273074541,2.25164328799446,5.16665863282959));
#16541=CARTESIAN_POINT('Ctrl Pts',(-3.79487861203899,2.42820978532064,5.15554484377278));
#16542=CARTESIAN_POINT('Ctrl Pts',(-3.68196868800459,2.57906042596279,5.14443105471598));
#16543=CARTESIAN_POINT('Ctrl Pts',(-3.49402748778406,2.56596267978888,5.13331726565918));
#16544=CARTESIAN_POINT('Ctrl Pts',(-3.40308633148933,2.40098355284719,5.12220347660236));
#16545=CARTESIAN_POINT('Ctrl Pts',(-3.49238138946403,2.23509111264493,5.11108968754557));
#16546=CARTESIAN_POINT('Ctrl Pts',(-3.68018153136171,2.22014816795705,5.09997589848877));
#16547=CARTESIAN_POINT('Ctrl Pts',(-3.79459033398193,2.36982238810866,5.08886210943195));
#16548=CARTESIAN_POINT('Ctrl Pts',(-3.73088853410035,2.54712014517116,5.07774832037516));
#16549=CARTESIAN_POINT('Ctrl Pts',(-3.54738290615879,2.58975635256414,5.06663453131835));
#16550=CARTESIAN_POINT('Ctrl Pts',(-3.41203833510047,2.45870682418337,5.05552074226154));
#16551=CARTESIAN_POINT('Ctrl Pts',(-3.44873719048823,2.27392207121964,5.04440695320474));
#16552=CARTESIAN_POINT('Ctrl Pts',(-3.62388861938279,2.20453797748901,5.03329316414794));
#16553=CARTESIAN_POINT('Ctrl Pts',(-3.77717451978384,2.31406243911007,5.02217937509113));
#16554=CARTESIAN_POINT('Ctrl Pts',(-3.76829057505717,2.5022465500548,5.01106558603433));
#16555=CARTESIAN_POINT('Ctrl Pts',(-3.60536835737386,2.5968432215724,4.99995179697752));
#16556=CARTESIAN_POINT('Ctrl Pts',(-3.43753242183529,2.51126706632734,4.98883800792072));
#16557=CARTESIAN_POINT('Ctrl Pts',(-3.41840490283366,2.32384690027379,4.97772421886392));
#16558=CARTESIAN_POINT('Ctrl Pts',(-3.56549343582914,2.20613053160512,4.96661042980711));
#16559=CARTESIAN_POINT('Ctrl Pts',(-3.74416621827519,2.26586508520319,4.95549664075031));
#16560=CARTESIAN_POINT('Ctrl Pts',(-3.79088202621085,2.44837484789993,4.9443828516935));
#16561=CARTESIAN_POINT('Ctrl Pts',(-3.66288135078982,2.58660656351012,4.9332690626367));
#16562=CARTESIAN_POINT('Ctrl Pts',(-3.47732466187608,2.55403517537485,4.9221552735799));
#16563=CARTESIAN_POINT('Ctrl Pts',(-3.40405410117601,2.38047364429248,4.91104148452309));
#16564=CARTESIAN_POINT('Ctrl Pts',(-3.51013504384922,2.2247848080575,4.89992769546628));
#16565=CARTESIAN_POINT('Ctrl Pts',(-3.69847040002413,2.22947242407076,4.88881390640949));
#16566=CARTESIAN_POINT('Ctrl Pts',(-3.79667468232717,2.39024586425236,4.87770011735267));
#16567=CARTESIAN_POINT('Ctrl Pts',(-3.7148603974533,2.55994737550017,4.86658632829588));
#16568=CARTESIAN_POINT('Ctrl Pts',(-3.52791308818505,2.58324724002758,4.85547253923907));
#16569=CARTESIAN_POINT('Ctrl Pts',(-3.40694774682213,2.43881882759193,4.84435875018226));
#16570=CARTESIAN_POINT('Ctrl Pts',(-3.46268532215442,2.25885910202633,4.83324496112546));
#16571=CARTESIAN_POINT('Ctrl Pts',(-3.64410857937311,2.20808724102248,4.82213117206866));
#16572=CARTESIAN_POINT('Ctrl Pts',(-3.78515875366629,2.33297530474957,4.81101738301185));
#16573=CARTESIAN_POINT('Ctrl Pts',(-3.75673102088563,2.51921183215107,4.79990359395505));
#16574=CARTESIAN_POINT('Ctrl Pts',(-3.58484560723768,2.59633241763059,4.78878980489824));
#16575=CARTESIAN_POINT('Ctrl Pts',(-3.42683118114759,2.49374771469177,4.77767601584145));
#16576=CARTESIAN_POINT('Ctrl Pts',(-3.42732013882109,2.30535466532418,4.76656222678463));
#16577=CARTESIAN_POINT('Ctrl Pts',(-3.58586493175446,2.20359156413646,4.75544843772784));
#16578=CARTESIAN_POINT('Ctrl Pts',(-3.75734771295555,2.28160333171781,4.74433464867102));
#16579=CARTESIAN_POINT('Ctrl Pts',(-3.784808348044,2.46798491248738,4.73322085961423));
#16580=CARTESIAN_POINT('Ctrl Pts',(-3.64311180629855,2.59213913185591,4.72210707055742));
#16581=CARTESIAN_POINT('Ctrl Pts',(-3.46195453932691,2.54042622483077,4.71099328150062));
#16582=CARTESIAN_POINT('Ctrl Pts',(-3.40715184805135,2.36017960167632,4.69987949244381));
#16583=CARTESIAN_POINT('Ctrl Pts',(-3.52886525730118,2.21638104070156,4.688765703387));
#16584=CARTESIAN_POINT('Ctrl Pts',(-3.7156891032661,2.24065099555331,4.67765191433021));
#16585=CARTESIAN_POINT('Ctrl Pts',(-3.79662140100789,2.41077490131571,4.6665381252734));
#16586=CARTESIAN_POINT('Ctrl Pts',(-3.69758390056881,2.57103641770819,4.65542433621659));
#16587=CARTESIAN_POINT('Ctrl Pts',(-3.50922674926239,2.57474636128738,4.64431054715979));
#16588=CARTESIAN_POINT('Ctrl Pts',(-3.40395538379481,2.41850897862188,4.63319675810298));
#16589=CARTESIAN_POINT('Ctrl Pts',(-3.47812587883694,2.24533011791732,4.62208296904618));
#16590=CARTESIAN_POINT('Ctrl Pts',(-3.6638491391263,2.21372235435953,4.61096917998938));
#16591=CARTESIAN_POINT('Ctrl Pts',(-3.79113055827457,2.35261663238717,4.59985539093257));
#16592=CARTESIAN_POINT('Ctrl Pts',(-3.74346800986679,2.53488144415775,4.58874160187577));
#16593=CARTESIAN_POINT('Ctrl Pts',(-3.56448756498879,2.59368774042515,4.57762781281897));
#16594=CARTESIAN_POINT('Ctrl Pts',(-3.41801205461748,2.475209451325,4.56651402376216));
#16595=CARTESIAN_POINT('Ctrl Pts',(-3.4381121745334,2.28789109846994,4.55540023470536));
#16596=CARTESIAN_POINT('Ctrl Pts',(-3.60639005704185,2.20318729463469,4.54428644564855));
#16597=CARTESIAN_POINT('Ctrl Pts',(-3.76881904785141,2.29862839193225,4.53317265659175));
#16598=CARTESIAN_POINT('Ctrl Pts',(-3.77672604966501,2.48685607191854,4.52205886753494));
#16599=CARTESIAN_POINT('Ctrl Pts',(-3.62287369392911,2.59558340387831,4.51094507847814));
#16600=CARTESIAN_POINT('Ctrl Pts',(-3.44808478689753,2.52529102897173,4.49983128942133));
#16601=CARTESIAN_POINT('Ctrl Pts',(-3.41234559692803,2.34031835280842,4.48871750036453));
#16602=CARTESIAN_POINT('Ctrl Pts',(-3.54836861088932,2.20997296824294,4.47760371130773));
#16603=CARTESIAN_POINT('Ctrl Pts',(-3.73165041953522,2.2535614747159,4.46648992225092));
#16604=CARTESIAN_POINT('Ctrl Pts',(-3.79443110878254,2.431186836485,4.45537613319412));
#16605=CARTESIAN_POINT('Ctrl Pts',(-3.67924679391792,2.58026650835313,4.44426234413731));
#16606=CARTESIAN_POINT('Ctrl Pts',(-3.49152700036135,2.56434625038721,4.43314855508051));
#16607=CARTESIAN_POINT('Ctrl Pts',(-3.40309375251607,2.39799790627107,4.4220347660237));
#16608=CARTESIAN_POINT('Ctrl Pts',(-3.49489106815987,2.23348230018954,4.4109209769669));
#16609=CARTESIAN_POINT('Ctrl Pts',(-3.68289569684173,2.22138183485646,4.3998071879101));
#16610=CARTESIAN_POINT('Ctrl Pts',(-3.79502512287648,2.37277339930001,4.38869339885329));
#16611=CARTESIAN_POINT('Ctrl Pts',(-3.72864550427982,2.54908418322982,4.37757960979649));
#16612=CARTESIAN_POINT('Ctrl Pts',(-3.54451587329345,2.58893972093235,4.36646582073968));
#16613=CARTESIAN_POINT('Ctrl Pts',(-3.41117013795305,2.4558501873037,4.35535203168288));
#16614=CARTESIAN_POINT('Ctrl Pts',(-3.45066522941702,2.27165316239582,4.34423824262608));
#16615=CARTESIAN_POINT('Ctrl Pts',(-3.62684269841689,2.20490778718547,4.33312445356927));
#16616=CARTESIAN_POINT('Ctrl Pts',(-3.77846161969435,2.31678392154068,4.32201066451247));
#16617=CARTESIAN_POINT('Ctrl Pts',(-3.76671077264337,2.50472571563538,4.31089687545566));
#16618=CARTESIAN_POINT('Ctrl Pts',(-3.6024119571336,2.59701778495161,4.29978308639886));
#16619=CARTESIAN_POINT('Ctrl Pts',(-3.43581014038123,2.50855356077874,4.28866929734205));
#16620=CARTESIAN_POINT('Ctrl Pts',(-3.42516046182893,2.38400982617005,4.28126010463752));
#16621=CARTESIAN_POINT('Ctrl Pts',(-3.44735576439472,2.33325198627315,4.27755550828525));
#16622=CARTESIAN_POINT('Ctrl Pts',(-3.46322193753412,2.51633123698097,5.20748149723825));
#16623=CARTESIAN_POINT('Ctrl Pts',(-3.42453903360215,2.47084927712496,5.20377690088598));
#16624=CARTESIAN_POINT('Ctrl Pts',(-3.39681573869656,2.33901189865735,5.19636770818145));
#16625=CARTESIAN_POINT('Ctrl Pts',(-3.54124744782407,2.19593128499412,5.18525391912464));
#16626=CARTESIAN_POINT('Ctrl Pts',(-3.73948937471845,2.24010393789599,5.17414013006784));
#16627=CARTESIAN_POINT('Ctrl Pts',(-3.81003648727512,2.43040397380471,5.16302634101103));
#16628=CARTESIAN_POINT('Ctrl Pts',(-3.68834430374324,2.59298794508905,5.15191255195423));
#16629=CARTESIAN_POINT('Ctrl Pts',(-3.48578482789531,2.57887144164721,5.14079876289743));
#16630=CARTESIAN_POINT('Ctrl Pts',(-3.38777016729695,2.40106005468179,5.12968497384062));
#16631=CARTESIAN_POINT('Ctrl Pts',(-3.48401069421676,2.22226431593439,5.11857118478382));
#16632=CARTESIAN_POINT('Ctrl Pts',(-3.68641814006856,2.20615909238548,5.10745739572702));
#16633=CARTESIAN_POINT('Ctrl Pts',(-3.80972578663008,2.36747513988482,5.0963436066702));
#16634=CARTESIAN_POINT('Ctrl Pts',(-3.74106918988897,2.55856331372564,5.0852298176134));
#16635=CARTESIAN_POINT('Ctrl Pts',(-3.5432902900662,2.60451581276008,5.0741160285566));
#16636=CARTESIAN_POINT('Ctrl Pts',(-3.39741846770758,2.46327310627647,5.06300223949979));
#16637=CARTESIAN_POINT('Ctrl Pts',(-3.43697180089285,2.26411558966434,5.05188845044299));
#16638=CARTESIAN_POINT('Ctrl Pts',(-3.62574670277316,2.18933472393736,5.04077466138618));
#16639=CARTESIAN_POINT('Ctrl Pts',(-3.79095535102953,2.30737812002324,5.02966087232938));
#16640=CARTESIAN_POINT('Ctrl Pts',(-3.78138040319912,2.51019940046172,5.01854708327258));
#16641=CARTESIAN_POINT('Ctrl Pts',(-3.60578591418241,2.61215390632356,5.00743329421578));
#16642=CARTESIAN_POINT('Ctrl Pts',(-3.42489551286939,2.51992154252476,4.99631950515897));
#16643=CARTESIAN_POINT('Ctrl Pts',(-3.40428023416151,2.31792362746096,4.98520571610217));
#16644=CARTESIAN_POINT('Ctrl Pts',(-3.56280947688127,2.19105114868425,4.97409192704536));
#16645=CARTESIAN_POINT('Ctrl Pts',(-3.75537962710962,2.25543192231258,4.96297813798856));
#16646=CARTESIAN_POINT('Ctrl Pts',(-3.80572904255528,2.45213749738394,4.95186434893175));
#16647=CARTESIAN_POINT('Ctrl Pts',(-3.6677723322063,2.60112102960948,4.94075055987495));
#16648=CARTESIAN_POINT('Ctrl Pts',(-3.46778283760724,2.56601620267116,4.92963677081815));
#16649=CARTESIAN_POINT('Ctrl Pts',(-3.38881321118645,2.37895486262355,4.91852298176134));
#16650=CARTESIAN_POINT('Ctrl Pts',(-3.50314524759,2.21115637551095,4.90740919270453));
#16651=CARTESIAN_POINT('Ctrl Pts',(-3.70612953728091,2.21620859951243,4.89629540364773));
#16652=CARTESIAN_POINT('Ctrl Pts',(-3.81197225790835,2.38948717672297,4.88518161459093));
#16653=CARTESIAN_POINT('Ctrl Pts',(-3.72379436694309,2.57238826029923,4.87406782553412));
#16654=CARTESIAN_POINT('Ctrl Pts',(-3.52230608799136,2.5975004142094,4.86295403647732));
#16655=CARTESIAN_POINT('Ctrl Pts',(-3.39193192780995,2.44183819918584,4.85184024742051));
#16656=CARTESIAN_POINT('Ctrl Pts',(-3.45200483375657,2.24788100597045,4.84072645836371));
#16657=CARTESIAN_POINT('Ctrl Pts',(-3.64753939374511,2.19316005313682,4.8296126693069));
#16658=CARTESIAN_POINT('Ctrl Pts',(-3.79956060750538,2.3277620493917,4.81849888025011));
#16659=CARTESIAN_POINT('Ctrl Pts',(-3.76892173404475,2.52848426107239,4.80738509119329));
#16660=CARTESIAN_POINT('Ctrl Pts',(-3.5836668817102,2.61160337148291,4.7962713021365));
#16661=CARTESIAN_POINT('Ctrl Pts',(-3.41336191777647,2.50103951622967,4.78515751307969));
#16662=CARTESIAN_POINT('Ctrl Pts',(-3.41388890712174,2.29799304590536,4.77404372402289));
#16663=CARTESIAN_POINT('Ctrl Pts',(-3.58476549042184,2.18831469750142,4.76292993496608));
#16664=CARTESIAN_POINT('Ctrl Pts',(-3.76958639310991,2.27239430714904,4.75181614590928));
#16665=CARTESIAN_POINT('Ctrl Pts',(-3.79918294694398,2.47327285461012,4.74070235685247));
#16666=CARTESIAN_POINT('Ctrl Pts',(-3.64646509055197,2.60708392727588,4.72958856779567));
#16667=CARTESIAN_POINT('Ctrl Pts',(-3.45121720982778,2.55134873281456,4.71847477873886));
#16668=CARTESIAN_POINT('Ctrl Pts',(-3.39215190425982,2.3570823267967,4.70736098968206));
#16669=CARTESIAN_POINT('Ctrl Pts',(-3.52333231788058,2.20209895378134,4.69624720062526));
#16670=CARTESIAN_POINT('Ctrl Pts',(-3.7246875304159,2.22825665272044,4.68513341156845));
#16671=CARTESIAN_POINT('Ctrl Pts',(-3.81191483230877,2.41161298512653,4.67401962251165));
#16672=CARTESIAN_POINT('Ctrl Pts',(-3.70517408491178,2.58433982054614,4.66290583345484));
#16673=CARTESIAN_POINT('Ctrl Pts',(-3.50216630483977,2.58833832766402,4.65179204439804));
#16674=CARTESIAN_POINT('Ctrl Pts',(-3.38870681545753,2.41994862756931,4.64067825534123));
#16675=CARTESIAN_POINT('Ctrl Pts',(-3.46864637411461,2.23329972242719,4.62956446628443));
#16676=CARTESIAN_POINT('Ctrl Pts',(-3.6688153961962,2.19923347185799,4.61845067722763));
#16677=CARTESIAN_POINT('Ctrl Pts',(-3.80599690571939,2.34893110134286,4.60733688817082));
#16678=CARTESIAN_POINT('Ctrl Pts',(-3.7546271112745,2.54537267293252,4.59622309911402));
#16679=CARTESIAN_POINT('Ctrl Pts',(-3.56172536828799,2.60875298834237,4.58510931005721));
#16680=CARTESIAN_POINT('Ctrl Pts',(-3.40385682977405,2.48105932611543,4.57399552100042));
#16681=CARTESIAN_POINT('Ctrl Pts',(-3.42552035937731,2.27917114339395,4.5628817319436));
#16682=CARTESIAN_POINT('Ctrl Pts',(-3.60688708278715,2.18787898346807,4.5517679428868));
#16683=CARTESIAN_POINT('Ctrl Pts',(-3.7819499811952,2.2907435954864,4.54065415383));
#16684=CARTESIAN_POINT('Ctrl Pts',(-3.79047199840596,2.49361183381496,4.52954036477319));
#16685=CARTESIAN_POINT('Ctrl Pts',(-3.62465283528865,2.61079609860775,4.51842657571639));
#16686=CARTESIAN_POINT('Ctrl Pts',(-3.43626865262511,2.53503630458453,4.50731278665958));
#16687=CARTESIAN_POINT('Ctrl Pts',(-3.39774962870189,2.33567624789731,4.49619899760278));
#16688=CARTESIAN_POINT('Ctrl Pts',(-3.54435266400721,2.19519245431826,4.48508520854598));
#16689=CARTESIAN_POINT('Ctrl Pts',(-3.74189033562052,2.24217132331451,4.47397141948917));
#16690=CARTESIAN_POINT('Ctrl Pts',(-3.80955417671754,2.43361258332043,4.46285763043237));
#16691=CARTESIAN_POINT('Ctrl Pts',(-3.68541069770656,2.59428783790942,4.45174384137556));
#16692=CARTESIAN_POINT('Ctrl Pts',(-3.48308984977921,2.57712928456848,4.44063005231877));
#16693=CARTESIAN_POINT('Ctrl Pts',(-3.38777816553941,2.39784218119362,4.42951626326195));
#16694=CARTESIAN_POINT('Ctrl Pts',(-3.48671557851344,2.22053036825651,4.41840247420515));
#16695=CARTESIAN_POINT('Ctrl Pts',(-3.68934341635898,2.20748871526871,4.40728868514834));
#16696=CARTESIAN_POINT('Ctrl Pts',(-3.81019439388853,2.37065568400947,4.39617489609154));
#16697=CARTESIAN_POINT('Ctrl Pts',(-3.73865169471375,2.56068011684939,4.38506110703474));
#16698=CARTESIAN_POINT('Ctrl Pts',(-3.54020025619518,2.60363566261151,4.37394731797793));
#16699=CARTESIAN_POINT('Ctrl Pts',(-3.3964827412202,2.46019427700244,4.36283352892113));
#16700=CARTESIAN_POINT('Ctrl Pts',(-3.43904980483436,2.26167020258818,4.35171973986432));
#16701=CARTESIAN_POINT('Ctrl Pts',(-3.62893055336078,2.18973329784341,4.34060595080752));
#16702=CARTESIAN_POINT('Ctrl Pts',(-3.79234256300291,2.3103112823848,4.32949216175072));
#16703=CARTESIAN_POINT('Ctrl Pts',(-3.77967772199614,2.5128713982991,4.31837837269391));
#16704=CARTESIAN_POINT('Ctrl Pts',(-3.60259956184262,2.61234204743659,4.30726458363711));
#16705=CARTESIAN_POINT('Ctrl Pts',(-3.42303927044789,2.51699697749597,4.2961507945803));
#16706=CARTESIAN_POINT('Ctrl Pts',(-3.41156124805062,2.38276609266137,4.28874160187577));
#16707=CARTESIAN_POINT('Ctrl Pts',(-3.43548292594103,2.32806025151199,4.2850370055235));
#16708=CARTESIAN_POINT('Ctrl Pts',(-3.45335096305347,2.52472660865709,5.2149629944765));
#16709=CARTESIAN_POINT('Ctrl Pts',(-3.41187639830495,2.47596231494597,5.21125839812423));
#16710=CARTESIAN_POINT('Ctrl Pts',(-3.38215237366538,2.33461052038716,5.20384920541969));
#16711=CARTESIAN_POINT('Ctrl Pts',(-3.53700740426192,2.18120409086806,5.19273541636289));
#16712=CARTESIAN_POINT('Ctrl Pts',(-3.7495560186915,2.22856458779753,5.18162162730609));
#16713=CARTESIAN_POINT('Ctrl Pts',(-3.82519436251124,2.43259816228878,5.17050783824928));
#16714=CARTESIAN_POINT('Ctrl Pts',(-3.69471991948189,2.60691546421531,5.15939404919248));
#16715=CARTESIAN_POINT('Ctrl Pts',(-3.47754216800657,2.59178020350553,5.14828026013568));
#16716=CARTESIAN_POINT('Ctrl Pts',(-3.37245400310457,2.4011365565164,5.13716647107886));
#16717=CARTESIAN_POINT('Ctrl Pts',(-3.47563999896949,2.20943751922385,5.12605268202207));
#16718=CARTESIAN_POINT('Ctrl Pts',(-3.69265474877542,2.19217001681392,5.11493889296526));
#16719=CARTESIAN_POINT('Ctrl Pts',(-3.82486123927823,2.36512789166097,5.10382510390846));
#16720=CARTESIAN_POINT('Ctrl Pts',(-3.75124984567759,2.57000648228012,5.09271131485165));
#16721=CARTESIAN_POINT('Ctrl Pts',(-3.53919767397361,2.61927527295602,5.08159752579485));
#16722=CARTESIAN_POINT('Ctrl Pts',(-3.38279860031468,2.46783938836956,5.07048373673804));
#16723=CARTESIAN_POINT('Ctrl Pts',(-3.42520641129747,2.25430910810904,5.05936994768124));
#16724=CARTESIAN_POINT('Ctrl Pts',(-3.62760478616353,2.17413147038572,5.04825615862444));
#16725=CARTESIAN_POINT('Ctrl Pts',(-3.80473618227523,2.30069380093641,5.03714236956763));
#16726=CARTESIAN_POINT('Ctrl Pts',(-3.79447023134107,2.51815225086865,5.02602858051083));
#16727=CARTESIAN_POINT('Ctrl Pts',(-3.60620347099095,2.62746459107471,5.01491479145402));
#16728=CARTESIAN_POINT('Ctrl Pts',(-3.4122586039035,2.52857601872219,5.00380100239722));
#16729=CARTESIAN_POINT('Ctrl Pts',(-3.39015556548935,2.31200035464812,4.99268721334042));
#16730=CARTESIAN_POINT('Ctrl Pts',(-3.56012551793341,2.17597176576338,4.98157342428361));
#16731=CARTESIAN_POINT('Ctrl Pts',(-3.76659303594405,2.24499875942197,4.9704596352268));
#16732=CARTESIAN_POINT('Ctrl Pts',(-3.82057605889971,2.45590014686796,4.95934584617));
#16733=CARTESIAN_POINT('Ctrl Pts',(-3.67266331362277,2.61563549570883,4.94823205711319));
#16734=CARTESIAN_POINT('Ctrl Pts',(-3.4582410133384,2.57799722996748,4.93711826805639));
#16735=CARTESIAN_POINT('Ctrl Pts',(-3.37357232119689,2.37743608095462,4.92600447899959));
#16736=CARTESIAN_POINT('Ctrl Pts',(-3.49615545133077,2.19752794296441,4.91489068994278));
#16737=CARTESIAN_POINT('Ctrl Pts',(-3.71378867453769,2.20294477495411,4.90377690088598));
#16738=CARTESIAN_POINT('Ctrl Pts',(-3.82726983348952,2.38872848919359,4.89266311182918));
#16739=CARTESIAN_POINT('Ctrl Pts',(-3.73272833643288,2.58482914509829,4.88154932277237));
#16740=CARTESIAN_POINT('Ctrl Pts',(-3.51669908779767,2.61175358839122,4.87043553371557));
#16741=CARTESIAN_POINT('Ctrl Pts',(-3.37691610879776,2.44485757077975,4.85932174465876));
#16742=CARTESIAN_POINT('Ctrl Pts',(-3.44132434535872,2.23690290991458,4.84820795560196));
#16743=CARTESIAN_POINT('Ctrl Pts',(-3.65097020811712,2.17823286525116,4.83709416654515));
#16744=CARTESIAN_POINT('Ctrl Pts',(-3.81396246134447,2.32254879403384,4.82598037748835));
#16745=CARTESIAN_POINT('Ctrl Pts',(-3.78111244720387,2.5377566899937,4.81486658843155));
#16746=CARTESIAN_POINT('Ctrl Pts',(-3.58248815618272,2.62687432533523,4.80375279937474));
#16747=CARTESIAN_POINT('Ctrl Pts',(-3.39989265440535,2.50833131776757,4.79263901031794));
#16748=CARTESIAN_POINT('Ctrl Pts',(-3.4004576754224,2.29063142648655,4.78152522126113));
#16749=CARTESIAN_POINT('Ctrl Pts',(-3.58366604908921,2.17303783086637,4.77041143220433));
#16750=CARTESIAN_POINT('Ctrl Pts',(-3.78182507326426,2.26318528258027,4.75929764314753));
#16751=CARTESIAN_POINT('Ctrl Pts',(-3.81355754584396,2.47856079673287,4.74818385409072));
#16752=CARTESIAN_POINT('Ctrl Pts',(-3.64981837480538,2.62202872269584,4.73707006503392));
#16753=CARTESIAN_POINT('Ctrl Pts',(-3.44047988032865,2.56227124079834,4.72595627597711));
#16754=CARTESIAN_POINT('Ctrl Pts',(-3.3771519604683,2.35398505191708,4.71484248692031));
#16755=CARTESIAN_POINT('Ctrl Pts',(-3.51779937845998,2.18781686686112,4.7037286978635));
#16756=CARTESIAN_POINT('Ctrl Pts',(-3.73368595756569,2.21586230988758,4.6926149088067));
#16757=CARTESIAN_POINT('Ctrl Pts',(-3.82720826360965,2.41245106893735,4.6815011197499));
#16758=CARTESIAN_POINT('Ctrl Pts',(-3.71276426925474,2.59764322338409,4.67038733069309));
#16759=CARTESIAN_POINT('Ctrl Pts',(-3.49510586041716,2.60193029404067,4.65927354163629));
#16760=CARTESIAN_POINT('Ctrl Pts',(-3.37345824712023,2.42138827651674,4.64815975257948));
#16761=CARTESIAN_POINT('Ctrl Pts',(-3.4591668693923,2.22126932693707,4.63704596352268));
#16762=CARTESIAN_POINT('Ctrl Pts',(-3.67378165326609,2.18474458935644,4.62593217446588));
#16763=CARTESIAN_POINT('Ctrl Pts',(-3.82086325316422,2.34524557029854,4.61481838540907));
#16764=CARTESIAN_POINT('Ctrl Pts',(-3.7657862126822,2.55586390170729,4.60370459635227));
#16765=CARTESIAN_POINT('Ctrl Pts',(-3.55896317158719,2.6238182362596,4.59259080729546));
#16766=CARTESIAN_POINT('Ctrl Pts',(-3.38970160493063,2.48690920090586,4.58147701823866));
#16767=CARTESIAN_POINT('Ctrl Pts',(-3.41292854422122,2.27045118831796,4.57036322918185));
#16768=CARTESIAN_POINT('Ctrl Pts',(-3.60738410853246,2.17257067230145,4.55924944012505));
#16769=CARTESIAN_POINT('Ctrl Pts',(-3.79508091453898,2.28285879904056,4.54813565106825));
#16770=CARTESIAN_POINT('Ctrl Pts',(-3.80421794714692,2.50036759571139,4.53702186201144));
#16771=CARTESIAN_POINT('Ctrl Pts',(-3.62643197664818,2.62600879333718,4.52590807295464));
#16772=CARTESIAN_POINT('Ctrl Pts',(-3.42445251835268,2.54478158019733,4.51479428389783));
#16773=CARTESIAN_POINT('Ctrl Pts',(-3.38315366047576,2.3310341429862,4.50368049484103));
#16774=CARTESIAN_POINT('Ctrl Pts',(-3.54033671712511,2.18041194039358,4.49256670578422));
#16775=CARTESIAN_POINT('Ctrl Pts',(-3.75213025170582,2.23078117191311,4.48145291672742));
#16776=CARTESIAN_POINT('Ctrl Pts',(-3.82467724465257,2.43603833015588,4.47033912767062));
#16777=CARTESIAN_POINT('Ctrl Pts',(-3.69157460149519,2.60830916746569,4.45922533861381));
#16778=CARTESIAN_POINT('Ctrl Pts',(-3.47465269919707,2.58991231874976,4.44811154955701));
#16779=CARTESIAN_POINT('Ctrl Pts',(-3.37246257856274,2.39768645611616,4.4369977605002));
#16780=CARTESIAN_POINT('Ctrl Pts',(-3.47854008886701,2.20757843632347,4.4258839714434));
#16781=CARTESIAN_POINT('Ctrl Pts',(-3.69579113587624,2.19359559568096,4.41477018238659));
#16782=CARTESIAN_POINT('Ctrl Pts',(-3.82536366490058,2.36853796871893,4.4036563933298));
#16783=CARTESIAN_POINT('Ctrl Pts',(-3.74865788514769,2.57227605046896,4.39254260427298));
#16784=CARTESIAN_POINT('Ctrl Pts',(-3.5358846390969,2.61833160429067,4.38142881521619));
#16785=CARTESIAN_POINT('Ctrl Pts',(-3.38179534448736,2.46453836670119,4.37031502615938));
#16786=CARTESIAN_POINT('Ctrl Pts',(-3.4274343802517,2.25168724278053,4.35920123710257));
#16787=CARTESIAN_POINT('Ctrl Pts',(-3.63101840830467,2.17455880850134,4.34808744804577));
#16788=CARTESIAN_POINT('Ctrl Pts',(-3.80622350631146,2.30383864322893,4.33697365898897));
#16789=CARTESIAN_POINT('Ctrl Pts',(-3.79264467134891,2.52101708096281,4.32585986993216));
#16790=CARTESIAN_POINT('Ctrl Pts',(-3.60278716655164,2.62766630992157,4.31474608087536));
#16791=CARTESIAN_POINT('Ctrl Pts',(-3.41026840051456,2.5254403942132,4.30363229181855));
#16792=CARTESIAN_POINT('Ctrl Pts',(-3.3979620342723,2.38152235915268,4.29622309911402));
#16793=CARTESIAN_POINT('Ctrl Pts',(-3.42361008748734,2.32286851675082,4.29251850276175));
#16794=CARTESIAN_POINT('Ctrl Pts',(-3.44347998857283,2.53312198033322,5.22244449171475));
#16795=CARTESIAN_POINT('Ctrl Pts',(-3.39921376300775,2.48107535276698,5.21873989536248));
#16796=CARTESIAN_POINT('Ctrl Pts',(-3.36748900863419,2.33020914211697,5.21133070265795));
#16797=CARTESIAN_POINT('Ctrl Pts',(-3.53276736069978,2.16647689674201,5.20021691360114));
#16798=CARTESIAN_POINT('Ctrl Pts',(-3.75962266266454,2.21702523769905,5.18910312454434));
#16799=CARTESIAN_POINT('Ctrl Pts',(-3.84035223774737,2.43479235077285,5.17798933548753));
#16800=CARTESIAN_POINT('Ctrl Pts',(-3.70109553522054,2.62084298334156,5.16687554643073));
#16801=CARTESIAN_POINT('Ctrl Pts',(-3.46929950811782,2.60468896536386,5.15576175737392));
#16802=CARTESIAN_POINT('Ctrl Pts',(-3.35713783891219,2.401213058351,5.14464796831712));
#16803=CARTESIAN_POINT('Ctrl Pts',(-3.46726930372222,2.19661072251331,5.13353417926031));
#16804=CARTESIAN_POINT('Ctrl Pts',(-3.69889135748228,2.17818094124235,5.12242039020352));
#16805=CARTESIAN_POINT('Ctrl Pts',(-3.83999669192638,2.36278064343714,5.1113066011467));
#16806=CARTESIAN_POINT('Ctrl Pts',(-3.76143050146621,2.5814496508346,5.1001928120899));
#16807=CARTESIAN_POINT('Ctrl Pts',(-3.53510505788101,2.63403473315196,5.0890790230331));
#16808=CARTESIAN_POINT('Ctrl Pts',(-3.36817873292179,2.47240567046266,5.07796523397629));
#16809=CARTESIAN_POINT('Ctrl Pts',(-3.41344102170209,2.24450262655374,5.06685144491949));
#16810=CARTESIAN_POINT('Ctrl Pts',(-3.6294628695539,2.15892821683407,5.05573765586269));
#16811=CARTESIAN_POINT('Ctrl Pts',(-3.81851701352091,2.29400948184958,5.04462386680588));
#16812=CARTESIAN_POINT('Ctrl Pts',(-3.80756005948302,2.52610510127557,5.03351007774908));
#16813=CARTESIAN_POINT('Ctrl Pts',(-3.60662102779949,2.64277527582587,5.02239628869227));
#16814=CARTESIAN_POINT('Ctrl Pts',(-3.39962169493761,2.53723049491962,5.01128249963547));
#16815=CARTESIAN_POINT('Ctrl Pts',(-3.3760308968172,2.30607708183528,5.00016871057867));
#16816=CARTESIAN_POINT('Ctrl Pts',(-3.55744155898554,2.16089238284251,4.98905492152186));
#16817=CARTESIAN_POINT('Ctrl Pts',(-3.77780644477848,2.23456559653136,4.97794113246506));
#16818=CARTESIAN_POINT('Ctrl Pts',(-3.83542307524414,2.45966279635197,4.96682734340825));
#16819=CARTESIAN_POINT('Ctrl Pts',(-3.67755429503925,2.63014996180817,4.95571355435145));
#16820=CARTESIAN_POINT('Ctrl Pts',(-3.44869918906956,2.58997825726379,4.94459976529464));
#16821=CARTESIAN_POINT('Ctrl Pts',(-3.35833143120733,2.37591729928569,4.93348597623784));
#16822=CARTESIAN_POINT('Ctrl Pts',(-3.48916565507154,2.18389951041786,4.92237218718103));
#16823=CARTESIAN_POINT('Ctrl Pts',(-3.72144781179447,2.18968095039579,4.91125839812423));
#16824=CARTESIAN_POINT('Ctrl Pts',(-3.84256740907069,2.38796980166419,4.90014460906742));
#16825=CARTESIAN_POINT('Ctrl Pts',(-3.74166230592267,2.59727002989735,4.88903082001062));
#16826=CARTESIAN_POINT('Ctrl Pts',(-3.51109208760397,2.62600676257303,4.87791703095382));
#16827=CARTESIAN_POINT('Ctrl Pts',(-3.36190028978558,2.44787694237367,4.86680324189701));
#16828=CARTESIAN_POINT('Ctrl Pts',(-3.43064385696086,2.2259248138587,4.85568945284022));
#16829=CARTESIAN_POINT('Ctrl Pts',(-3.65440102248913,2.16330567736551,4.8445756637834));
#16830=CARTESIAN_POINT('Ctrl Pts',(-3.82836431518356,2.31733553867597,4.8334618747266));
#16831=CARTESIAN_POINT('Ctrl Pts',(-3.79330316036299,2.54702911891502,4.8223480856698));
#16832=CARTESIAN_POINT('Ctrl Pts',(-3.58130943065524,2.64214527918755,4.81123429661299));
#16833=CARTESIAN_POINT('Ctrl Pts',(-3.38642339103422,2.51562311930547,4.80012050755619));
#16834=CARTESIAN_POINT('Ctrl Pts',(-3.38702644372307,2.28326980706774,4.78900671849939));
#16835=CARTESIAN_POINT('Ctrl Pts',(-3.58256660775658,2.15776096423133,4.77789292944257));
#16836=CARTESIAN_POINT('Ctrl Pts',(-3.79406375341862,2.2539762580115,4.76677914038578));
#16837=CARTESIAN_POINT('Ctrl Pts',(-3.82793214474394,2.48384873885561,4.75566535132897));
#16838=CARTESIAN_POINT('Ctrl Pts',(-3.65317165905879,2.6369735181158,4.74455156227217));
#16839=CARTESIAN_POINT('Ctrl Pts',(-3.42974255082951,2.57319374878213,4.73343777321536));
#16840=CARTESIAN_POINT('Ctrl Pts',(-3.36215201667677,2.35088777703746,4.72232398415856));
#16841=CARTESIAN_POINT('Ctrl Pts',(-3.51226643903938,2.1735347799409,4.71121019510176));
#16842=CARTESIAN_POINT('Ctrl Pts',(-3.74268438471549,2.20346796705471,4.70009640604495));
#16843=CARTESIAN_POINT('Ctrl Pts',(-3.84250169491054,2.41328915274817,4.68898261698815));
#16844=CARTESIAN_POINT('Ctrl Pts',(-3.7203544535977,2.61094662622203,4.67786882793133));
#16845=CARTESIAN_POINT('Ctrl Pts',(-3.48804541599454,2.61552226041731,4.66675503887454));
#16846=CARTESIAN_POINT('Ctrl Pts',(-3.35820967878295,2.42282792546417,4.65564124981773));
#16847=CARTESIAN_POINT('Ctrl Pts',(-3.44968736466998,2.20923893144694,4.64452746076093));
#16848=CARTESIAN_POINT('Ctrl Pts',(-3.67874791033599,2.17025570685489,4.63341367170413));
#16849=CARTESIAN_POINT('Ctrl Pts',(-3.83572960060904,2.34156003925422,4.62229988264732));
#16850=CARTESIAN_POINT('Ctrl Pts',(-3.77694531408991,2.56635513048207,4.61118609359051));
#16851=CARTESIAN_POINT('Ctrl Pts',(-3.55620097488638,2.63888348417682,4.60007230453371));
#16852=CARTESIAN_POINT('Ctrl Pts',(-3.3755463800872,2.4927590756963,4.58895851547691));
#16853=CARTESIAN_POINT('Ctrl Pts',(-3.40033672906513,2.26173123324197,4.5778447264201));
#16854=CARTESIAN_POINT('Ctrl Pts',(-3.60788113427776,2.15726236113484,4.5667309373633));
#16855=CARTESIAN_POINT('Ctrl Pts',(-3.80821184788277,2.27497400259471,4.55561714830649));
#16856=CARTESIAN_POINT('Ctrl Pts',(-3.81796389588787,2.50712335760782,4.54450335924969));
#16857=CARTESIAN_POINT('Ctrl Pts',(-3.62821111800771,2.64122148806661,4.53338957019289));
#16858=CARTESIAN_POINT('Ctrl Pts',(-3.41263638408026,2.55452685581013,4.52227578113608));
#16859=CARTESIAN_POINT('Ctrl Pts',(-3.36855769224962,2.32639203807509,4.51116199207928));
#16860=CARTESIAN_POINT('Ctrl Pts',(-3.536320770243,2.1656314264689,4.50004820302247));
#16861=CARTESIAN_POINT('Ctrl Pts',(-3.76237016779111,2.21939102051171,4.48893441396567));
#16862=CARTESIAN_POINT('Ctrl Pts',(-3.83980031258758,2.43846407699132,4.47782062490887));
#16863=CARTESIAN_POINT('Ctrl Pts',(-3.69773850528383,2.62233049702197,4.46670683585206));
#16864=CARTESIAN_POINT('Ctrl Pts',(-3.46621554861493,2.60269535293104,4.45559304679526));
#16865=CARTESIAN_POINT('Ctrl Pts',(-3.35714699158608,2.39753073103871,4.44447925773845));
#16866=CARTESIAN_POINT('Ctrl Pts',(-3.47036459922058,2.19462650439043,4.43336546868165));
#16867=CARTESIAN_POINT('Ctrl Pts',(-3.70223885539349,2.17970247609322,4.42225167962484));
#16868=CARTESIAN_POINT('Ctrl Pts',(-3.84053293591263,2.36642025342839,4.41113789056805));
#16869=CARTESIAN_POINT('Ctrl Pts',(-3.75866407558161,2.58387198408852,4.40002410151123));
#16870=CARTESIAN_POINT('Ctrl Pts',(-3.53156902199863,2.63302754596983,4.38891031245443));
#16871=CARTESIAN_POINT('Ctrl Pts',(-3.36710794775451,2.46888245639993,4.37779652339763));
#16872=CARTESIAN_POINT('Ctrl Pts',(-3.41581895566904,2.24170428297288,4.36668273434082));
#16873=CARTESIAN_POINT('Ctrl Pts',(-3.63310626324856,2.15938431915927,4.35556894528402));
#16874=CARTESIAN_POINT('Ctrl Pts',(-3.82010444962002,2.29736600407305,4.34445515622722));
#16875=CARTESIAN_POINT('Ctrl Pts',(-3.80561162070166,2.52916276362653,4.33334136717041));
#16876=CARTESIAN_POINT('Ctrl Pts',(-3.60297477126067,2.64299057240655,4.32222757811361));
#16877=CARTESIAN_POINT('Ctrl Pts',(-3.39749753058122,2.53388381093044,4.3111137890568));
#16878=CARTESIAN_POINT('Ctrl Pts',(-3.38436282049399,2.380278625644,4.30370459635227));
#16879=CARTESIAN_POINT('Ctrl Pts',(-3.41173724903364,2.31767678198965,4.3));
#16880=CARTESIAN_POINT('Ctrl Pts',(-3.47309291201476,2.50793586530485,5.2));
#16881=CARTESIAN_POINT('Ctrl Pts',(-3.46488109712516,2.50027511355887,5.2));
#16882=CARTESIAN_POINT('Ctrl Pts',(-3.45756392397337,2.49177395403935,5.2));
#16883=CARTESIAN_POINT('Ctrl Pts',(-3.45114582175476,2.48262659215394,5.2));
#16884=CARTESIAN_POINT('Ctrl Pts',(-3.44637505636198,2.47582708724863,5.2));
#16885=CARTESIAN_POINT('Ctrl Pts',(-3.44210140258396,2.46866923691254,5.2));
#16886=CARTESIAN_POINT('Ctrl Pts',(-3.4383368615674,2.46121837901648,5.2));
#16887=CARTESIAN_POINT('Ctrl Pts',(-3.43611956164057,2.45682985287343,5.2));
#16888=CARTESIAN_POINT('Ctrl Pts',(-3.43407749071882,2.45233446363919,5.2));
#16889=CARTESIAN_POINT('Ctrl Pts',(-3.4322255599542,2.44777399682775,5.2));
#16890=CARTESIAN_POINT('Ctrl Pts',(-3.42766722424942,2.43654888026604,5.2));
#16891=CARTESIAN_POINT('Ctrl Pts',(-3.42424189960471,2.42490562017205,5.2));
#16892=CARTESIAN_POINT('Ctrl Pts',(-3.42197767565222,2.41304271238881,5.2));
#16893=CARTESIAN_POINT('Ctrl Pts',(-3.42053879301361,2.40550400048974,5.2));
#16894=CARTESIAN_POINT('Ctrl Pts',(-3.41956954249672,2.39787570455109,5.2));
#16895=CARTESIAN_POINT('Ctrl Pts',(-3.41908669765048,2.39020364672881,5.2));
#16896=CARTESIAN_POINT('Ctrl Pts',(-3.4188613702662,2.3866233564252,5.2));
#16897=CARTESIAN_POINT('Ctrl Pts',(-3.4187425132976,2.38303698501937,5.2));
#16898=CARTESIAN_POINT('Ctrl Pts',(-3.4187312729093,2.37945933257344,5.2));
#16899=CARTESIAN_POINT('Ctrl Pts',(-3.41869622423253,2.36830384747272,5.2));
#16900=CARTESIAN_POINT('Ctrl Pts',(-3.4197031160267,2.35720597826242,5.2));
#16901=CARTESIAN_POINT('Ctrl Pts',(-3.42178566785009,2.34630687436894,5.2));
#16902=CARTESIAN_POINT('Ctrl Pts',(-3.42294604955552,2.3402339783087,5.2));
#16903=CARTESIAN_POINT('Ctrl Pts',(-3.42444092603953,2.33422255306027,5.2));
#16904=CARTESIAN_POINT('Ctrl Pts',(-3.42625156753842,2.32828873958556,5.2));
#16905=CARTESIAN_POINT('Ctrl Pts',(-3.42738421175614,2.32457685099508,5.2));
#16906=CARTESIAN_POINT('Ctrl Pts',(-3.42864107094821,2.32089381471682,5.2));
#16907=CARTESIAN_POINT('Ctrl Pts',(-3.4300164442918,2.31724844575858,5.2));
#16908=CARTESIAN_POINT('Ctrl Pts',(-3.43439823178552,2.30563470307137,5.2));
#16909=CARTESIAN_POINT('Ctrl Pts',(-3.43994733372525,2.29448387749046,5.2));
#16910=CARTESIAN_POINT('Ctrl Pts',(-3.44649833143843,2.28391851131164,5.2));
#16911=CARTESIAN_POINT('Ctrl Pts',(-3.45083930540137,2.27691744345919,5.2));
#16912=CARTESIAN_POINT('Ctrl Pts',(-3.45562139981211,2.27017330264703,5.2));
#16913=CARTESIAN_POINT('Ctrl Pts',(-3.46080803162185,2.26372396193311,5.2));
#16914=CARTESIAN_POINT('Ctrl Pts',(-3.46351816065219,2.2603540397685,5.2));
#16915=CARTESIAN_POINT('Ctrl Pts',(-3.46634013864158,2.25706328802701,5.2));
#16916=CARTESIAN_POINT('Ctrl Pts',(-3.46926558695491,2.25386191331523,5.2));
#16917=CARTESIAN_POINT('Ctrl Pts',(-3.47553201369268,2.24700444124844,5.2));
#16918=CARTESIAN_POINT('Ctrl Pts',(-3.48224798017073,2.24058272300471,5.2));
#16919=CARTESIAN_POINT('Ctrl Pts',(-3.48935940275436,2.23464751188384,5.2));
#16920=CARTESIAN_POINT('Ctrl Pts',(-3.49388585721574,2.23086972163985,5.2));
#16921=CARTESIAN_POINT('Ctrl Pts',(-3.49857277644925,2.2272891074735,5.2));
#16922=CARTESIAN_POINT('Ctrl Pts',(-3.50340840926684,2.2239201748241,5.2));
#16923=CARTESIAN_POINT('Ctrl Pts',(-3.50748096973522,2.22108286635877,5.2));
#16924=CARTESIAN_POINT('Ctrl Pts',(-3.51165201299164,2.21840074277452,5.2));
#16925=CARTESIAN_POINT('Ctrl Pts',(-3.51591072169151,2.21588342574414,5.2));
#16926=CARTESIAN_POINT('Ctrl Pts',(-3.52463381704441,2.21072721571968,5.2));
#16927=CARTESIAN_POINT('Ctrl Pts',(-3.53372795060187,2.20625881994954,5.2));
#16928=CARTESIAN_POINT('Ctrl Pts',(-3.54313435341931,2.20255201733462,5.2));
#16929=CARTESIAN_POINT('Ctrl Pts',(-3.5443736619696,2.20206364018726,5.2));
#16930=CARTESIAN_POINT('Ctrl Pts',(-3.54561840623672,2.20158850319392,5.2));
#16931=CARTESIAN_POINT('Ctrl Pts',(-3.54686839490754,2.2011265482535,5.2));
#16932=CARTESIAN_POINT('Ctrl Pts',(-3.76673280722786,2.39986996770474,5.08714803633902));
#16933=CARTESIAN_POINT('Ctrl Pts',(-3.76680595967625,2.39134538779314,5.08771939403666));
#16934=CARTESIAN_POINT('Ctrl Pts',(-3.76620865205667,2.38283109327188,5.08829075173431));
#16935=CARTESIAN_POINT('Ctrl Pts',(-3.76490523356496,2.37442631092714,5.08886210943196));
#16936=CARTESIAN_POINT('Ctrl Pts',(-3.75645406644185,2.31993098139145,5.09256670578422));
#16937=CARTESIAN_POINT('Ctrl Pts',(-3.71831779890178,2.27003957467425,5.0962713021365));
#16938=CARTESIAN_POINT('Ctrl Pts',(-3.66794964148213,2.24758436209697,5.09997589848877));
#16939=CARTESIAN_POINT('Ctrl Pts',(-3.61758148406248,2.22512914951968,5.10368049484103));
#16940=CARTESIAN_POINT('Ctrl Pts',(-3.55498143676326,2.2301101310823,5.1073850911933));
#16941=CARTESIAN_POINT('Ctrl Pts',(-3.50879890345119,2.26024936189732,5.11108968754557));
#16942=CARTESIAN_POINT('Ctrl Pts',(-3.46261637013913,2.29038859271235,5.11479428389783));
#16943=CARTESIAN_POINT('Ctrl Pts',(-3.43285135081423,2.34568607277977,5.1184988802501));
#16944=CARTESIAN_POINT('Ctrl Pts',(-3.43312570053424,2.40083133397043,5.12220347660237));
#16945=CARTESIAN_POINT('Ctrl Pts',(-3.43340005025424,2.45597659516109,5.12590807295464));
#16946=CARTESIAN_POINT('Ctrl Pts',(-3.46371376901915,2.51096963747498,5.12961266930691));
#16947=CARTESIAN_POINT('Ctrl Pts',(-3.51019416177169,2.54064911632758,5.13331726565918));
#16948=CARTESIAN_POINT('Ctrl Pts',(-3.55667455452423,2.57032859518018,5.13702186201145));
#16949=CARTESIAN_POINT('Ctrl Pts',(-3.61932162126441,2.57469451057149,5.14072645836371));
#16950=CARTESIAN_POINT('Ctrl Pts',(-3.6694634753069,2.55173569482678,5.14443105471598));
#16951=CARTESIAN_POINT('Ctrl Pts',(-3.71960532934939,2.52877687908207,5.14813565106825));
#16952=CARTESIAN_POINT('Ctrl Pts',(-3.75724197069419,2.47849333220135,5.15184024742052));
#16953=CARTESIAN_POINT('Ctrl Pts',(-3.76515097781766,2.42392380920663,5.15554484377278));
#16954=CARTESIAN_POINT('Ctrl Pts',(-3.76629187237323,2.41605201560311,5.15607924129486));
#16955=CARTESIAN_POINT('Ctrl Pts',(-3.76681417046854,2.40809103597041,5.15661363881694));
#16956=CARTESIAN_POINT('Ctrl Pts',(-3.76674783252531,2.40012156540224,5.15714803633902));
#16957=CARTESIAN_POINT('Ctrl Pts',(-3.65301702171886,2.20148256743283,5.2));
#16958=CARTESIAN_POINT('Ctrl Pts',(-3.71902879097456,2.21911198848201,5.19629540364773));
#16959=CARTESIAN_POINT('Ctrl Pts',(-3.83093279751213,2.32515241961692,5.1888862109432));
#16960=CARTESIAN_POINT('Ctrl Pts',(-3.78812294461068,2.55382789975093,5.17777242188639));
#16961=CARTESIAN_POINT('Ctrl Pts',(-3.57278676575927,2.64128531597693,5.16665863282959));
#16962=CARTESIAN_POINT('Ctrl Pts',(-3.38252462806861,2.5080933346037,5.15554484377278));
#16963=CARTESIAN_POINT('Ctrl Pts',(-3.39123766596766,2.27586209704876,5.14443105471597));
#16964=CARTESIAN_POINT('Ctrl Pts',(-3.59107442724388,2.15730569128375,5.13331726565918));
#16965=CARTESIAN_POINT('Ctrl Pts',(-3.79906029518588,2.2608651698129,5.12220347660237));
#16966=CARTESIAN_POINT('Ctrl Pts',(-3.82485429121136,2.49178880612566,5.11108968754556));
#16967=CARTESIAN_POINT('Ctrl Pts',(-3.64483147349944,2.63869087951471,5.09997589848877));
#16968=CARTESIAN_POINT('Ctrl Pts',(-3.42377646220466,2.56711959422357,5.08886210943196));
#16969=CARTESIAN_POINT('Ctrl Pts',(-3.36401957377094,2.34258029572384,5.07774832037515));
#16970=CARTESIAN_POINT('Ctrl Pts',(-3.52025888482579,2.17059867951396,5.06663453131835));
#16971=CARTESIAN_POINT('Ctrl Pts',(-3.74948582371233,2.20859030608788,5.05552074226155));
#16972=CARTESIAN_POINT('Ctrl Pts',(-3.8418868522934,2.42178158973285,5.04440695320474));
#16973=CARTESIAN_POINT('Ctrl Pts',(-3.71288602216703,2.61503584063672,5.03329316414794));
#16974=CARTESIAN_POINT('Ctrl Pts',(-3.48055937550073,2.61146539619723,5.02217937509113));
#16975=CARTESIAN_POINT('Ctrl Pts',(-3.35755806712823,2.4143382523336,5.01106558603433));
#16976=CARTESIAN_POINT('Ctrl Pts',(-3.45646661930996,2.20408715554039,4.99995179697752));
#16977=CARTESIAN_POINT('Ctrl Pts',(-3.68675289766315,2.17315730107164,4.98883800792072));
#16978=CARTESIAN_POINT('Ctrl Pts',(-3.83763326741432,2.34985914450584,4.97772421886391));
#16979=CARTESIAN_POINT('Ctrl Pts',(-3.77100521132112,2.57245548011022,4.96661042980712));
#16980=CARTESIAN_POINT('Ctrl Pts',(-3.54785414659174,2.63720135974049,4.9554966407503));
#16981=CARTESIAN_POINT('Ctrl Pts',(-3.37243277255298,2.48483414437987,4.94438285169351));
#16982=CARTESIAN_POINT('Ctrl Pts',(-3.40530626273826,2.25481727477052,4.9332690626367));
#16983=CARTESIAN_POINT('Ctrl Pts',(-3.61638513853951,2.15768779995451,4.9221552735799));
#16984=CARTESIAN_POINT('Ctrl Pts',(-3.81246651125382,2.28234942989398,4.91104148452309));
#16985=CARTESIAN_POINT('Ctrl Pts',(-3.81407487666422,2.51469796087643,4.89992769546629));
#16986=CARTESIAN_POINT('Ctrl Pts',(-3.6197380796992,2.64206214751696,4.88881390640948));
#16987=CARTESIAN_POINT('Ctrl Pts',(-3.40733479453568,2.54786410535795,4.87770011735268));
#16988=CARTESIAN_POINT('Ctrl Pts',(-3.37128015690807,2.3183243706747,4.86658632829587));
#16989=CARTESIAN_POINT('Ctrl Pts',(-3.54457538552076,2.16354326577609,4.85547253923908));
#16990=CARTESIAN_POINT('Ctrl Pts',(-3.76860139232476,2.2251936913151,4.84435875018226));
#16991=CARTESIAN_POINT('Ctrl Pts',(-3.83830463266378,2.44684631363142,4.83324496112547));
#16992=CARTESIAN_POINT('Ctrl Pts',(-3.68988494016744,2.62561997380774,4.82213117206865));
#16993=CARTESIAN_POINT('Ctrl Pts',(-3.45919254257122,2.59788111325323,4.81101738301186));
#16994=CARTESIAN_POINT('Ctrl Pts',(-3.35738280762477,2.38901942561361,4.79990359395505));
#16995=CARTESIAN_POINT('Ctrl Pts',(-3.47764334032546,2.19020838223802,4.78878980489825));
#16996=CARTESIAN_POINT('Ctrl Pts',(-3.70989831124516,2.18342198579874,4.77767601584144));
#16997=CARTESIAN_POINT('Ctrl Pts',(-3.84156211155055,2.3748719019196,4.76656222678464));
#16998=CARTESIAN_POINT('Ctrl Pts',(-3.75212137165305,2.58932185118547,4.75544843772783));
#16999=CARTESIAN_POINT('Ctrl Pts',(-3.52344221510783,2.63048336300545,4.74433464867103));
#17000=CARTESIAN_POINT('Ctrl Pts',(-3.36483726729874,2.46068083880743,4.73322085961422));
#17001=CARTESIAN_POINT('Ctrl Pts',(-3.42147943565789,2.23533645468145,4.72210707055742));
#17002=CARTESIAN_POINT('Ctrl Pts',(-3.64152350112028,2.16071048099716,4.71099328150062));
#17003=CARTESIAN_POINT('Ctrl Pts',(-3.82356063509873,2.30510891778388,4.69987949244381));
#17004=CARTESIAN_POINT('Ctrl Pts',(-3.80097018442129,2.53636223826109,4.68876570338701));
#17005=CARTESIAN_POINT('Ctrl Pts',(-3.59442944478611,2.64280165560495,4.6776519143302));
#17006=CARTESIAN_POINT('Ctrl Pts',(-3.39298749751263,2.52700196401557,4.6665381252734));
#17007=CARTESIAN_POINT('Ctrl Pts',(-3.38102644144724,2.29495593446246,4.65542433621659));
#17008=CARTESIAN_POINT('Ctrl Pts',(-3.56949436685434,2.15905792937668,4.64431054715979));
#17009=CARTESIAN_POINT('Ctrl Pts',(-3.7858844442369,2.24369693400118,4.63319675810299));
#17010=CARTESIAN_POINT('Ctrl Pts',(-3.83213238173679,2.47140190753206,4.62208296904618));
#17011=CARTESIAN_POINT('Ctrl Pts',(-3.66590691767206,2.63375190534549,4.61096917998937));
#17012=CARTESIAN_POINT('Ctrl Pts',(-3.43935610442817,2.58214613327058,4.59985539093257));
#17013=CARTESIAN_POINT('Ctrl Pts',(-3.35984447062414,2.36381993973287,4.58874160187577));
#17014=CARTESIAN_POINT('Ctrl Pts',(-3.50014991641224,2.17860976567263,4.57762781281897));
#17015=CARTESIAN_POINT('Ctrl Pts',(-3.73184927607424,2.1960405838179,4.56651402376216));
#17016=CARTESIAN_POINT('Ctrl Pts',(-3.84286549809491,2.40015776867247,4.55540023470536));
#17017=CARTESIAN_POINT('Ctrl Pts',(-3.73158417538336,2.60413054603043,4.54428644564855));
#17018=CARTESIAN_POINT('Ctrl Pts',(-3.49986236476522,2.62126031969194,4.53317265659175));
#17019=CARTESIAN_POINT('Ctrl Pts',(-3.35979766713961,2.43586801331045,4.52205886753494));
#17020=CARTESIAN_POINT('Ctrl Pts',(-3.43959288921302,2.2176453079079,4.51094507847814));
#17021=CARTESIAN_POINT('Ctrl Pts',(-3.66621055822496,2.16633391955349,4.49983128942134));
#17022=CARTESIAN_POINT('Ctrl Pts',(-3.83222495382674,2.32889974592014,4.48871750036453));
#17023=CARTESIAN_POINT('Ctrl Pts',(-3.78568121275365,2.55654443850517,4.47760371130773));
#17024=CARTESIAN_POINT('Ctrl Pts',(-3.56918135753979,2.64090223654315,4.46648992225092));
#17025=CARTESIAN_POINT('Ctrl Pts',(-3.38089014394226,2.50475947474088,4.45537613319412));
#17026=CARTESIAN_POINT('Ctrl Pts',(-3.3931526891646,2.27272919910994,4.44426234413731));
#17027=CARTESIAN_POINT('Ctrl Pts',(-3.59474487835949,2.15719128792351,4.43314855508051));
#17028=CARTESIAN_POINT('Ctrl Pts',(-3.80114723098,2.26389903055612,4.4220347660237));
#17029=CARTESIAN_POINT('Ctrl Pts',(-3.82343705972838,2.49518136177793,4.4109209769669));
#17030=CARTESIAN_POINT('Ctrl Pts',(-3.64121277856108,2.63934345799643,4.3998071879101));
#17031=CARTESIAN_POINT('Ctrl Pts',(-3.4212652433475,2.56443108225311,4.38869339885329));
#17032=CARTESIAN_POINT('Ctrl Pts',(-3.36491712045917,2.33901445477475,4.3775796097965));
#17033=CARTESIAN_POINT('Ctrl Pts',(-3.52374009472539,2.16941582002738,4.36646582073968));
#17034=CARTESIAN_POINT('Ctrl Pts',(-3.75237048890211,2.21087904346051,4.35535203168288));
#17035=CARTESIAN_POINT('Ctrl Pts',(-3.84152270551859,2.42543572391857,4.34423824262608));
#17036=CARTESIAN_POINT('Ctrl Pts',(-3.70962996035205,2.61673302206395,4.33312445356927));
#17037=CARTESIAN_POINT('Ctrl Pts',(-3.47734458963256,2.60960762555316,4.32201066451247));
#17038=CARTESIAN_POINT('Ctrl Pts',(-3.35742145615876,2.41071512444121,4.31089687545567));
#17039=CARTESIAN_POINT('Ctrl Pts',(-3.45934316515028,2.20183612882053,4.29978308639885));
#17040=CARTESIAN_POINT('Ctrl Pts',(-3.69040350703126,2.17470170179864,4.28866929734206));
#17041=CARTESIAN_POINT('Ctrl Pts',(-3.7885754343637,2.29356865430552,4.28126010463752));
#17042=CARTESIAN_POINT('Ctrl Pts',(-3.80166758614466,2.36062792457102,4.27755550828525));
#17043=CARTESIAN_POINT('Ctrl Pts',(-3.64967348970877,2.21400211999972,5.20748149723825));
#17044=CARTESIAN_POINT('Ctrl Pts',(-3.71152220988337,2.2305197371096,5.20377690088598));
#17045=CARTESIAN_POINT('Ctrl Pts',(-3.81636896167925,2.32987270138258,5.19636770818145));
#17046=CARTESIAN_POINT('Ctrl Pts',(-3.7762589230805,2.54412670398045,5.18525391912464));
#17047=CARTESIAN_POINT('Ctrl Pts',(-3.57450297532427,2.62606859592404,5.17414013006784));
#17048=CARTESIAN_POINT('Ctrl Pts',(-3.39623976792153,2.50127640086039,5.16302634101103));
#17049=CARTESIAN_POINT('Ctrl Pts',(-3.404403315861,2.28369088559113,5.15191255195423));
#17050=CARTESIAN_POINT('Ctrl Pts',(-3.59163732076848,2.17261126982347,5.14079876289742));
#17051=CARTESIAN_POINT('Ctrl Pts',(-3.78650650684933,2.26963974340016,5.12968497384063));
#17052=CARTESIAN_POINT('Ctrl Pts',(-3.8106737979302,2.48600012163341,5.11857118478381));
#17053=CARTESIAN_POINT('Ctrl Pts',(-3.64200416517759,2.62363777825967,5.10745739572702));
#17054=CARTESIAN_POINT('Ctrl Pts',(-3.43489004460608,2.55658015434777,5.0963436066702));
#17055=CARTESIAN_POINT('Ctrl Pts',(-3.37890173959752,2.34620148403342,5.0852298176134));
#17056=CARTESIAN_POINT('Ctrl Pts',(-3.52528777861237,2.18506593235721,5.0741160285566));
#17057=CARTESIAN_POINT('Ctrl Pts',(-3.74005846207577,2.22066160730187,5.06300223949979));
#17058=CARTESIAN_POINT('Ctrl Pts',(-3.82663219619914,2.42040792821545,5.05188845044299));
#17059=CARTESIAN_POINT('Ctrl Pts',(-3.70576683635895,2.60147455044772,5.04077466138619));
#17060=CARTESIAN_POINT('Ctrl Pts',(-3.4880919289783,2.59812927699836,5.02966087232938));
#17061=CARTESIAN_POINT('Ctrl Pts',(-3.37284772952088,2.41343400678959,5.01854708327258));
#17062=CARTESIAN_POINT('Ctrl Pts',(-3.46551858860765,2.21644244909332,5.00743329421577));
#17063=CARTESIAN_POINT('Ctrl Pts',(-3.68128180402377,2.18746319379313,4.99631950515897));
#17064=CARTESIAN_POINT('Ctrl Pts',(-3.82264686473641,2.35302129035867,4.98520571610216));
#17065=CARTESIAN_POINT('Ctrl Pts',(-3.76022072401106,2.56157953122871,4.97409192704537));
#17066=CARTESIAN_POINT('Ctrl Pts',(-3.55114273814991,2.6222421954303,4.96297813798855));
#17067=CARTESIAN_POINT('Ctrl Pts',(-3.38678435785046,2.47948405740616,4.95186434893176));
#17068=CARTESIAN_POINT('Ctrl Pts',(-3.41758467298453,2.26397326040267,4.94075055987495));
#17069=CARTESIAN_POINT('Ctrl Pts',(-3.61535180559434,2.17296928071335,4.92963677081814));
#17070=CARTESIAN_POINT('Ctrl Pts',(-3.79906725647832,2.28976909313423,4.91852298176134));
#17071=CARTESIAN_POINT('Ctrl Pts',(-3.80057418991348,2.50746450469106,4.90740919270453));
#17072=CARTESIAN_POINT('Ctrl Pts',(-3.61849329266379,2.62679643638467,4.89629540364773));
#17073=CARTESIAN_POINT('Ctrl Pts',(-3.41948527490624,2.53853901780343,4.88518161459093));
#17074=CARTESIAN_POINT('Ctrl Pts',(-3.38570443220547,2.32347526509011,4.87406782553412));
#17075=CARTESIAN_POINT('Ctrl Pts',(-3.54807075298295,2.17845547008797,4.86295403647732));
#17076=CARTESIAN_POINT('Ctrl Pts',(-3.7579685024734,2.23621789580084,4.85184024742051));
#17077=CARTESIAN_POINT('Ctrl Pts',(-3.82327589016501,2.44389193890226,4.84072645836371));
#17078=CARTESIAN_POINT('Ctrl Pts',(-3.6842163234679,2.61139119255816,4.8296126693069));
#17079=CARTESIAN_POINT('Ctrl Pts',(-3.4680726008225,2.58540169032632,4.8184988802501));
#17080=CARTESIAN_POINT('Ctrl Pts',(-3.37268352280275,2.38971191834066,4.8073850911933));
#17081=CARTESIAN_POINT('Ctrl Pts',(-3.48535979430583,2.20343894417256,4.79627130213649));
#17082=CARTESIAN_POINT('Ctrl Pts',(-3.70296754618914,2.19708053355731,4.78515751307969));
#17083=CARTESIAN_POINT('Ctrl Pts',(-3.82632793531414,2.37645661184032,4.77404372402288));
#17084=CARTESIAN_POINT('Ctrl Pts',(-3.74252779851275,2.57738222030606,4.76292993496608));
#17085=CARTESIAN_POINT('Ctrl Pts',(-3.52827035135747,2.61594787087447,4.75181614590928));
#17086=CARTESIAN_POINT('Ctrl Pts',(-3.37966786507423,2.45685398621605,4.74070235685247));
#17087=CARTESIAN_POINT('Ctrl Pts',(-3.43273788062492,2.24572100320602,4.72958856779567));
#17088=CARTESIAN_POINT('Ctrl Pts',(-3.63890481092106,2.17580133560435,4.71847477873887));
#17089=CARTESIAN_POINT('Ctrl Pts',(-3.80946172657059,2.31109324810979,4.70736098968206));
#17090=CARTESIAN_POINT('Ctrl Pts',(-3.78829594843252,2.5277625188915,4.69624720062526));
#17091=CARTESIAN_POINT('Ctrl Pts',(-3.59478075327286,2.62748930720629,4.68513341156845));
#17092=CARTESIAN_POINT('Ctrl Pts',(-3.40604279383286,2.51899255273097,4.67401962251165));
#17093=CARTESIAN_POINT('Ctrl Pts',(-3.39483606482192,2.30158056527362,4.66290583345485));
#17094=CARTESIAN_POINT('Ctrl Pts',(-3.57141821239684,2.17425300257371,4.65179204439804));
#17095=CARTESIAN_POINT('Ctrl Pts',(-3.77416159430429,2.253554226763,4.64067825534124));
#17096=CARTESIAN_POINT('Ctrl Pts',(-3.81749289381852,2.46689892800445,4.62956446628442));
#17097=CARTESIAN_POINT('Ctrl Pts',(-3.66175048108285,2.61901028175737,4.61845067722763));
#17098=CARTESIAN_POINT('Ctrl Pts',(-3.44948715271524,2.57065904087346,4.60733688817082));
#17099=CARTESIAN_POINT('Ctrl Pts',(-3.37498994039659,2.36610164447049,4.59622309911403));
#17100=CARTESIAN_POINT('Ctrl Pts',(-3.50644698742571,2.19257179732202,4.58510931005721));
#17101=CARTESIAN_POINT('Ctrl Pts',(-3.72353416781713,2.20890333647083,4.57399552100042));
#17102=CARTESIAN_POINT('Ctrl Pts',(-3.82754912345333,2.40014781895086,4.5628817319436));
#17103=CARTESIAN_POINT('Ctrl Pts',(-3.723285785769,2.59125700102993,4.55176794288681));
#17104=CARTESIAN_POINT('Ctrl Pts',(-3.50617757029671,2.60730648114219,4.54065415382999));
#17105=CARTESIAN_POINT('Ctrl Pts',(-3.37494608858577,2.43360598789383,4.52954036477319));
#17106=CARTESIAN_POINT('Ctrl Pts',(-3.44970900460718,2.22914555312034,4.51842657571639));
#17107=CARTESIAN_POINT('Ctrl Pts',(-3.66203497246676,2.18107013057245,4.50731278665959));
#17108=CARTESIAN_POINT('Ctrl Pts',(-3.81757962782599,2.33338370159577,4.49619899760278));
#17109=CARTESIAN_POINT('Ctrl Pts',(-3.77397117966642,2.54667192352462,4.48508520854598));
#17110=CARTESIAN_POINT('Ctrl Pts',(-3.57112494309463,2.62570967549255,4.47397141948917));
#17111=CARTESIAN_POINT('Ctrl Pts',(-3.3947083629539,2.49815279172096,4.46285763043237));
#17112=CARTESIAN_POINT('Ctrl Pts',(-3.40619756763113,2.28075556466066,4.45174384137556));
#17113=CARTESIAN_POINT('Ctrl Pts',(-3.59507629394739,2.17250408134035,4.44063005231876));
#17114=CARTESIAN_POINT('Ctrl Pts',(-3.78846182950481,2.27248227294105,4.42951626326195));
#17115=CARTESIAN_POINT('Ctrl Pts',(-3.80934594451251,2.48917872489734,4.41840247420516));
#17116=CARTESIAN_POINT('Ctrl Pts',(-3.63861368415939,2.62424920171285,4.40728868514834));
#17117=CARTESIAN_POINT('Ctrl Pts',(-3.43253719640727,2.55406119407111,4.39617489609155));
#17118=CARTESIAN_POINT('Ctrl Pts',(-3.37974268227471,2.34286052375416,4.38506110703474));
#17119=CARTESIAN_POINT('Ctrl Pts',(-3.5285494451209,2.18395767020613,4.37394731797793));
#17120=CARTESIAN_POINT('Ctrl Pts',(-3.74276120511889,2.22280600486777,4.36283352892113));
#17121=CARTESIAN_POINT('Ctrl Pts',(-3.82629101443365,2.42383161349583,4.35171973986432));
#17122=CARTESIAN_POINT('Ctrl Pts',(-3.70271611891361,2.60306469869495,4.34060595080752));
#17123=CARTESIAN_POINT('Ctrl Pts',(-3.48507988440164,2.59638866713425,4.32949216175072));
#17124=CARTESIAN_POINT('Ctrl Pts',(-3.37271973395708,2.41003937238272,4.31837837269391));
#17125=CARTESIAN_POINT('Ctrl Pts',(-3.46821372435015,2.21433338394825,4.30726458363711));
#17126=CARTESIAN_POINT('Ctrl Pts',(-3.68470218678007,2.18891019649399,4.2961507945803));
#17127=CARTESIAN_POINT('Ctrl Pts',(-3.77668287645173,2.30028077429396,4.28874160187577));
#17128=CARTESIAN_POINT('Ctrl Pts',(-3.78894936833816,2.36311093455975,4.2850370055235));
#17129=CARTESIAN_POINT('Ctrl Pts',(-3.64632995769868,2.22652167256662,5.2149629944765));
#17130=CARTESIAN_POINT('Ctrl Pts',(-3.70401562879218,2.24192748573719,5.21125839812423));
#17131=CARTESIAN_POINT('Ctrl Pts',(-3.80180512584637,2.33459298314823,5.2038492054197));
#17132=CARTESIAN_POINT('Ctrl Pts',(-3.76439490155032,2.53442550820997,5.19273541636289));
#17133=CARTESIAN_POINT('Ctrl Pts',(-3.57621918488928,2.61085187587115,5.18162162730609));
#17134=CARTESIAN_POINT('Ctrl Pts',(-3.40995490777444,2.49445946711708,5.17050783824928));
#17135=CARTESIAN_POINT('Ctrl Pts',(-3.41756896575436,2.2915196741335,5.15939404919248));
#17136=CARTESIAN_POINT('Ctrl Pts',(-3.59220021429306,2.18791684836318,5.14828026013568));
#17137=CARTESIAN_POINT('Ctrl Pts',(-3.7739527185128,2.27841431698741,5.13716647107887));
#17138=CARTESIAN_POINT('Ctrl Pts',(-3.79649330464903,2.48021143714115,5.12605268202206));
#17139=CARTESIAN_POINT('Ctrl Pts',(-3.63917685685576,2.60858467700464,5.11493889296527));
#17140=CARTESIAN_POINT('Ctrl Pts',(-3.44600362700749,2.54604071447196,5.10382510390845));
#17141=CARTESIAN_POINT('Ctrl Pts',(-3.39378390542411,2.349822672343,5.09271131485166));
#17142=CARTESIAN_POINT('Ctrl Pts',(-3.53031667239896,2.19953318520045,5.08159752579485));
#17143=CARTESIAN_POINT('Ctrl Pts',(-3.73063110043921,2.23273290851586,5.07048373673805));
#17144=CARTESIAN_POINT('Ctrl Pts',(-3.81137754010487,2.41903426669804,5.05936994768123));
#17145=CARTESIAN_POINT('Ctrl Pts',(-3.69864765055087,2.58791326025872,5.04825615862444));
#17146=CARTESIAN_POINT('Ctrl Pts',(-3.49562448245587,2.58479315779948,5.03714236956762));
#17147=CARTESIAN_POINT('Ctrl Pts',(-3.38813739191354,2.41252976124558,5.02602858051083));
#17148=CARTESIAN_POINT('Ctrl Pts',(-3.47457055790533,2.22879774264625,5.01491479145402));
#17149=CARTESIAN_POINT('Ctrl Pts',(-3.67581071038439,2.20176908651461,5.00380100239723));
#17150=CARTESIAN_POINT('Ctrl Pts',(-3.8076604620585,2.35618343621151,4.99268721334041));
#17151=CARTESIAN_POINT('Ctrl Pts',(-3.74943623670099,2.5507035823472,4.98157342428361));
#17152=CARTESIAN_POINT('Ctrl Pts',(-3.55443132970808,2.6072830311201,4.97045963522681));
#17153=CARTESIAN_POINT('Ctrl Pts',(-3.40113594314794,2.47413397043246,4.95934584617));
#17154=CARTESIAN_POINT('Ctrl Pts',(-3.42986308323079,2.27312924603482,4.9482320571132));
#17155=CARTESIAN_POINT('Ctrl Pts',(-3.61431847264918,2.18825076147219,4.93711826805639));
#17156=CARTESIAN_POINT('Ctrl Pts',(-3.78566800170281,2.29718875637448,4.92600447899959));
#17157=CARTESIAN_POINT('Ctrl Pts',(-3.78707350316275,2.50023104850568,4.91489068994278));
#17158=CARTESIAN_POINT('Ctrl Pts',(-3.61724850562837,2.61153072525238,4.90377690088598));
#17159=CARTESIAN_POINT('Ctrl Pts',(-3.43163575527681,2.52921393024892,4.89266311182917));
#17160=CARTESIAN_POINT('Ctrl Pts',(-3.40012870750287,2.32862615950552,4.88154932277238));
#17161=CARTESIAN_POINT('Ctrl Pts',(-3.55156612044514,2.19336767439986,4.87043553371556));
#17162=CARTESIAN_POINT('Ctrl Pts',(-3.74733561262204,2.24724210028659,4.85932174465877));
#17163=CARTESIAN_POINT('Ctrl Pts',(-3.80824714766624,2.4409375641731,4.84820795560196));
#17164=CARTESIAN_POINT('Ctrl Pts',(-3.67854770676838,2.59716241130857,4.83709416654516));
#17165=CARTESIAN_POINT('Ctrl Pts',(-3.47695265907377,2.57292226739941,4.82598037748835));
#17166=CARTESIAN_POINT('Ctrl Pts',(-3.38798423798073,2.39040441106771,4.81486658843155));
#17167=CARTESIAN_POINT('Ctrl Pts',(-3.49307624828619,2.2166695061071,4.80375279937474));
#17168=CARTESIAN_POINT('Ctrl Pts',(-3.69603678113312,2.21073908131588,4.79263901031794));
#17169=CARTESIAN_POINT('Ctrl Pts',(-3.81109375907773,2.37804132176103,4.78152522126113));
#17170=CARTESIAN_POINT('Ctrl Pts',(-3.73293422537244,2.56544258942666,4.77041143220433));
#17171=CARTESIAN_POINT('Ctrl Pts',(-3.5330984876071,2.6014123787435,4.75929764314753));
#17172=CARTESIAN_POINT('Ctrl Pts',(-3.39449846284973,2.45302713362467,4.74818385409072));
#17173=CARTESIAN_POINT('Ctrl Pts',(-3.44399632559195,2.2561055517306,4.73707006503392));
#17174=CARTESIAN_POINT('Ctrl Pts',(-3.63628612072185,2.19089219021153,4.72595627597712));
#17175=CARTESIAN_POINT('Ctrl Pts',(-3.79536281804244,2.31707757843571,4.7148424869203));
#17176=CARTESIAN_POINT('Ctrl Pts',(-3.77562171244375,2.5191627995219,4.70372869786351));
#17177=CARTESIAN_POINT('Ctrl Pts',(-3.5951320617596,2.61217695880763,4.6926149088067));
#17178=CARTESIAN_POINT('Ctrl Pts',(-3.41909809015308,2.51098314144638,4.6815011197499));
#17179=CARTESIAN_POINT('Ctrl Pts',(-3.40864568819661,2.30820519608479,4.67038733069309));
#17180=CARTESIAN_POINT('Ctrl Pts',(-3.57334205793934,2.18944807577074,4.65927354163629));
#17181=CARTESIAN_POINT('Ctrl Pts',(-3.76243874437168,2.26341151952482,4.64815975257949));
#17182=CARTESIAN_POINT('Ctrl Pts',(-3.80285340590026,2.46239594847684,4.63704596352267));
#17183=CARTESIAN_POINT('Ctrl Pts',(-3.65759404449364,2.60426865816925,4.62593217446588));
#17184=CARTESIAN_POINT('Ctrl Pts',(-3.45961820100231,2.55917194847634,4.61481838540907));
#17185=CARTESIAN_POINT('Ctrl Pts',(-3.39013541016905,2.3683833492081,4.60370459635227));
#17186=CARTESIAN_POINT('Ctrl Pts',(-3.51274405843916,2.20653382897141,4.59259080729546));
#17187=CARTESIAN_POINT('Ctrl Pts',(-3.71521905956003,2.22176608912375,4.58147701823867));
#17188=CARTESIAN_POINT('Ctrl Pts',(-3.81223274881174,2.40013786922925,4.57036322918185));
#17189=CARTESIAN_POINT('Ctrl Pts',(-3.71498739615465,2.57838345602943,4.55924944012506));
#17190=CARTESIAN_POINT('Ctrl Pts',(-3.51249277582821,2.59335264259245,4.54813565106824));
#17191=CARTESIAN_POINT('Ctrl Pts',(-3.39009451003192,2.4313439624772,4.53702186201144));
#17192=CARTESIAN_POINT('Ctrl Pts',(-3.45982512000134,2.24064579833279,4.52590807295464));
#17193=CARTESIAN_POINT('Ctrl Pts',(-3.65785938670857,2.1958063415914,4.51479428389783));
#17194=CARTESIAN_POINT('Ctrl Pts',(-3.80293430182523,2.33786765727141,4.50368049484103));
#17195=CARTESIAN_POINT('Ctrl Pts',(-3.76226114657918,2.53679940854407,4.49256670578423));
#17196=CARTESIAN_POINT('Ctrl Pts',(-3.57306852864947,2.61051711444195,4.48145291672742));
#17197=CARTESIAN_POINT('Ctrl Pts',(-3.40852658196552,2.49154610870105,4.47033912767061));
#17198=CARTESIAN_POINT('Ctrl Pts',(-3.41924244609765,2.28878193021138,4.45922533861382));
#17199=CARTESIAN_POINT('Ctrl Pts',(-3.5954077095353,2.18781687475719,4.44811154955701));
#17200=CARTESIAN_POINT('Ctrl Pts',(-3.77577642802961,2.28106551532598,4.43699776050021));
#17201=CARTESIAN_POINT('Ctrl Pts',(-3.79525482929664,2.48317608801675,4.4258839714434));
#17202=CARTESIAN_POINT('Ctrl Pts',(-3.6360145897577,2.60915494542926,4.4147701823866));
#17203=CARTESIAN_POINT('Ctrl Pts',(-3.44380914946703,2.54369130588911,4.40365639332979));
#17204=CARTESIAN_POINT('Ctrl Pts',(-3.39456824409026,2.34670659273357,4.39254260427299));
#17205=CARTESIAN_POINT('Ctrl Pts',(-3.53335879551641,2.19849952038487,4.38142881521618));
#17206=CARTESIAN_POINT('Ctrl Pts',(-3.73315192133567,2.23473296627504,4.37031502615938));
#17207=CARTESIAN_POINT('Ctrl Pts',(-3.81105932334871,2.4222275030731,4.35920123710257));
#17208=CARTESIAN_POINT('Ctrl Pts',(-3.69580227747518,2.58939637532595,4.34808744804577));
#17209=CARTESIAN_POINT('Ctrl Pts',(-3.49281517917073,2.58316970871533,4.33697365898897));
#17210=CARTESIAN_POINT('Ctrl Pts',(-3.38801801175539,2.40936362032424,4.32585986993216));
#17211=CARTESIAN_POINT('Ctrl Pts',(-3.47708428355003,2.22683063907596,4.31474608087536));
#17212=CARTESIAN_POINT('Ctrl Pts',(-3.67900086652888,2.20311869118934,4.30363229181856));
#17213=CARTESIAN_POINT('Ctrl Pts',(-3.76479031853975,2.3069928942824,4.29622309911402));
#17214=CARTESIAN_POINT('Ctrl Pts',(-3.77623115053166,2.36559394454847,4.29251850276175));
#17215=CARTESIAN_POINT('Ctrl Pts',(-3.64298642568859,2.23904122513352,5.22244449171475));
#17216=CARTESIAN_POINT('Ctrl Pts',(-3.69650904770099,2.25333523436478,5.21873989536248));
#17217=CARTESIAN_POINT('Ctrl Pts',(-3.78724129001348,2.33931326491388,5.21133070265794));
#17218=CARTESIAN_POINT('Ctrl Pts',(-3.75253088002014,2.52472431243949,5.20021691360114));
#17219=CARTESIAN_POINT('Ctrl Pts',(-3.57793539445428,2.59563515581826,5.18910312454433));
#17220=CARTESIAN_POINT('Ctrl Pts',(-3.42367004762736,2.48764253337377,5.17798933548753));
#17221=CARTESIAN_POINT('Ctrl Pts',(-3.4307346156477,2.29934846267587,5.16687554643072));
#17222=CARTESIAN_POINT('Ctrl Pts',(-3.59276310781765,2.2032224269029,5.15576175737392));
#17223=CARTESIAN_POINT('Ctrl Pts',(-3.76139893017626,2.28718889057467,5.14464796831712));
#17224=CARTESIAN_POINT('Ctrl Pts',(-3.78231281136787,2.47442275264891,5.13353417926031));
#17225=CARTESIAN_POINT('Ctrl Pts',(-3.63634954853391,2.5935315757496,5.12242039020352));
#17226=CARTESIAN_POINT('Ctrl Pts',(-3.45711720940891,2.53550127459616,5.1113066011467));
#17227=CARTESIAN_POINT('Ctrl Pts',(-3.4086660712507,2.35344386065259,5.1001928120899));
#17228=CARTESIAN_POINT('Ctrl Pts',(-3.53534556618555,2.21400043804369,5.0890790230331));
#17229=CARTESIAN_POINT('Ctrl Pts',(-3.72120373880265,2.24480420972985,5.07796523397629));
#17230=CARTESIAN_POINT('Ctrl Pts',(-3.79612288401061,2.41766060518064,5.06685144491949));
#17231=CARTESIAN_POINT('Ctrl Pts',(-3.6915284647428,2.57435197006973,5.05573765586269));
#17232=CARTESIAN_POINT('Ctrl Pts',(-3.50315703593343,2.5714570386006,5.04462386680588));
#17233=CARTESIAN_POINT('Ctrl Pts',(-3.40342705430619,2.41162551570156,5.03351007774908));
#17234=CARTESIAN_POINT('Ctrl Pts',(-3.48362252720301,2.24115303619919,5.02239628869227));
#17235=CARTESIAN_POINT('Ctrl Pts',(-3.67033961674501,2.21607497923609,5.01128249963547));
#17236=CARTESIAN_POINT('Ctrl Pts',(-3.79267405938058,2.35934558206435,5.00016871057866));
#17237=CARTESIAN_POINT('Ctrl Pts',(-3.73865174939092,2.53982763346569,4.98905492152186));
#17238=CARTESIAN_POINT('Ctrl Pts',(-3.55771992126626,2.59232386680991,4.97794113246505));
#17239=CARTESIAN_POINT('Ctrl Pts',(-3.41548752844543,2.46878388345875,4.96682734340825));
#17240=CARTESIAN_POINT('Ctrl Pts',(-3.44214149347704,2.28228523166696,4.95571355435145));
#17241=CARTESIAN_POINT('Ctrl Pts',(-3.61328513970402,2.20353224223104,4.94459976529464));
#17242=CARTESIAN_POINT('Ctrl Pts',(-3.7722687469273,2.30460841961473,4.93348597623784));
#17243=CARTESIAN_POINT('Ctrl Pts',(-3.77357281641202,2.4929975923203,4.92237218718104));
#17244=CARTESIAN_POINT('Ctrl Pts',(-3.61600371859295,2.59626501412009,4.91125839812423));
#17245=CARTESIAN_POINT('Ctrl Pts',(-3.44378623564737,2.51988884269441,4.90014460906743));
#17246=CARTESIAN_POINT('Ctrl Pts',(-3.41455298280027,2.33377705392094,4.88903082001062));
#17247=CARTESIAN_POINT('Ctrl Pts',(-3.55506148790733,2.20827987871175,4.87791703095382));
#17248=CARTESIAN_POINT('Ctrl Pts',(-3.73670272277068,2.25826630477233,4.86680324189701));
#17249=CARTESIAN_POINT('Ctrl Pts',(-3.79321840516747,2.43798318944394,4.85568945284021));
#17250=CARTESIAN_POINT('Ctrl Pts',(-3.67287909006884,2.58293363005899,4.8445756637834));
#17251=CARTESIAN_POINT('Ctrl Pts',(-3.48583271732505,2.5604428444725,4.8334618747266));
#17252=CARTESIAN_POINT('Ctrl Pts',(-3.40328495315871,2.39109690379476,4.8223480856698));
#17253=CARTESIAN_POINT('Ctrl Pts',(-3.50079270226656,2.22990006804163,4.81123429661299));
#17254=CARTESIAN_POINT('Ctrl Pts',(-3.68910601607711,2.22439762907444,4.80012050755619));
#17255=CARTESIAN_POINT('Ctrl Pts',(-3.79585958284132,2.37962603168174,4.78900671849938));
#17256=CARTESIAN_POINT('Ctrl Pts',(-3.72334065223214,2.55350295854726,4.77789292944258));
#17257=CARTESIAN_POINT('Ctrl Pts',(-3.53792662385674,2.58687688661252,4.76677914038578));
#17258=CARTESIAN_POINT('Ctrl Pts',(-3.40932906062523,2.4492002810333,4.75566535132897));
#17259=CARTESIAN_POINT('Ctrl Pts',(-3.45525477055898,2.26649010025516,4.74455156227217));
#17260=CARTESIAN_POINT('Ctrl Pts',(-3.63366743052263,2.20598304481872,4.73343777321536));
#17261=CARTESIAN_POINT('Ctrl Pts',(-3.7812639095143,2.32306190876162,4.72232398415856));
#17262=CARTESIAN_POINT('Ctrl Pts',(-3.76294747645498,2.51056308015232,4.71121019510176));
#17263=CARTESIAN_POINT('Ctrl Pts',(-3.59548337024634,2.59686461040897,4.70009640604495));
#17264=CARTESIAN_POINT('Ctrl Pts',(-3.43215338647331,2.50297373016179,4.68898261698815));
#17265=CARTESIAN_POINT('Ctrl Pts',(-3.42245531157129,2.31482982689595,4.67786882793134));
#17266=CARTESIAN_POINT('Ctrl Pts',(-3.57526590348185,2.20464314896778,4.66675503887454));
#17267=CARTESIAN_POINT('Ctrl Pts',(-3.75071589443907,2.27326881228664,4.65564124981773));
#17268=CARTESIAN_POINT('Ctrl Pts',(-3.78821391798199,2.45789296894922,4.64452746076093));
#17269=CARTESIAN_POINT('Ctrl Pts',(-3.65343760790444,2.58952703458114,4.63341367170412));
#17270=CARTESIAN_POINT('Ctrl Pts',(-3.46974924928937,2.54768485607922,4.62229988264733));
#17271=CARTESIAN_POINT('Ctrl Pts',(-3.40528087994151,2.37066505394572,4.61118609359051));
#17272=CARTESIAN_POINT('Ctrl Pts',(-3.51904112945263,2.2204958606208,4.60007230453372));
#17273=CARTESIAN_POINT('Ctrl Pts',(-3.70690395130293,2.23462884177668,4.58895851547691));
#17274=CARTESIAN_POINT('Ctrl Pts',(-3.79691637417015,2.40012791950764,4.57784472642011));
#17275=CARTESIAN_POINT('Ctrl Pts',(-3.7066890065403,2.56550991102893,4.5667309373633));
#17276=CARTESIAN_POINT('Ctrl Pts',(-3.5188079813597,2.57939880404271,4.55561714830649));
#17277=CARTESIAN_POINT('Ctrl Pts',(-3.40524293147808,2.42908193706057,4.54450335924969));
#17278=CARTESIAN_POINT('Ctrl Pts',(-3.4699412353955,2.25214604354523,4.53338957019289));
#17279=CARTESIAN_POINT('Ctrl Pts',(-3.65368380095038,2.21054255261035,4.52227578113608));
#17280=CARTESIAN_POINT('Ctrl Pts',(-3.78828897582448,2.34235161294705,4.51116199207928));
#17281=CARTESIAN_POINT('Ctrl Pts',(-3.75055111349195,2.52692689356351,4.50004820302248));
#17282=CARTESIAN_POINT('Ctrl Pts',(-3.57501211420431,2.59532455339135,4.48893441396567));
#17283=CARTESIAN_POINT('Ctrl Pts',(-3.42234480097716,2.48493942568113,4.47782062490887));
#17284=CARTESIAN_POINT('Ctrl Pts',(-3.43228732456417,2.29680829576209,4.46670683585206));
#17285=CARTESIAN_POINT('Ctrl Pts',(-3.5957391251232,2.20312966817403,4.45559304679526));
#17286=CARTESIAN_POINT('Ctrl Pts',(-3.76309102655441,2.2896487577109,4.44447925773845));
#17287=CARTESIAN_POINT('Ctrl Pts',(-3.78116371408077,2.47717345113617,4.43336546868165));
#17288=CARTESIAN_POINT('Ctrl Pts',(-3.63341549535601,2.59406068914566,4.42225167962485));
#17289=CARTESIAN_POINT('Ctrl Pts',(-3.4550811025268,2.53332141770711,4.41113789056804));
#17290=CARTESIAN_POINT('Ctrl Pts',(-3.40939380590581,2.35055266171297,4.40002410151124));
#17291=CARTESIAN_POINT('Ctrl Pts',(-3.53816814591191,2.21304137056363,4.38891031245443));
#17292=CARTESIAN_POINT('Ctrl Pts',(-3.72354263755246,2.2466599276823,4.37779652339763));
#17293=CARTESIAN_POINT('Ctrl Pts',(-3.79582763226376,2.42062339265036,4.36668273434082));
#17294=CARTESIAN_POINT('Ctrl Pts',(-3.68888843603675,2.57572805195694,4.35556894528402));
#17295=CARTESIAN_POINT('Ctrl Pts',(-3.50055047393982,2.56995075029642,4.34445515622722));
#17296=CARTESIAN_POINT('Ctrl Pts',(-3.40331628955371,2.40868786826575,4.33334136717041));
#17297=CARTESIAN_POINT('Ctrl Pts',(-3.4859548427499,2.23932789420368,4.32222757811361));
#17298=CARTESIAN_POINT('Ctrl Pts',(-3.67329954627769,2.21732718588468,4.3111137890568));
#17299=CARTESIAN_POINT('Ctrl Pts',(-3.75289776062778,2.31370501427084,4.30370459635227));
#17300=CARTESIAN_POINT('Ctrl Pts',(-3.76351293272515,2.3680769545372,4.3));
#17301=CARTESIAN_POINT('Ctrl Pts',(-3.76638442018051,2.4000942147675,5.13785196366098));
#17302=CARTESIAN_POINT('Ctrl Pts',(-3.76649613151981,2.42168271873493,5.13641270219409));
#17303=CARTESIAN_POINT('Ctrl Pts',(-3.76259704654914,2.44323253526348,5.1349734407272));
#17304=CARTESIAN_POINT('Ctrl Pts',(-3.75449995403028,2.46306857948665,5.13353417926031));
#17305=CARTESIAN_POINT('Ctrl Pts',(-3.73365839042322,2.51412569368247,5.12982958290804));
#17306=CARTESIAN_POINT('Ctrl Pts',(-3.68500396947857,2.55382863471604,5.12612498655578));
#17307=CARTESIAN_POINT('Ctrl Pts',(-3.63080470248541,2.56400838837391,5.12242039020351));
#17308=CARTESIAN_POINT('Ctrl Pts',(-3.57660543549225,2.57418814203179,5.11871579385124));
#17309=CARTESIAN_POINT('Ctrl Pts',(-3.51686132245058,2.55484470831398,5.11501119749897));
#17310=CARTESIAN_POINT('Ctrl Pts',(-3.47891407623671,2.51483008913114,5.1113066011467));
#17311=CARTESIAN_POINT('Ctrl Pts',(-3.44096683002284,2.47481546994831,5.10760200479444));
#17312=CARTESIAN_POINT('Ctrl Pts',(-3.42481645063677,2.41412966530045,5.10389740844217));
#17313=CARTESIAN_POINT('Ctrl Pts',(-3.43785451009954,2.3605461925417,5.1001928120899));
#17314=CARTESIAN_POINT('Ctrl Pts',(-3.45089256956232,2.30696271978295,5.09648821573763));
#17315=CARTESIAN_POINT('Ctrl Pts',(-3.49311906787393,2.26048157891332,5.09278361938537));
#17316=CARTESIAN_POINT('Ctrl Pts',(-3.54520867913259,2.2423749704262,5.0890790230331));
#17317=CARTESIAN_POINT('Ctrl Pts',(-3.59729829039125,2.22426836193908,5.08537442668083));
#17318=CARTESIAN_POINT('Ctrl Pts',(-3.65925101459695,2.23453628583446,5.08166983032856));
#17319=CARTESIAN_POINT('Ctrl Pts',(-3.70271390090113,2.26847964702395,5.07796523397629));
#17320=CARTESIAN_POINT('Ctrl Pts',(-3.74226404132859,2.29936725748381,5.07459414387119));
#17321=CARTESIAN_POINT('Ctrl Pts',(-3.76650358790754,2.34985942080815,5.07122305376608));
#17322=CARTESIAN_POINT('Ctrl Pts',(-3.76682061973634,2.40008640134019,5.06785196366098));
#17323=CARTESIAN_POINT('Ctrl Pts',(-3.65301702171886,2.20148256743283,5.2));
#17324=CARTESIAN_POINT('Ctrl Pts',(-3.66542047547214,2.20607510650608,5.2));
#17325=CARTESIAN_POINT('Ctrl Pts',(-3.67726977303962,2.21193437262237,5.2));
#17326=CARTESIAN_POINT('Ctrl Pts',(-3.688447163997,2.21889712590693,5.2));
#17327=CARTESIAN_POINT('Ctrl Pts',(-3.69411334108481,2.22242676831449,5.2));
#17328=CARTESIAN_POINT('Ctrl Pts',(-3.69960641439008,2.22624073198774,5.2));
#17329=CARTESIAN_POINT('Ctrl Pts',(-3.70490760860864,2.23032132776193,5.2));
#17330=CARTESIAN_POINT('Ctrl Pts',(-3.70949455661916,2.2338521323121,5.2));
#17331=CARTESIAN_POINT('Ctrl Pts',(-3.71393782222619,2.23758261370384,5.2));
#17332=CARTESIAN_POINT('Ctrl Pts',(-3.71822343533123,2.24150219834368,5.2));
#17333=CARTESIAN_POINT('Ctrl Pts',(-3.72133392659836,2.24434702672511,5.2));
#17334=CARTESIAN_POINT('Ctrl Pts',(-3.72435518261367,2.24728605527231,5.2));
#17335=CARTESIAN_POINT('Ctrl Pts',(-3.72727779974184,2.25030906336475,5.2));
#17336=CARTESIAN_POINT('Ctrl Pts',(-3.73622279642463,2.25956131782473,5.2));
#17337=CARTESIAN_POINT('Ctrl Pts',(-3.74426351405243,2.26961342426582,5.2));
#17338=CARTESIAN_POINT('Ctrl Pts',(-3.75126091239845,2.28033434366482,5.2));
#17339=CARTESIAN_POINT('Ctrl Pts',(-3.75579176664188,2.28727619844431,5.2));
#17340=CARTESIAN_POINT('Ctrl Pts',(-3.75988435832116,2.29449904020269,5.2));
#17341=CARTESIAN_POINT('Ctrl Pts',(-3.76348920729151,2.30196994667654,5.2));
#17342=CARTESIAN_POINT('Ctrl Pts',(-3.76515597383801,2.30542425421759,5.2));
#17343=CARTESIAN_POINT('Ctrl Pts',(-3.76671433719502,2.30892350560647,5.2));
#17344=CARTESIAN_POINT('Ctrl Pts',(-3.76815916520543,2.31246074610162,5.2));
#17345=CARTESIAN_POINT('Ctrl Pts',(-3.77216128940432,2.32225878135629,5.2));
#17346=CARTESIAN_POINT('Ctrl Pts',(-3.77529844536059,2.33235630265294,5.2));
#17347=CARTESIAN_POINT('Ctrl Pts',(-3.77747651815115,2.34267992422407,5.2));
#17348=CARTESIAN_POINT('Ctrl Pts',(-3.77933030902448,2.35146651553144,5.2));
#17349=CARTESIAN_POINT('Ctrl Pts',(-3.78048860368035,2.36041737528633,5.2));
#17350=CARTESIAN_POINT('Ctrl Pts',(-3.78096403138949,2.36945420421056,5.2));
#17351=CARTESIAN_POINT('Ctrl Pts',(-3.781133173515,2.37266922180987,5.2));
#17352=CARTESIAN_POINT('Ctrl Pts',(-3.78121552286205,2.37589368165894,5.2));
#17353=CARTESIAN_POINT('Ctrl Pts',(-3.78121200959806,2.37911434872485,5.2));
#17354=CARTESIAN_POINT('Ctrl Pts',(-3.78119923720175,2.3908230151512,5.2));
#17355=CARTESIAN_POINT('Ctrl Pts',(-3.78005717470715,2.40251790081025,5.2));
#17356=CARTESIAN_POINT('Ctrl Pts',(-3.77783120806398,2.41402669258654,5.2));
#17357=CARTESIAN_POINT('Ctrl Pts',(-3.77668819949671,2.41993632633585,5.2));
#17358=CARTESIAN_POINT('Ctrl Pts',(-3.77525870411221,2.42579670928221,5.2));
#17359=CARTESIAN_POINT('Ctrl Pts',(-3.77354493887783,2.43158224657623,5.2));
#17360=CARTESIAN_POINT('Ctrl Pts',(-3.77185769889076,2.43727823671147,5.2));
#17361=CARTESIAN_POINT('Ctrl Pts',(-3.7698921652597,2.44290711736645,5.2));
#17362=CARTESIAN_POINT('Ctrl Pts',(-3.76766231085216,2.44841156899725,5.2));
#17363=CARTESIAN_POINT('Ctrl Pts',(-3.76420558690842,2.45694457890368,5.2));
#17364=CARTESIAN_POINT('Ctrl Pts',(-3.7601120066452,2.46519219654187,5.2));
#17365=CARTESIAN_POINT('Ctrl Pts',(-3.75539091261074,2.47305855746262,5.2));
#17366=CARTESIAN_POINT('Ctrl Pts',(-3.75297690030925,2.47708082261811,5.2));
#17367=CARTESIAN_POINT('Ctrl Pts',(-3.75039789825265,2.48100349927224,5.2));
#17368=CARTESIAN_POINT('Ctrl Pts',(-3.74766394598163,2.48480007876844,5.2));
#17369=CARTESIAN_POINT('Ctrl Pts',(-3.74222934299289,2.49234699262488,5.2));
#17370=CARTESIAN_POINT('Ctrl Pts',(-3.73617584476421,2.49941040205976,5.2));
#17371=CARTESIAN_POINT('Ctrl Pts',(-3.7295081017749,2.50587917960273,5.2));
#17372=CARTESIAN_POINT('Ctrl Pts',(-3.72872963243595,2.50663441941712,5.2));
#17373=CARTESIAN_POINT('Ctrl Pts',(-3.72794277607053,2.50738152833223,5.2));
#17374=CARTESIAN_POINT('Ctrl Pts',(-3.72714768981588,2.50812044061668,5.2));
#17375=CARTESIAN_POINT('Origin',(-3.6,2.4,4.7));
#17376=CARTESIAN_POINT('Origin',(-3.6,-2.4,4.3));
#17377=CARTESIAN_POINT('Ctrl Pts',(-3.76351293272515,-2.4319230454628,4.3));
#17378=CARTESIAN_POINT('Ctrl Pts',(-3.76286871316703,-2.44021936733959,
4.3));
#17379=CARTESIAN_POINT('Ctrl Pts',(-3.76155560816075,-2.4484297641735,4.3));
#17380=CARTESIAN_POINT('Ctrl Pts',(-3.75963220162413,-2.45650290122813,
4.3));
#17381=CARTESIAN_POINT('Ctrl Pts',(-3.75857027465495,-2.46096013988305,
4.3));
#17382=CARTESIAN_POINT('Ctrl Pts',(-3.75732202640333,-2.4653756041272,4.3));
#17383=CARTESIAN_POINT('Ctrl Pts',(-3.75589532148576,-2.46974082414556,
4.3));
#17384=CARTESIAN_POINT('Ctrl Pts',(-3.75435560354459,-2.47445182464518,
4.3));
#17385=CARTESIAN_POINT('Ctrl Pts',(-3.75261043098936,-2.47909640157799,
4.3));
#17386=CARTESIAN_POINT('Ctrl Pts',(-3.75067343320617,-2.48365784346818,
4.3));
#17387=CARTESIAN_POINT('Ctrl Pts',(-3.74745266086646,-2.49124244991258,
4.3));
#17388=CARTESIAN_POINT('Ctrl Pts',(-3.74370038620747,-2.49860287239871,
4.3));
#17389=CARTESIAN_POINT('Ctrl Pts',(-3.73945960595045,-2.50569089060563,
4.3));
#17390=CARTESIAN_POINT('Ctrl Pts',(-3.73760643937826,-2.50878826363795,
4.3));
#17391=CARTESIAN_POINT('Ctrl Pts',(-3.73566012601582,-2.511832700902,4.3));
#17392=CARTESIAN_POINT('Ctrl Pts',(-3.73363013483138,-2.51481171247594,
4.3));
#17393=CARTESIAN_POINT('Ctrl Pts',(-3.72675413466501,-2.52490224106299,
4.3));
#17394=CARTESIAN_POINT('Ctrl Pts',(-3.71890630233768,-2.53427022723708,
4.3));
#17395=CARTESIAN_POINT('Ctrl Pts',(-3.710220437496,-2.54276718643201,4.3));
#17396=CARTESIAN_POINT('Ctrl Pts',(-3.70599062580354,-2.54690500552178,
4.3));
#17397=CARTESIAN_POINT('Ctrl Pts',(-3.70156129932866,-2.55083607679561,
4.3));
#17398=CARTESIAN_POINT('Ctrl Pts',(-3.69694397352711,-2.55454119955382,
4.3));
#17399=CARTESIAN_POINT('Ctrl Pts',(-3.69303800092373,-2.55767550469228,
4.3));
#17400=CARTESIAN_POINT('Ctrl Pts',(-3.68899293859581,-2.56065058734466,
4.3));
#17401=CARTESIAN_POINT('Ctrl Pts',(-3.68484116924407,-2.56343733372212,
4.3));
#17402=CARTESIAN_POINT('Ctrl Pts',(-3.67976588279258,-2.56684396230261,
4.3));
#17403=CARTESIAN_POINT('Ctrl Pts',(-3.67452566755957,-2.56997445255576,
4.3));
#17404=CARTESIAN_POINT('Ctrl Pts',(-3.66913578324553,-2.57281068802155,
4.3));
#17405=CARTESIAN_POINT('Ctrl Pts',(-3.66156268589167,-2.57679576192101,
4.3));
#17406=CARTESIAN_POINT('Ctrl Pts',(-3.6536944302201,-2.58020053259861,4.3));
#17407=CARTESIAN_POINT('Ctrl Pts',(-3.64559780863821,-2.58304072868827,
4.3));
#17408=CARTESIAN_POINT('Ctrl Pts',(-3.63968764062526,-2.58511394353595,
4.3));
#17409=CARTESIAN_POINT('Ctrl Pts',(-3.633655561192,-2.58688612240617,4.3));
#17410=CARTESIAN_POINT('Ctrl Pts',(-3.6275253141649,-2.58835973744293,4.3));
#17411=CARTESIAN_POINT('Ctrl Pts',(-3.62399736219549,-2.58920780164787,
4.3));
#17412=CARTESIAN_POINT('Ctrl Pts',(-3.62044138799033,-2.58995568069818,
4.3));
#17413=CARTESIAN_POINT('Ctrl Pts',(-3.61687019594187,-2.59060310935882,
4.3));
#17414=CARTESIAN_POINT('Ctrl Pts',(-3.6053532973959,-2.59269103129053,4.3));
#17415=CARTESIAN_POINT('Ctrl Pts',(-3.5936552916365,-2.5937426794922,4.3));
#17416=CARTESIAN_POINT('Ctrl Pts',(-3.58193296271379,-2.5937913460953,4.3));
#17417=CARTESIAN_POINT('Ctrl Pts',(-3.57526861453522,-2.59381901390686,
4.3));
#17418=CARTESIAN_POINT('Ctrl Pts',(-3.56859601622939,-2.59352191446421,
4.3));
#17419=CARTESIAN_POINT('Ctrl Pts',(-3.56194230797419,-2.5929013482942,4.3));
#17420=CARTESIAN_POINT('Ctrl Pts',(-3.55784543918526,-2.59251924885793,
4.3));
#17421=CARTESIAN_POINT('Ctrl Pts',(-3.55375366053793,-2.59201412364595,
4.3));
#17422=CARTESIAN_POINT('Ctrl Pts',(-3.54967980921583,-2.59138661988454,
4.3));
#17423=CARTESIAN_POINT('Ctrl Pts',(-3.53642388866962,-2.5893447829725,4.3));
#17424=CARTESIAN_POINT('Ctrl Pts',(-3.52344434481125,-2.58602557270852,
4.3));
#17425=CARTESIAN_POINT('Ctrl Pts',(-3.51095537008143,-2.58146161840675,
4.3));
#17426=CARTESIAN_POINT('Ctrl Pts',(-3.50062243383895,-2.57768556394,4.3));
#17427=CARTESIAN_POINT('Ctrl Pts',(-3.49062430896861,-2.57305657702062,
4.3));
#17428=CARTESIAN_POINT('Ctrl Pts',(-3.48108410771908,-2.56756616374223,
4.3));
#17429=CARTESIAN_POINT('Ctrl Pts',(-3.47992982857924,-2.56690187277492,
4.3));
#17430=CARTESIAN_POINT('Ctrl Pts',(-3.47878226433178,-2.56622494144235,
4.3));
#17431=CARTESIAN_POINT('Ctrl Pts',(-3.47764149510761,-2.56553553810743,
4.3));
#17432=CARTESIAN_POINT('Ctrl Pts',(-3.41173724903364,-2.48232321801034,
4.3));
#17433=CARTESIAN_POINT('Ctrl Pts',(-3.40908132671273,-2.474270631223,4.3));
#17434=CARTESIAN_POINT('Ctrl Pts',(-3.40697195813618,-2.46606039521676,
4.3));
#17435=CARTESIAN_POINT('Ctrl Pts',(-3.40539675699364,-2.45774386680553,
4.3));
#17436=CARTESIAN_POINT('Ctrl Pts',(-3.40421043018009,-2.45148046311471,
4.3));
#17437=CARTESIAN_POINT('Ctrl Pts',(-3.40332727350005,-2.44515671203471,
4.3));
#17438=CARTESIAN_POINT('Ctrl Pts',(-3.40274510705531,-2.43879482091291,
4.3));
#17439=CARTESIAN_POINT('Ctrl Pts',(-3.40230912033401,-2.4340303758362,4.3));
#17440=CARTESIAN_POINT('Ctrl Pts',(-3.40204240567473,-2.42924590842869,
4.3));
#17441=CARTESIAN_POINT('Ctrl Pts',(-3.40194407560279,-2.42446300988855,
4.3));
#17442=CARTESIAN_POINT('Ctrl Pts',(-3.4017383892304,-2.41445816568562,4.3));
#17443=CARTESIAN_POINT('Ctrl Pts',(-3.40226690961593,-2.40444523502109,
4.3));
#17444=CARTESIAN_POINT('Ctrl Pts',(-3.40352193796024,-2.39451254861871,
4.3));
#17445=CARTESIAN_POINT('Ctrl Pts',(-3.40417749889618,-2.3893242345667,4.3));
#17446=CARTESIAN_POINT('Ctrl Pts',(-3.4050325722576,-2.38415490381948,4.3));
#17447=CARTESIAN_POINT('Ctrl Pts',(-3.40608153527603,-2.37904223030681,
4.3));
#17448=CARTESIAN_POINT('Ctrl Pts',(-3.40864847953637,-2.36653087604773,
4.3));
#17449=CARTESIAN_POINT('Ctrl Pts',(-3.41237572714265,-2.35432631626979,
4.3));
#17450=CARTESIAN_POINT('Ctrl Pts',(-3.41724961050618,-2.34261710559519,
4.3));
#17451=CARTESIAN_POINT('Ctrl Pts',(-3.41948718042203,-2.33724147889476,
4.3));
#17452=CARTESIAN_POINT('Ctrl Pts',(-3.42196704076708,-2.33197060519316,
4.3));
#17453=CARTESIAN_POINT('Ctrl Pts',(-3.42469079211682,-2.32682518779718,
4.3));
#17454=CARTESIAN_POINT('Ctrl Pts',(-3.42647141933207,-2.32346141883567,
4.3));
#17455=CARTESIAN_POINT('Ctrl Pts',(-3.42835738874669,-2.3201495667824,4.3));
#17456=CARTESIAN_POINT('Ctrl Pts',(-3.430346105223,-2.31690145647487,4.3));
#17457=CARTESIAN_POINT('Ctrl Pts',(-3.43461852095602,-2.30992344943073,
4.3));
#17458=CARTESIAN_POINT('Ctrl Pts',(-3.43934738846969,-2.3032660957291,4.3));
#17459=CARTESIAN_POINT('Ctrl Pts',(-3.44453058590951,-2.29698173842211,
4.3));
#17460=CARTESIAN_POINT('Ctrl Pts',(-3.4502359337428,-2.29006430092116,4.3));
#17461=CARTESIAN_POINT('Ctrl Pts',(-3.45649195144988,-2.28359849259699,
4.3));
#17462=CARTESIAN_POINT('Ctrl Pts',(-3.4632263722909,-2.27761731307503,4.3));
#17463=CARTESIAN_POINT('Ctrl Pts',(-3.46747035511976,-2.27384801742411,
4.3));
#17464=CARTESIAN_POINT('Ctrl Pts',(-3.47190450284819,-2.27027143263625,
4.3));
#17465=CARTESIAN_POINT('Ctrl Pts',(-3.47651159455371,-2.26689859050011,
4.3));
#17466=CARTESIAN_POINT('Ctrl Pts',(-3.4793251060266,-2.26483882467541,4.3));
#17467=CARTESIAN_POINT('Ctrl Pts',(-3.48219970787858,-2.26285776645565,
4.3));
#17468=CARTESIAN_POINT('Ctrl Pts',(-3.48512436737332,-2.26096157786103,
4.3));
#17469=CARTESIAN_POINT('Ctrl Pts',(-3.49373619954507,-2.25537813884111,
4.3));
#17470=CARTESIAN_POINT('Ctrl Pts',(-3.50279847994849,-2.25051611152294,
4.3));
#17471=CARTESIAN_POINT('Ctrl Pts',(-3.51220227087042,-2.24642657080492,
4.3));
#17472=CARTESIAN_POINT('Ctrl Pts',(-3.5210281717619,-2.24258834413989,4.3));
#17473=CARTESIAN_POINT('Ctrl Pts',(-3.53015556945347,-2.23943063412497,
4.3));
#17474=CARTESIAN_POINT('Ctrl Pts',(-3.53949489532435,-2.23701751505981,
4.3));
#17475=CARTESIAN_POINT('Ctrl Pts',(-3.54298225084135,-2.23611644316218,
4.3));
#17476=CARTESIAN_POINT('Ctrl Pts',(-3.54649061678302,-2.23532167500438,
4.3));
#17477=CARTESIAN_POINT('Ctrl Pts',(-3.5500119948057,-2.23463615769257,4.3));
#17478=CARTESIAN_POINT('Ctrl Pts',(-3.5610932074021,-2.23247894451586,4.3));
#17479=CARTESIAN_POINT('Ctrl Pts',(-3.57231428638466,-2.23139729676061,
4.3));
#17480=CARTESIAN_POINT('Ctrl Pts',(-3.58352462409827,-2.2314877485142,4.3));
#17481=CARTESIAN_POINT('Ctrl Pts',(-3.58970653876345,-2.23153762792339,
4.3));
#17482=CARTESIAN_POINT('Ctrl Pts',(-3.59588508216706,-2.23194477463139,
4.3));
#17483=CARTESIAN_POINT('Ctrl Pts',(-3.60203269161667,-2.23273189903069,
4.3));
#17484=CARTESIAN_POINT('Ctrl Pts',(-3.60310835631345,-2.23286962442383,
4.3));
#17485=CARTESIAN_POINT('Ctrl Pts',(-3.60418306761235,-2.23301899515145,
4.3));
#17486=CARTESIAN_POINT('Ctrl Pts',(-3.60525667255607,-2.23317994016621,
4.3));
#17487=CARTESIAN_POINT('Origin',(-3.6,-2.4,5.35459252805377));
#17488=CARTESIAN_POINT('Ctrl Pts',(-3.80565733457988,-2.39985006589818,
5.17959252805377));
#17489=CARTESIAN_POINT('Ctrl Pts',(-3.8057391516022,-2.39002097154438,5.17905813053169));
#17490=CARTESIAN_POINT('Ctrl Pts',(-3.80062938506941,-2.31213685567809,
5.17481913665734));
#17491=CARTESIAN_POINT('Ctrl Pts',(-3.70109554203788,-2.17915701647198,
5.16687554643073));
#17492=CARTESIAN_POINT('Ctrl Pts',(-3.46929950206046,-2.19531102353728,
5.15576175737392));
#17493=CARTESIAN_POINT('Ctrl Pts',(-3.35713783153282,-2.39878694399818,
5.14464796831711));
#17494=CARTESIAN_POINT('Ctrl Pts',(-3.46726929886284,-2.60338928299931,
5.13353417926032));
#17495=CARTESIAN_POINT('Ctrl Pts',(-3.69889136100131,-2.62181906697108,
5.12242039020351));
#17496=CARTESIAN_POINT('Ctrl Pts',(-3.80021578451737,-2.48926235936684,
5.11443983980133));
#17497=CARTESIAN_POINT('Ctrl Pts',(-3.80572902589707,-2.41067410853188,
5.11016388575141));
#17498=CARTESIAN_POINT('Ctrl Pts',(-3.8056388038084,-2.40016037433918,5.10959252805377));
#17499=CARTESIAN_POINT('Ctrl Pts',(-3.80526708169851,-2.40022955265959,
5.18540747194623));
#17500=CARTESIAN_POINT('Ctrl Pts',(-3.80491230300414,-2.3532097525552,5.18286245525962));
#17501=CARTESIAN_POINT('Ctrl Pts',(-3.76565541968849,-2.23704708335906,
5.17661284222073));
#17502=CARTESIAN_POINT('Ctrl Pts',(-3.5727867642971,-2.15871465280967,5.16665863282959));
#17503=CARTESIAN_POINT('Ctrl Pts',(-3.38252461999799,-2.29190667528476,
5.15554484377278));
#17504=CARTESIAN_POINT('Ctrl Pts',(-3.39123766053156,-2.52413789941101,
5.14443105471598));
#17505=CARTESIAN_POINT('Ctrl Pts',(-3.59107442597796,-2.64269432067786,
5.13331726565918));
#17506=CARTESIAN_POINT('Ctrl Pts',(-3.77212564872883,-2.55254602634109,
5.12364273806926));
#17507=CARTESIAN_POINT('Ctrl Pts',(-3.80499226553068,-2.44179202539712,
5.11767280683161));
#17508=CARTESIAN_POINT('Ctrl Pts',(-3.80520912268496,-2.39988380060309,
5.11540747194623));
#17509=CARTESIAN_POINT('Ctrl Pts',(-3.47309291201476,-2.29206413469515,
5.2));
#17510=CARTESIAN_POINT('Ctrl Pts',(-3.43720166889934,-2.33426376069605,
5.19629540364773));
#17511=CARTESIAN_POINT('Ctrl Pts',(-3.4114791580674,-2.45658678033172,5.1888862109432));
#17512=CARTESIAN_POINT('Ctrl Pts',(-3.54548746492724,-2.5893415011903,5.17777242188639));
#17513=CARTESIAN_POINT('Ctrl Pts',(-3.72942274690437,-2.54835673318009,
5.16665863282959));
#17514=CARTESIAN_POINT('Ctrl Pts',(-3.79487861290014,-2.37179020383286,
5.15554484377278));
#17515=CARTESIAN_POINT('Ctrl Pts',(-3.68196869353212,-2.22093957388603,
5.14443105471598));
#17516=CARTESIAN_POINT('Ctrl Pts',(-3.49402748287272,-2.23403731121212,
5.13331726565918));
#17517=CARTESIAN_POINT('Ctrl Pts',(-3.40308632550611,-2.39901644905753,
5.12220347660237));
#17518=CARTESIAN_POINT('Ctrl Pts',(-3.49238138552402,-2.56490889182472,
5.11108968754557));
#17519=CARTESIAN_POINT('Ctrl Pts',(-3.68018153421496,-2.57985183870243,
5.09997589848876));
#17520=CARTESIAN_POINT('Ctrl Pts',(-3.79459034046341,-2.43017761257843,
5.08886210943196));
#17521=CARTESIAN_POINT('Ctrl Pts',(-3.73088853854501,-2.25287985005212,
5.07774832037516));
#17522=CARTESIAN_POINT('Ctrl Pts',(-3.5473829043692,-2.21024364094684,5.06663453131835));
#17523=CARTESIAN_POINT('Ctrl Pts',(-3.41203832877697,-2.34129317389102,
5.05552074226154));
#17524=CARTESIAN_POINT('Ctrl Pts',(-3.44873718538878,-2.52607793299967,
5.04440695320475));
#17525=CARTESIAN_POINT('Ctrl Pts',(-3.62388862018941,-2.59546202911018,
5.03329316414794));
#17526=CARTESIAN_POINT('Ctrl Pts',(-3.77717452575129,-2.48593756377701,
5.02217937509113));
#17527=CARTESIAN_POINT('Ctrl Pts',(-3.76829058072669,-2.29775344650504,
5.01106558603433));
#17528=CARTESIAN_POINT('Ctrl Pts',(-3.6053683575545,-2.20315677179449,4.99995179697753));
#17529=CARTESIAN_POINT('Ctrl Pts',(-3.43753241636245,-2.28873292992563,
4.98883800792072));
#17530=CARTESIAN_POINT('Ctrl Pts',(-3.41840489671633,-2.47615310229093,
4.97772421886392));
#17531=CARTESIAN_POINT('Ctrl Pts',(-3.56549343466676,-2.59386947492594,
4.96661042980711));
#17532=CARTESIAN_POINT('Ctrl Pts',(-3.74416622313161,-2.53413491931517,
4.95549664075031));
#17533=CARTESIAN_POINT('Ctrl Pts',(-3.79088203264097,-2.35162515047058,
4.9443828516935));
#17534=CARTESIAN_POINT('Ctrl Pts',(-3.66288135290806,-2.21339343020375,
4.9332690626367));
#17535=CARTESIAN_POINT('Ctrl Pts',(-3.47732465774361,-2.24596481943629,
4.9221552735799));
#17536=CARTESIAN_POINT('Ctrl Pts',(-3.40405409457531,-2.41952635636528,
4.91104148452309));
#17537=CARTESIAN_POINT('Ctrl Pts',(-3.51013504082201,-2.57521519784486,
4.89992769546629));
#17538=CARTESIAN_POINT('Ctrl Pts',(-3.69847040334124,-2.57052758167369,
4.88881390640948));
#17539=CARTESIAN_POINT('Ctrl Pts',(-3.79667468895243,-2.40975413607622,
4.87770011735268));
#17540=CARTESIAN_POINT('Ctrl Pts',(-3.71486040132253,-2.24005261911178,
4.86658632829587));
#17541=CARTESIAN_POINT('Ctrl Pts',(-3.5279130857567,-2.2167527537995,4.85547253923907));
#17542=CARTESIAN_POINT('Ctrl Pts',(-3.40694774031892,-2.3611811711004,4.84435875018227));
#17543=CARTESIAN_POINT('Ctrl Pts',(-3.46268531752878,-2.5411409027282,4.83324496112546));
#17544=CARTESIAN_POINT('Ctrl Pts',(-3.64410858085897,-2.59191276544236,
4.82213117206866));
#17545=CARTESIAN_POINT('Ctrl Pts',(-3.7851587599036,-2.46702469750825,4.81101738301185));
#17546=CARTESIAN_POINT('Ctrl Pts',(-3.75673102616532,-2.28078816383312,
4.79990359395505));
#17547=CARTESIAN_POINT('Ctrl Pts',(-3.58484560672719,-2.20366757575568,
4.78878980489824));
#17548=CARTESIAN_POINT('Ctrl Pts',(-3.42683117531417,-2.30625228215021,
4.77767601584145));
#17549=CARTESIAN_POINT('Ctrl Pts',(-3.42732013300413,-2.49464533786407,
4.76656222678464));
#17550=CARTESIAN_POINT('Ctrl Pts',(-3.5858649312783,-2.59640844247982,4.75544843772783));
#17551=CARTESIAN_POINT('Ctrl Pts',(-3.75734771825602,-2.51839667227055,
4.74433464867103));
#17552=CARTESIAN_POINT('Ctrl Pts',(-3.78480835426951,-2.33201508522246,
4.73322085961423));
#17553=CARTESIAN_POINT('Ctrl Pts',(-3.64311180775084,-2.20786086167162,
4.72210707055742));
#17554=CARTESIAN_POINT('Ctrl Pts',(-3.46195453467666,-2.25957377043879,
4.71099328150062));
#17555=CARTESIAN_POINT('Ctrl Pts',(-3.407151841555,-2.43982039966509,4.69987949244381));
#17556=CARTESIAN_POINT('Ctrl Pts',(-3.52886525490491,-2.58361896548389,
4.68876570338701));
#17557=CARTESIAN_POINT('Ctrl Pts',(-3.71568910716324,-2.55934900981458,
4.6776519143302));
#17558=CARTESIAN_POINT('Ctrl Pts',(-3.79662140763134,-2.38922509832133,
4.6665381252734));
#17559=CARTESIAN_POINT('Ctrl Pts',(-3.69758390385606,-2.22896357653021,
4.65542433621659));
#17560=CARTESIAN_POINT('Ctrl Pts',(-3.50922674620458,-2.22525363282606,
4.64431054715979));
#17561=CARTESIAN_POINT('Ctrl Pts',(-3.40395537719079,-2.38149102075462,
4.63319675810299));
#17562=CARTESIAN_POINT('Ctrl Pts',(-3.47812587473144,-2.55466988729295,
4.62208296904618));
#17563=CARTESIAN_POINT('Ctrl Pts',(-3.66384914127714,-2.58627765191548,
4.61096917998938));
#17564=CARTESIAN_POINT('Ctrl Pts',(-3.79113056471305,-2.447383369209,4.59985539093257));
#17565=CARTESIAN_POINT('Ctrl Pts',(-3.74346801469971,-2.26511855129859,
4.58874160187577));
#17566=CARTESIAN_POINT('Ctrl Pts',(-3.56448756379251,-2.20631225305021,
4.57762781281896));
#17567=CARTESIAN_POINT('Ctrl Pts',(-3.41801204848697,-2.32479054614148,
4.56651402376216));
#17568=CARTESIAN_POINT('Ctrl Pts',(-3.43811216908,-2.51210890530657,4.55540023470536));
#17569=CARTESIAN_POINT('Ctrl Pts',(-3.60639005725709,-2.59681271199525,
4.54428644564855));
#17570=CARTESIAN_POINT('Ctrl Pts',(-3.76881905353834,-2.50137161148251,
4.53317265659175));
#17571=CARTESIAN_POINT('Ctrl Pts',(-3.77672605561821,-2.31314392515575,
4.52205886753495));
#17572=CARTESIAN_POINT('Ctrl Pts',(-3.62287369469976,-2.2044165895329,4.51094507847814));
#17573=CARTESIAN_POINT('Ctrl Pts',(-3.44808478177985,-2.27470896680823,
4.49983128942134));
#17574=CARTESIAN_POINT('Ctrl Pts',(-3.41234559060706,-2.45968164920097,
4.48871750036453));
#17575=CARTESIAN_POINT('Ctrl Pts',(-3.54836860914922,-2.5900270381604,4.47760371130773));
#17576=CARTESIAN_POINT('Ctrl Pts',(-3.73165042397165,-2.54643853021323,
4.46648992225092));
#17577=CARTESIAN_POINT('Ctrl Pts',(-3.79443111532907,-2.36881316247168,
4.45537613319412));
#17578=CARTESIAN_POINT('Ctrl Pts',(-3.67924679659355,-2.21973348556073,
4.44426234413731));
#17579=CARTESIAN_POINT('Ctrl Pts',(-3.49152699669547,-2.23565374410205,
4.43314855508051));
#17580=CARTESIAN_POINT('Ctrl Pts',(-3.40309374590592,-2.40200209374894,
4.4220347660237));
#17581=CARTESIAN_POINT('Ctrl Pts',(-3.49489106457482,-2.5665177055076,4.41092097696691));
#17582=CARTESIAN_POINT('Ctrl Pts',(-3.68289569971986,-2.57861817099917,
4.39980718791009));
#17583=CARTESIAN_POINT('Ctrl Pts',(-3.79502512928071,-2.42722660191142,
4.3886933988533));
#17584=CARTESIAN_POINT('Ctrl Pts',(-3.72864550893249,-2.25091581121659,
4.37757960979648));
#17585=CARTESIAN_POINT('Ctrl Pts',(-3.54451587080997,-2.21106027365159,
4.36646582073969));
#17586=CARTESIAN_POINT('Ctrl Pts',(-3.41117013277341,-2.34414980914689,
4.35535203168287));
#17587=CARTESIAN_POINT('Ctrl Pts',(-3.45066522211898,-2.5283468448043,4.34423824262609));
#17588=CARTESIAN_POINT('Ctrl Pts',(-3.62684270366593,-2.59509221455348,
4.33312445356927));
#17589=CARTESIAN_POINT('Ctrl Pts',(-3.77846161739066,-2.4832160890933,4.32201066451248));
#17590=CARTESIAN_POINT('Ctrl Pts',(-3.76671079422265,-2.29527426875025,
4.31089687545566));
#17591=CARTESIAN_POINT('Ctrl Pts',(-3.60241192612029,-2.2029822262702,4.29978308639886));
#17592=CARTESIAN_POINT('Ctrl Pts',(-3.43581020892599,-2.29144640006724,
4.28866929734205));
#17593=CARTESIAN_POINT('Ctrl Pts',(-3.42516046182893,-2.41599017382995,
4.28126010463752));
#17594=CARTESIAN_POINT('Ctrl Pts',(-3.44735576439472,-2.46674801372685,
4.27755550828525));
#17595=CARTESIAN_POINT('Ctrl Pts',(-3.46322193753412,-2.28366876301903,
5.20748149723825));
#17596=CARTESIAN_POINT('Ctrl Pts',(-3.42453903360214,-2.32915072287504,
5.20377690088598));
#17597=CARTESIAN_POINT('Ctrl Pts',(-3.39681579726281,-2.4609881630556,5.19636770818145));
#17598=CARTESIAN_POINT('Ctrl Pts',(-3.54124741930709,-2.60406869378488,
5.18525391912464));
#17599=CARTESIAN_POINT('Ctrl Pts',(-3.73948939213428,-2.55989608492554,
5.17414013006784));
#17600=CARTESIAN_POINT('Ctrl Pts',(-3.81003648820324,-2.36959601450513,
5.16302634101103));
#17601=CARTESIAN_POINT('Ctrl Pts',(-3.68834430970071,-2.20701205474802,
5.15191255195423));
#17602=CARTESIAN_POINT('Ctrl Pts',(-3.48578482260197,-2.22112854865384,
5.14079876289742));
#17603=CARTESIAN_POINT('Ctrl Pts',(-3.38777016084835,-2.39893994737108,
5.12968497384062));
#17604=CARTESIAN_POINT('Ctrl Pts',(-3.4840106899703,-2.57773568888292,5.11857118478382));
#17605=CARTESIAN_POINT('Ctrl Pts',(-3.68641814314374,-2.59384091479198,
5.10745739572701));
#17606=CARTESIAN_POINT('Ctrl Pts',(-3.8097257936157,-2.43252486085572,5.0963436066702));
#17607=CARTESIAN_POINT('Ctrl Pts',(-3.74106919467933,-2.2414366811261,5.08522981761341));
#17608=CARTESIAN_POINT('Ctrl Pts',(-3.54329028813742,-2.19548418024617,
5.0741160285566));
#17609=CARTESIAN_POINT('Ctrl Pts',(-3.39741846089223,-2.33672689164815,
5.06300223949979));
#17610=CARTESIAN_POINT('Ctrl Pts',(-3.43697179539676,-2.53588441488314,
5.051888450443));
#17611=CARTESIAN_POINT('Ctrl Pts',(-3.62574670364252,-2.61066528317513,
5.04077466138618));
#17612=CARTESIAN_POINT('Ctrl Pts',(-3.79095535746114,-2.4926218830884,5.02966087232938));
#17613=CARTESIAN_POINT('Ctrl Pts',(-3.78138040930963,-2.28980059583054,
5.01854708327258));
#17614=CARTESIAN_POINT('Ctrl Pts',(-3.60578591437709,-2.1878460865274,5.00743329421578));
#17615=CARTESIAN_POINT('Ctrl Pts',(-3.42489550697087,-2.28007845343676,
4.99631950515897));
#17616=CARTESIAN_POINT('Ctrl Pts',(-3.40428022756837,-2.48207637530325,
4.98520571610216));
#17617=CARTESIAN_POINT('Ctrl Pts',(-3.56280947562848,-2.60894885835481,
4.97409192704536));
#17618=CARTESIAN_POINT('Ctrl Pts',(-3.75537963234378,-2.54456808255722,
4.96297813798856));
#17619=CARTESIAN_POINT('Ctrl Pts',(-3.80572904948554,-2.34786250085983,
4.95186434893175));
#17620=CARTESIAN_POINT('Ctrl Pts',(-3.6677723344893,-2.19887896361545,4.94075055987495));
#17621=CARTESIAN_POINT('Ctrl Pts',(-3.46778283315333,-2.23398379173638,
4.92963677081814));
#17622=CARTESIAN_POINT('Ctrl Pts',(-3.38881320407234,-2.42104513808537,
4.91852298176134));
#17623=CARTESIAN_POINT('Ctrl Pts',(-3.50314524432732,-2.5888436308505,4.90740919270454));
#17624=CARTESIAN_POINT('Ctrl Pts',(-3.70612954085602,-2.58379140667882,
4.89629540364773));
#17625=CARTESIAN_POINT('Ctrl Pts',(-3.81197226504892,-2.41051282363117,
4.88518161459093));
#17626=CARTESIAN_POINT('Ctrl Pts',(-3.72379437111327,-2.22761173389364,
4.87406782553412));
#17627=CARTESIAN_POINT('Ctrl Pts',(-3.52230608537413,-2.20249957913754,
4.86295403647732));
#17628=CARTESIAN_POINT('Ctrl Pts',(-3.3919319208009,-2.35816179940478,4.85184024742052));
#17629=CARTESIAN_POINT('Ctrl Pts',(-3.45200482877115,-2.55211899915388,
4.84072645836371));
#17630=CARTESIAN_POINT('Ctrl Pts',(-3.64753939534654,-2.60683995383086,
4.82961266930691));
#17631=CARTESIAN_POINT('Ctrl Pts',(-3.79956061422784,-2.47223795304173,
4.8184988802501));
#17632=CARTESIAN_POINT('Ctrl Pts',(-3.7689217397351,-2.27151573459945,4.8073850911933));
#17633=CARTESIAN_POINT('Ctrl Pts',(-3.58366688116,-2.18839662138894,4.79627130213649));
#17634=CARTESIAN_POINT('Ctrl Pts',(-3.41336191148932,-2.29896048036668,
4.78515751307969));
#17635=CARTESIAN_POINT('Ctrl Pts',(-3.41388890085234,-2.50200695753087,
4.77404372402289));
#17636=CARTESIAN_POINT('Ctrl Pts',(-3.58476548990864,-2.61168530962949,
4.76292993496608));
#17637=CARTESIAN_POINT('Ctrl Pts',(-3.76958639882265,-2.52760569714953,
4.75181614590928));
#17638=CARTESIAN_POINT('Ctrl Pts',(-3.79918295365372,-2.32672714292159,
4.74070235685248));
#17639=CARTESIAN_POINT('Ctrl Pts',(-3.64646509211721,-2.19291606574822,
4.72958856779567));
#17640=CARTESIAN_POINT('Ctrl Pts',(-3.45121720481583,-2.24865126208706,
4.71847477873887));
#17641=CARTESIAN_POINT('Ctrl Pts',(-3.39215189725818,-2.44291767464904,
4.70736098968205));
#17642=CARTESIAN_POINT('Ctrl Pts',(-3.52333231529793,-2.59790105288522,
4.69624720062526));
#17643=CARTESIAN_POINT('Ctrl Pts',(-3.72468753461616,-2.57174335306496,
4.68513341156845));
#17644=CARTESIAN_POINT('Ctrl Pts',(-3.8119148394474,-2.38838701448227,4.67401962251165));
#17645=CARTESIAN_POINT('Ctrl Pts',(-3.70517408845471,-2.21566017324412,
4.66290583345485));
#17646=CARTESIAN_POINT('Ctrl Pts',(-3.50216630154411,-2.21166166599155,
4.65179204439804));
#17647=CARTESIAN_POINT('Ctrl Pts',(-3.38870680833984,-2.38005137175869,
4.64067825534123));
#17648=CARTESIAN_POINT('Ctrl Pts',(-3.46864636968979,-2.56670028318833,
4.62956446628443));
#17649=CARTESIAN_POINT('Ctrl Pts',(-3.66881539851434,-2.6007665349051,4.61845067722763));
#17650=CARTESIAN_POINT('Ctrl Pts',(-3.80599691265867,-2.45106890037747,
4.60733688817082));
#17651=CARTESIAN_POINT('Ctrl Pts',(-3.75462711648332,-2.25462732217041,
4.59622309911401));
#17652=CARTESIAN_POINT('Ctrl Pts',(-3.56172536699866,-2.1912470046255,4.58510931005722));
#17653=CARTESIAN_POINT('Ctrl Pts',(-3.4038568231667,-2.31894067115399,4.57399552100041));
#17654=CARTESIAN_POINT('Ctrl Pts',(-3.42552035349974,-2.5208288606763,4.56288173194361));
#17655=CARTESIAN_POINT('Ctrl Pts',(-3.60688708301913,-2.61212102367755,
4.5517679428868));
#17656=CARTESIAN_POINT('Ctrl Pts',(-3.78194998732446,-2.50925640819396,
4.54065415383));
#17657=CARTESIAN_POINT('Ctrl Pts',(-3.79047200482221,-2.30638816303176,
4.52954036477319));
#17658=CARTESIAN_POINT('Ctrl Pts',(-3.62465283611923,-2.18920389429099,
4.51842657571639));
#17659=CARTESIAN_POINT('Ctrl Pts',(-3.43626864710937,-2.2649636908672,4.50731278665958));
#17660=CARTESIAN_POINT('Ctrl Pts',(-3.39774962188927,-2.46432375426836,
4.49619899760278));
#17661=CARTESIAN_POINT('Ctrl Pts',(-3.54435266213177,-2.60480755258314,
4.48508520854598));
#17662=CARTESIAN_POINT('Ctrl Pts',(-3.74189034040202,-2.55782868199802,
4.47397141948917));
#17663=CARTESIAN_POINT('Ctrl Pts',(-3.80955418377328,-2.36638741555509,
4.46285763043236));
#17664=CARTESIAN_POINT('Ctrl Pts',(-3.68541070059029,-2.20571215553106,
4.45174384137557));
#17665=CARTESIAN_POINT('Ctrl Pts',(-3.4830898458282,-2.22287070949214,4.44063005231875));
#17666=CARTESIAN_POINT('Ctrl Pts',(-3.3877781584151,-2.40215781882795,4.42951626326196));
#17667=CARTESIAN_POINT('Ctrl Pts',(-3.48671557464955,-2.57946963788377,
4.41840247420515));
#17668=CARTESIAN_POINT('Ctrl Pts',(-3.68934341946097,-2.59251129104238,
4.40728868514835));
#17669=CARTESIAN_POINT('Ctrl Pts',(-3.81019440079089,-2.42934431729619,
4.39617489609154));
#17670=CARTESIAN_POINT('Ctrl Pts',(-3.73865169972831,-2.23931987716506,
4.38506110703474));
#17671=CARTESIAN_POINT('Ctrl Pts',(-3.54020025351852,-2.19636433155117,
4.37394731797794));
#17672=CARTESIAN_POINT('Ctrl Pts',(-3.39648273563768,-2.33980571917207,
4.36283352892113));
#17673=CARTESIAN_POINT('Ctrl Pts',(-3.43904979696867,-2.53832980517198,
4.35171973986433));
#17674=CARTESIAN_POINT('Ctrl Pts',(-3.6289305590181,-2.6102667040308,4.34060595080752));
#17675=CARTESIAN_POINT('Ctrl Pts',(-3.79234256052004,-2.48968872907629,
4.32949216175072));
#17676=CARTESIAN_POINT('Ctrl Pts',(-3.77967774525388,-2.28712858487203,
4.31837837269391));
#17677=CARTESIAN_POINT('Ctrl Pts',(-3.60259952841706,-2.18765796465806,
4.30726458363711));
#17678=CARTESIAN_POINT('Ctrl Pts',(-3.42303934432415,-2.28300298030457,
4.29615079458031));
#17679=CARTESIAN_POINT('Ctrl Pts',(-3.41156124805061,-2.41723390733863,
4.28874160187577));
#17680=CARTESIAN_POINT('Ctrl Pts',(-3.43548292594103,-2.47193974848801,
4.2850370055235));
#17681=CARTESIAN_POINT('Ctrl Pts',(-3.45335096305347,-2.2752733913429,5.2149629944765));
#17682=CARTESIAN_POINT('Ctrl Pts',(-3.41187639830495,-2.32403768505403,
5.21125839812423));
#17683=CARTESIAN_POINT('Ctrl Pts',(-3.38215243645823,-2.46538954577948,
5.20384920541969));
#17684=CARTESIAN_POINT('Ctrl Pts',(-3.53700737368693,-2.61879588637947,
5.19273541636289));
#17685=CARTESIAN_POINT('Ctrl Pts',(-3.74955603736419,-2.571435436671,5.18162162730609));
#17686=CARTESIAN_POINT('Ctrl Pts',(-3.82519436350635,-2.3674018251774,5.17050783824928));
#17687=CARTESIAN_POINT('Ctrl Pts',(-3.69471992586929,-2.19308453561,5.15939404919247));
#17688=CARTESIAN_POINT('Ctrl Pts',(-3.47754216233122,-2.20821978609556,
5.14828026013568));
#17689=CARTESIAN_POINT('Ctrl Pts',(-3.37245399619058,-2.39886344568463,
5.13716647107886));
#17690=CARTESIAN_POINT('Ctrl Pts',(-3.47563999441657,-2.59056248594111,
5.12605268202207));
#17691=CARTESIAN_POINT('Ctrl Pts',(-3.69265475207253,-2.60782999088153,
5.11493889296526));
#17692=CARTESIAN_POINT('Ctrl Pts',(-3.82486124676799,-2.434872109133,5.10382510390846));
#17693=CARTESIAN_POINT('Ctrl Pts',(-3.75124985081366,-2.22999351220008,
5.09271131485165));
#17694=CARTESIAN_POINT('Ctrl Pts',(-3.53919767190563,-2.18072471954551,
5.08159752579485));
#17695=CARTESIAN_POINT('Ctrl Pts',(-3.38279859300748,-2.33216060940528,
5.07048373673804));
#17696=CARTESIAN_POINT('Ctrl Pts',(-3.42520640540474,-2.54569089676662,
5.05936994768124));
#17697=CARTESIAN_POINT('Ctrl Pts',(-3.62760478709563,-2.62586853724007,
5.04825615862444));
#17698=CARTESIAN_POINT('Ctrl Pts',(-3.80473618917098,-2.49930620239979,
5.03714236956763));
#17699=CARTESIAN_POINT('Ctrl Pts',(-3.79447023789256,-2.28184774515603,
5.02602858051083));
#17700=CARTESIAN_POINT('Ctrl Pts',(-3.60620347119968,-2.17253540126032,
5.01491479145402));
#17701=CARTESIAN_POINT('Ctrl Pts',(-3.4122585975793,-2.27142397694788,5.00380100239722));
#17702=CARTESIAN_POINT('Ctrl Pts',(-3.39015555842041,-2.48799964831557,
4.99268721334041));
#17703=CARTESIAN_POINT('Ctrl Pts',(-3.56012551659021,-2.62402824178367,
4.98157342428361));
#17704=CARTESIAN_POINT('Ctrl Pts',(-3.76659304155595,-2.55500124579927,
4.97045963522681));
#17705=CARTESIAN_POINT('Ctrl Pts',(-3.82057606633011,-2.34409985124907,
4.95934584617));
#17706=CARTESIAN_POINT('Ctrl Pts',(-3.67266331607053,-2.18436449702716,
4.9482320571132));
#17707=CARTESIAN_POINT('Ctrl Pts',(-3.45824100856306,-2.22200276403647,
4.93711826805639));
#17708=CARTESIAN_POINT('Ctrl Pts',(-3.37357231356937,-2.42256391980546,
4.92600447899959));
#17709=CARTESIAN_POINT('Ctrl Pts',(-3.49615544783263,-2.60247206385614,
4.91489068994279));
#17710=CARTESIAN_POINT('Ctrl Pts',(-3.71378867837081,-2.59705523168396,
4.90377690088598));
#17711=CARTESIAN_POINT('Ctrl Pts',(-3.82726984114541,-2.41127151118611,
4.89266311182918));
#17712=CARTESIAN_POINT('Ctrl Pts',(-3.73272834090401,-2.21517084867549,
4.88154932277237));
#17713=CARTESIAN_POINT('Ctrl Pts',(-3.51669908499156,-2.18824640447558,
4.87043553371557));
#17714=CARTESIAN_POINT('Ctrl Pts',(-3.37691610128289,-2.35514242770916,
4.85932174465877));
#17715=CARTESIAN_POINT('Ctrl Pts',(-3.44132434001351,-2.56309709557957,
4.84820795560196));
#17716=CARTESIAN_POINT('Ctrl Pts',(-3.65097020983412,-2.62176714221935,
4.83709416654516));
#17717=CARTESIAN_POINT('Ctrl Pts',(-3.81396246855208,-2.47745120857521,
4.82598037748835));
#17718=CARTESIAN_POINT('Ctrl Pts',(-3.78111245330488,-2.26224330536578,
4.81486658843155));
#17719=CARTESIAN_POINT('Ctrl Pts',(-3.58248815559281,-2.1731256670222,4.80375279937474));
#17720=CARTESIAN_POINT('Ctrl Pts',(-3.39989264766446,-2.29166867858314,
4.79263901031794));
#17721=CARTESIAN_POINT('Ctrl Pts',(-3.40045766870055,-2.50936857719767,
4.78152522126113));
#17722=CARTESIAN_POINT('Ctrl Pts',(-3.58366604853898,-2.62696217677915,
4.77041143220433));
#17723=CARTESIAN_POINT('Ctrl Pts',(-3.78182507938928,-2.53681472202852,
4.75929764314753));
#17724=CARTESIAN_POINT('Ctrl Pts',(-3.81355755303793,-2.32143920062071,
4.74818385409072));
#17725=CARTESIAN_POINT('Ctrl Pts',(-3.64981837648358,-2.17797126982482,
4.73707006503392));
#17726=CARTESIAN_POINT('Ctrl Pts',(-3.440479874955,-2.23772875373533,4.72595627597712));
#17727=CARTESIAN_POINT('Ctrl Pts',(-3.37715195296136,-2.44601494963299,
4.71484248692031));
#17728=CARTESIAN_POINT('Ctrl Pts',(-3.51779937569094,-2.61218314028655,
4.7037286978635));
#17729=CARTESIAN_POINT('Ctrl Pts',(-3.73368596206909,-2.58413769631535,
4.69261490880671));
#17730=CARTESIAN_POINT('Ctrl Pts',(-3.82720827126346,-2.38754893064322,
4.68150111974989));
#17731=CARTESIAN_POINT('Ctrl Pts',(-3.71276427305336,-2.20235676995803,
4.6703873306931));
#17732=CARTESIAN_POINT('Ctrl Pts',(-3.49510585688365,-2.19806969915704,
4.65927354163628));
#17733=CARTESIAN_POINT('Ctrl Pts',(-3.37345823948888,-2.37861172276277,
4.64815975257949));
#17734=CARTESIAN_POINT('Ctrl Pts',(-3.45916686464814,-2.57873067908372,
4.63704596352267));
#17735=CARTESIAN_POINT('Ctrl Pts',(-3.67378165575153,-2.61525541789472,
4.62593217446588));
#17736=CARTESIAN_POINT('Ctrl Pts',(-3.82086326060429,-2.45475443154594,
4.61481838540906));
#17737=CARTESIAN_POINT('Ctrl Pts',(-3.76578621826694,-2.24413609304223,
4.60370459635227));
#17738=CARTESIAN_POINT('Ctrl Pts',(-3.55896317020481,-2.17618175620078,
4.59259080729546));
#17739=CARTESIAN_POINT('Ctrl Pts',(-3.38970159784644,-2.3130907961665,4.58147701823866));
#17740=CARTESIAN_POINT('Ctrl Pts',(-3.41292853791948,-2.52954881604603,
4.57036322918185));
#17741=CARTESIAN_POINT('Ctrl Pts',(-3.60738410878117,-2.62742933535986,
4.55924944012506));
#17742=CARTESIAN_POINT('Ctrl Pts',(-3.79508092111058,-2.51714120490541,
4.54813565106824));
#17743=CARTESIAN_POINT('Ctrl Pts',(-3.8042179540262,-2.29963240090777,4.53702186201145));
#17744=CARTESIAN_POINT('Ctrl Pts',(-3.62643197753871,-2.17399119904908,
4.52590807295463));
#17745=CARTESIAN_POINT('Ctrl Pts',(-3.42445251243888,-2.25521841492616,
4.51479428389784));
#17746=CARTESIAN_POINT('Ctrl Pts',(-3.38315365317149,-2.46896585933577,
4.50368049484102));
#17747=CARTESIAN_POINT('Ctrl Pts',(-3.54033671511431,-2.61958806700588,
4.49256670578423));
#17748=CARTESIAN_POINT('Ctrl Pts',(-3.75213025683239,-2.56921883378282,
4.48145291672742));
#17749=CARTESIAN_POINT('Ctrl Pts',(-3.82467725221749,-2.3639616686385,4.47033912767062));
#17750=CARTESIAN_POINT('Ctrl Pts',(-3.69157460458704,-2.1916908255014,4.45922533861381));
#17751=CARTESIAN_POINT('Ctrl Pts',(-3.47465269496093,-2.21008767488223,
4.44811154955701));
#17752=CARTESIAN_POINT('Ctrl Pts',(-3.37246257092429,-2.40231354390696,
4.4369977605002));
#17753=CARTESIAN_POINT('Ctrl Pts',(-3.47854008472427,-2.59242157025994,
4.4258839714434));
#17754=CARTESIAN_POINT('Ctrl Pts',(-3.69579113920209,-2.60640441108558,
4.41477018238659));
#17755=CARTESIAN_POINT('Ctrl Pts',(-3.82536367230107,-2.43146203268096,
4.4036563933298));
#17756=CARTESIAN_POINT('Ctrl Pts',(-3.74865789052413,-2.22772394311352,
4.39254260427298));
#17757=CARTESIAN_POINT('Ctrl Pts',(-3.53588463622708,-2.18166838945074,
4.38142881521619));
#17758=CARTESIAN_POINT('Ctrl Pts',(-3.38179533850196,-2.33546162919725,
4.37031502615938));
#17759=CARTESIAN_POINT('Ctrl Pts',(-3.42743437181836,-2.54831276553967,
4.35920123710258));
#17760=CARTESIAN_POINT('Ctrl Pts',(-3.63101841437027,-2.62544119350812,
4.34808744804577));
#17761=CARTESIAN_POINT('Ctrl Pts',(-3.80622350364941,-2.49616136905929,
4.33697365898897));
#17762=CARTESIAN_POINT('Ctrl Pts',(-3.7926446962851,-2.27898290099381,4.32585986993216));
#17763=CARTESIAN_POINT('Ctrl Pts',(-3.60278713071383,-2.17233370304593,
4.31474608087535));
#17764=CARTESIAN_POINT('Ctrl Pts',(-3.4102684797223,-2.27455956054189,4.30363229181856));
#17765=CARTESIAN_POINT('Ctrl Pts',(-3.3979620342723,-2.41847764084731,4.29622309911402));
#17766=CARTESIAN_POINT('Ctrl Pts',(-3.42361008748733,-2.47713148324918,
4.29251850276175));
#17767=CARTESIAN_POINT('Ctrl Pts',(-3.44347998857283,-2.26687801966678,
5.22244449171475));
#17768=CARTESIAN_POINT('Ctrl Pts',(-3.39921376300775,-2.31892464723302,
5.21873989536248));
#17769=CARTESIAN_POINT('Ctrl Pts',(-3.36748907565365,-2.46979092850336,
5.21133070265795));
#17770=CARTESIAN_POINT('Ctrl Pts',(-3.53276732806678,-2.63352307897406,
5.20021691360113));
#17771=CARTESIAN_POINT('Ctrl Pts',(-3.75962268259409,-2.58297478841644,
5.18910312454434));
#17772=CARTESIAN_POINT('Ctrl Pts',(-3.84035223880946,-2.36520763584968,
5.17798933548753));
#17773=CARTESIAN_POINT('Ctrl Pts',(-3.70109554203788,-2.17915701647198,
5.16687554643073));
#17774=CARTESIAN_POINT('Ctrl Pts',(-3.46929950206046,-2.19531102353728,
5.15576175737392));
#17775=CARTESIAN_POINT('Ctrl Pts',(-3.35713783153282,-2.39878694399818,
5.14464796831711));
#17776=CARTESIAN_POINT('Ctrl Pts',(-3.46726929886284,-2.60338928299931,
5.13353417926032));
#17777=CARTESIAN_POINT('Ctrl Pts',(-3.69889136100131,-2.62181906697108,
5.12242039020351));
#17778=CARTESIAN_POINT('Ctrl Pts',(-3.83999669992028,-2.43721935741029,
5.1113066011467));
#17779=CARTESIAN_POINT('Ctrl Pts',(-3.76143050694799,-2.21855034327406,
5.10019281208991));
#17780=CARTESIAN_POINT('Ctrl Pts',(-3.53510505567384,-2.16596525884485,
5.0890790230331));
#17781=CARTESIAN_POINT('Ctrl Pts',(-3.36817872512274,-2.32759432716241,
5.07796523397629));
#17782=CARTESIAN_POINT('Ctrl Pts',(-3.41344101541272,-2.5554973786501,5.06685144491949));
#17783=CARTESIAN_POINT('Ctrl Pts',(-3.62946287054873,-2.64107179130501,
5.05573765586269));
#17784=CARTESIAN_POINT('Ctrl Pts',(-3.81851702088083,-2.50599052171118,
5.04462386680588));
#17785=CARTESIAN_POINT('Ctrl Pts',(-3.8075600664755,-2.27389489448153,5.03351007774907));
#17786=CARTESIAN_POINT('Ctrl Pts',(-3.60662102802227,-2.15722471599323,
5.02239628869228));
#17787=CARTESIAN_POINT('Ctrl Pts',(-3.39962168818772,-2.262769500459,5.01128249963546));
#17788=CARTESIAN_POINT('Ctrl Pts',(-3.37603088927244,-2.49392292132789,
5.00016871057867));
#17789=CARTESIAN_POINT('Ctrl Pts',(-3.55744155755193,-2.63910762521254,
4.98905492152185));
#17790=CARTESIAN_POINT('Ctrl Pts',(-3.77780645076812,-2.56543440904132,
4.97794113246506));
#17791=CARTESIAN_POINT('Ctrl Pts',(-3.83542308317469,-2.34033720163832,
4.96682734340825));
#17792=CARTESIAN_POINT('Ctrl Pts',(-3.67755429765177,-2.16985003043886,
4.95571355435145));
#17793=CARTESIAN_POINT('Ctrl Pts',(-3.44869918397279,-2.21002173633656,
4.94459976529464));
#17794=CARTESIAN_POINT('Ctrl Pts',(-3.3583314230664,-2.42408270152555,4.93348597623784));
#17795=CARTESIAN_POINT('Ctrl Pts',(-3.48916565133794,-2.61610049686178,
4.92237218718103));
#17796=CARTESIAN_POINT('Ctrl Pts',(-3.7214478158856,-2.61031905668909,4.91125839812423));
#17797=CARTESIAN_POINT('Ctrl Pts',(-3.8425674172419,-2.41203019874106,4.90014460906743));
#17798=CARTESIAN_POINT('Ctrl Pts',(-3.74166231069475,-2.20272996345734,
4.88903082001062));
#17799=CARTESIAN_POINT('Ctrl Pts',(-3.511092084609,-2.17399322981363,4.87791703095382));
#17800=CARTESIAN_POINT('Ctrl Pts',(-3.36190028176488,-2.35212305601353,
4.86680324189701));
#17801=CARTESIAN_POINT('Ctrl Pts',(-3.43064385125587,-2.57407519200526,
4.85568945284021));
#17802=CARTESIAN_POINT('Ctrl Pts',(-3.6544010243217,-2.63669433060785,4.84457566378341));
#17803=CARTESIAN_POINT('Ctrl Pts',(-3.82836432287631,-2.48266446410869,
4.8334618747266));
#17804=CARTESIAN_POINT('Ctrl Pts',(-3.79330316687467,-2.25297087613211,
4.8223480856698));
#17805=CARTESIAN_POINT('Ctrl Pts',(-3.58130943002562,-2.15785471265546,
4.81123429661298));
#17806=CARTESIAN_POINT('Ctrl Pts',(-3.38642338383962,-2.28437687679961,
4.8001205075562));
#17807=CARTESIAN_POINT('Ctrl Pts',(-3.38702643654876,-2.51673019686447,
4.78900671849938));
#17808=CARTESIAN_POINT('Ctrl Pts',(-3.58256660716932,-2.64223904392882,
4.77789292944258));
#17809=CARTESIAN_POINT('Ctrl Pts',(-3.79406375995591,-2.54602374690751,
4.76677914038577));
#17810=CARTESIAN_POINT('Ctrl Pts',(-3.82793215242214,-2.31615125831984,
4.75566535132897));
#17811=CARTESIAN_POINT('Ctrl Pts',(-3.65317166084996,-2.16302647390142,
4.74455156227217));
#17812=CARTESIAN_POINT('Ctrl Pts',(-3.42974254509416,-2.22680624538361,
4.73343777321536));
#17813=CARTESIAN_POINT('Ctrl Pts',(-3.36215200866455,-2.44911222461694,
4.72232398415856));
#17814=CARTESIAN_POINT('Ctrl Pts',(-3.51226643608395,-2.62646522768789,
4.71121019510176));
#17815=CARTESIAN_POINT('Ctrl Pts',(-3.74268438952201,-2.59653203956573,
4.70009640604495));
#17816=CARTESIAN_POINT('Ctrl Pts',(-3.84250170307953,-2.38671084680417,
4.68898261698815));
#17817=CARTESIAN_POINT('Ctrl Pts',(-3.72035445765201,-2.18905336667194,
4.67786882793134));
#17818=CARTESIAN_POINT('Ctrl Pts',(-3.4880454122232,-2.18447773232253,4.66675503887454));
#17819=CARTESIAN_POINT('Ctrl Pts',(-3.35820967063793,-2.37717207376684,
4.65564124981773));
#17820=CARTESIAN_POINT('Ctrl Pts',(-3.4496873596065,-2.5907610749791,4.64452746076093));
#17821=CARTESIAN_POINT('Ctrl Pts',(-3.67874791298872,-2.62974430088435,
4.63341367170412));
#17822=CARTESIAN_POINT('Ctrl Pts',(-3.83572960854991,-2.4584399627144,4.62229988264733));
#17823=CARTESIAN_POINT('Ctrl Pts',(-3.77694532005055,-2.23364486391404,
4.61118609359051));
#17824=CARTESIAN_POINT('Ctrl Pts',(-3.55620097341096,-2.16111650777606,
4.60007230453371));
#17825=CARTESIAN_POINT('Ctrl Pts',(-3.37554637252617,-2.307240921179,4.58895851547691));
#17826=CARTESIAN_POINT('Ctrl Pts',(-3.40033672233922,-2.53826877141577,
4.57784472642011));
#17827=CARTESIAN_POINT('Ctrl Pts',(-3.60788113454322,-2.64273764704216,
4.5667309373633));
#17828=CARTESIAN_POINT('Ctrl Pts',(-3.8082118548967,-2.52502600161686,4.5556171483065));
#17829=CARTESIAN_POINT('Ctrl Pts',(-3.8179639032302,-2.29287663878378,4.54450335924969));
#17830=CARTESIAN_POINT('Ctrl Pts',(-3.62821111895818,-2.15877850380716,
4.53338957019289));
#17831=CARTESIAN_POINT('Ctrl Pts',(-3.4126363777684,-2.24547313898512,4.52227578113608));
#17832=CARTESIAN_POINT('Ctrl Pts',(-3.3685576844537,-2.47360796440317,4.51116199207928));
#17833=CARTESIAN_POINT('Ctrl Pts',(-3.53632076809686,-2.63436858142862,
4.50004820302248));
#17834=CARTESIAN_POINT('Ctrl Pts',(-3.76237017326276,-2.5806089855676,4.48893441396567));
#17835=CARTESIAN_POINT('Ctrl Pts',(-3.83980032066171,-2.36153592172191,
4.47782062490887));
#17836=CARTESIAN_POINT('Ctrl Pts',(-3.69773850858379,-2.17766949547173,
4.46670683585206));
#17837=CARTESIAN_POINT('Ctrl Pts',(-3.46621554409366,-2.19730464027232,
4.45559304679525));
#17838=CARTESIAN_POINT('Ctrl Pts',(-3.35714698343348,-2.40246926898597,
4.44447925773846));
#17839=CARTESIAN_POINT('Ctrl Pts',(-3.47036459479899,-2.60537350263611,
4.43336546868164));
#17840=CARTESIAN_POINT('Ctrl Pts',(-3.70223885894321,-2.62029753112878,
4.42225167962485));
#17841=CARTESIAN_POINT('Ctrl Pts',(-3.84053294381125,-2.43357974806573,
4.41113789056804));
#17842=CARTESIAN_POINT('Ctrl Pts',(-3.75866408131995,-2.21612800906199,
4.40002410151124));
#17843=CARTESIAN_POINT('Ctrl Pts',(-3.53156901893564,-2.16697244735031,
4.38891031245443));
#17844=CARTESIAN_POINT('Ctrl Pts',(-3.36710794136624,-2.33111753922242,
4.37779652339762));
#17845=CARTESIAN_POINT('Ctrl Pts',(-3.41581894666805,-2.55829572590735,
4.36668273434083));
#17846=CARTESIAN_POINT('Ctrl Pts',(-3.63310626972243,-2.64061568298545,
4.35556894528402));
#17847=CARTESIAN_POINT('Ctrl Pts',(-3.82010444677879,-2.50263400904229,
4.34445515622722));
#17848=CARTESIAN_POINT('Ctrl Pts',(-3.80561164731632,-2.27083721711559,
4.33334136717041));
#17849=CARTESIAN_POINT('Ctrl Pts',(-3.60297473301061,-2.15700944143379,
4.32222757811361));
#17850=CARTESIAN_POINT('Ctrl Pts',(-3.39749761512046,-2.26611614077921,
4.3111137890568));
#17851=CARTESIAN_POINT('Ctrl Pts',(-3.38436282049399,-2.419721374356,4.30370459635227));
#17852=CARTESIAN_POINT('Ctrl Pts',(-3.41173724903364,-2.48232321801035,
4.3));
#17853=CARTESIAN_POINT('Ctrl Pts',(-3.47309291201476,-2.29206413469515,
5.2));
#17854=CARTESIAN_POINT('Ctrl Pts',(-3.46488110023315,-2.2997248835417,5.2));
#17855=CARTESIAN_POINT('Ctrl Pts',(-3.45756393061001,-2.3082260406838,5.2));
#17856=CARTESIAN_POINT('Ctrl Pts',(-3.45114583189458,-2.31737340047652,
5.2));
#17857=CARTESIAN_POINT('Ctrl Pts',(-3.44637506584917,-2.32417290846779,
5.2));
#17858=CARTESIAN_POINT('Ctrl Pts',(-3.44210141208336,-2.33133076253531,
5.2));
#17859=CARTESIAN_POINT('Ctrl Pts',(-3.43833687158849,-2.33878162457801,
5.2));
#17860=CARTESIAN_POINT('Ctrl Pts',(-3.43611957198332,-2.34317015313494,
5.2));
#17861=CARTESIAN_POINT('Ctrl Pts',(-3.43407750155671,-2.34766554493455,
5.2));
#17862=CARTESIAN_POINT('Ctrl Pts',(-3.43222557143088,-2.35222601439271,
5.2));
#17863=CARTESIAN_POINT('Ctrl Pts',(-3.42766723914997,-2.36345113290954,
5.2));
#17864=CARTESIAN_POINT('Ctrl Pts',(-3.42424191788099,-2.37509439510727,
5.2));
#17865=CARTESIAN_POINT('Ctrl Pts',(-3.42197769676804,-2.38695730471617,
5.2));
#17866=CARTESIAN_POINT('Ctrl Pts',(-3.42053881602809,-2.39449601728207,
5.2));
#17867=CARTESIAN_POINT('Ctrl Pts',(-3.41956956713255,-2.40212431376417,
5.2));
#17868=CARTESIAN_POINT('Ctrl Pts',(-3.41908672349853,-2.40979637190619,
5.2));
#17869=CARTESIAN_POINT('Ctrl Pts',(-3.4188613967758,-2.41337666083611,5.2));
#17870=CARTESIAN_POINT('Ctrl Pts',(-3.41874254028701,-2.41696303084227,
5.2));
#17871=CARTESIAN_POINT('Ctrl Pts',(-3.4187313001846,-2.42054068183377,5.2));
#17872=CARTESIAN_POINT('Ctrl Pts',(-3.41869625236243,-2.43169617411961,
5.2));
#17873=CARTESIAN_POINT('Ctrl Pts',(-3.41970314531555,-2.44279404991157,
5.2));
#17874=CARTESIAN_POINT('Ctrl Pts',(-3.4217856982914,-2.45369315923086,5.2));
#17875=CARTESIAN_POINT('Ctrl Pts',(-3.42294608022389,-2.45976605614203,
5.2));
#17876=CARTESIAN_POINT('Ctrl Pts',(-3.42444095669484,-2.46577748192705,
5.2));
#17877=CARTESIAN_POINT('Ctrl Pts',(-3.42625159798616,-2.47171129566944,
5.2));
#17878=CARTESIAN_POINT('Ctrl Pts',(-3.42738424188737,-2.4754231838156,5.2));
#17879=CARTESIAN_POINT('Ctrl Pts',(-3.4286411006463,-2.47910621955531,5.2));
#17880=CARTESIAN_POINT('Ctrl Pts',(-3.43001647345192,-2.48275158788973,
5.2));
#17881=CARTESIAN_POINT('Ctrl Pts',(-3.43439826051469,-2.49436533198986,
5.2));
#17882=CARTESIAN_POINT('Ctrl Pts',(-3.43994736167241,-2.50551615790537,
5.2));
#17883=CARTESIAN_POINT('Ctrl Pts',(-3.44649835855225,-2.51608152365555,
5.2));
#17884=CARTESIAN_POINT('Ctrl Pts',(-3.45083933347942,-2.52308259366964,
5.2));
#17885=CARTESIAN_POINT('Ctrl Pts',(-3.45562142913928,-2.5298267361278,5.2));
#17886=CARTESIAN_POINT('Ctrl Pts',(-3.46080806253422,-2.53627607801171,
5.2));
#17887=CARTESIAN_POINT('Ctrl Pts',(-3.46351819008795,-2.53964599792162,
5.2));
#17888=CARTESIAN_POINT('Ctrl Pts',(-3.46634016652161,-2.54293674743321,
5.2));
#17889=CARTESIAN_POINT('Ctrl Pts',(-3.46926561316249,-2.5461381198978,5.2));
#17890=CARTESIAN_POINT('Ctrl Pts',(-3.47553204021621,-2.55299559141714,
5.2));
#17891=CARTESIAN_POINT('Ctrl Pts',(-3.48224800724127,-2.55941730873493,
5.2));
#17892=CARTESIAN_POINT('Ctrl Pts',(-3.48935943070669,-2.56535251864156,
5.2));
#17893=CARTESIAN_POINT('Ctrl Pts',(-3.49388595591638,-2.56913036669094,
5.2));
#17894=CARTESIAN_POINT('Ctrl Pts',(-3.49857295100653,-2.57271103243443,
5.2));
#17895=CARTESIAN_POINT('Ctrl Pts',(-3.50340866428261,-2.5760800097667,5.2));
#17896=CARTESIAN_POINT('Ctrl Pts',(-3.50748115648314,-2.57891726109367,
5.2));
#17897=CARTESIAN_POINT('Ctrl Pts',(-3.51165212725609,-2.58159933242901,
5.2));
#17898=CARTESIAN_POINT('Ctrl Pts',(-3.51591076075252,-2.58411660325874,
5.2));
#17899=CARTESIAN_POINT('Ctrl Pts',(-3.52463384142318,-2.58927280102407,
5.2));
#17900=CARTESIAN_POINT('Ctrl Pts',(-3.53372795938425,-2.593741186929,5.2));
#17901=CARTESIAN_POINT('Ctrl Pts',(-3.54313434616876,-2.59744798259885,
5.2));
#17902=CARTESIAN_POINT('Ctrl Pts',(-3.54437365456163,-2.59793635960157,
5.2));
#17903=CARTESIAN_POINT('Ctrl Pts',(-3.54561839868079,-2.59841149645932,
5.2));
#17904=CARTESIAN_POINT('Ctrl Pts',(-3.54686838721289,-2.59887345127292,
5.2));
#17905=CARTESIAN_POINT('Ctrl Pts',(-3.76673281282141,-2.40013003219325,
5.08714803633902));
#17906=CARTESIAN_POINT('Ctrl Pts',(-3.76680596527292,-2.4086546123928,5.08771939403667));
#17907=CARTESIAN_POINT('Ctrl Pts',(-3.76620865763489,-2.417168907206,5.08829075173431));
#17908=CARTESIAN_POINT('Ctrl Pts',(-3.76490523910227,-2.42557368984471,
5.08886210943196));
#17909=CARTESIAN_POINT('Ctrl Pts',(-3.75645407171393,-2.48006902128643,
5.09256670578423));
#17910=CARTESIAN_POINT('Ctrl Pts',(-3.71831780296444,-2.52996042999443,
5.09627130213649));
#17911=CARTESIAN_POINT('Ctrl Pts',(-3.66794964380788,-2.55241564320215,
5.09997589848876));
#17912=CARTESIAN_POINT('Ctrl Pts',(-3.61758148465131,-2.57487085640986,
5.10368049484103));
#17913=CARTESIAN_POINT('Ctrl Pts',(-3.55498143508767,-2.56988987411729,
5.1073850911933));
#17914=CARTESIAN_POINT('Ctrl Pts',(-3.50879890030286,-2.53975064250981,
5.11108968754557));
#17915=CARTESIAN_POINT('Ctrl Pts',(-3.46261636551805,-2.50961141090233,
5.11479428389784));
#17916=CARTESIAN_POINT('Ctrl Pts',(-3.43285134551208,-2.45431392997993,
5.1184988802501));
#17917=CARTESIAN_POINT('Ctrl Pts',(-3.4331256950702,-2.3991686665445,5.12220347660237));
#17918=CARTESIAN_POINT('Ctrl Pts',(-3.43340004462832,-2.34402340310906,
5.12590807295464));
#17919=CARTESIAN_POINT('Ctrl Pts',(-3.46371376375052,-2.28903035716059,
5.12961266930691));
#17920=CARTESIAN_POINT('Ctrl Pts',(-3.51019415842152,-2.25935087796534,
5.13331726565918));
#17921=CARTESIAN_POINT('Ctrl Pts',(-3.55667455309252,-2.22967139877009,
5.13702186201145));
#17922=CARTESIAN_POINT('Ctrl Pts',(-3.61932162331232,-2.22530548632806,
5.14072645836371));
#17923=CARTESIAN_POINT('Ctrl Pts',(-3.66946347831689,-2.24826430176485,
5.14443105471598));
#17924=CARTESIAN_POINT('Ctrl Pts',(-3.71960533332146,-2.27122311720164,
5.14813565106825));
#17925=CARTESIAN_POINT('Ctrl Pts',(-3.7572419731108,-2.32150666051725,5.15184024742051));
#17926=CARTESIAN_POINT('Ctrl Pts',(-3.76515098200617,-2.37607618706626,
5.15554484377278));
#17927=CARTESIAN_POINT('Ctrl Pts',(-3.76629187681735,-2.3839479811825,5.15607924129486));
#17928=CARTESIAN_POINT('Ctrl Pts',(-3.7668141752375,-2.39190896147606,5.15661363881694));
#17929=CARTESIAN_POINT('Ctrl Pts',(-3.76674783764939,-2.3998784327954,5.15714803633902));
#17930=CARTESIAN_POINT('Ctrl Pts',(-3.65301702171886,-2.59851743256717,
5.2));
#17931=CARTESIAN_POINT('Ctrl Pts',(-3.71902879097456,-2.58088801151799,
5.19629540364773));
#17932=CARTESIAN_POINT('Ctrl Pts',(-3.83093278328674,-2.47484748886485,
5.1888862109432));
#17933=CARTESIAN_POINT('Ctrl Pts',(-3.78812295700318,-2.24617213689742,
5.17777242188639));
#17934=CARTESIAN_POINT('Ctrl Pts',(-3.5727867642971,-2.15871465280967,5.16665863282959));
#17935=CARTESIAN_POINT('Ctrl Pts',(-3.38252461999799,-2.29190667528476,
5.15554484377278));
#17936=CARTESIAN_POINT('Ctrl Pts',(-3.39123766053156,-2.52413789941101,
5.14443105471598));
#17937=CARTESIAN_POINT('Ctrl Pts',(-3.59107442597796,-2.64269432067786,
5.13331726565918));
#17938=CARTESIAN_POINT('Ctrl Pts',(-3.79906030223171,-2.53913483234337,
5.12220347660237));
#17939=CARTESIAN_POINT('Ctrl Pts',(-3.82485429799751,-2.30821119218956,
5.11108968754557));
#17940=CARTESIAN_POINT('Ctrl Pts',(-3.64483147519039,-2.16130911215383,
5.09997589848876));
#17941=CARTESIAN_POINT('Ctrl Pts',(-3.42377645640768,-2.23288040078699,
5.08886210943196));
#17942=CARTESIAN_POINT('Ctrl Pts',(-3.36401956629289,-2.45741970591997,
5.07774832037515));
#17943=CARTESIAN_POINT('Ctrl Pts',(-3.52025888222192,-2.62940132794335,
5.06663453131835));
#17944=CARTESIAN_POINT('Ctrl Pts',(-3.74948582853024,-2.5914096999913,5.05552074226155));
#17945=CARTESIAN_POINT('Ctrl Pts',(-3.84188686003135,-2.37821840959849,
5.04440695320474));
#17946=CARTESIAN_POINT('Ctrl Pts',(-3.71288602579316,-2.18496415245566,
5.03329316414794));
#17947=CARTESIAN_POINT('Ctrl Pts',(-3.4805593716682,-2.1885345970333,5.02217937509112));
#17948=CARTESIAN_POINT('Ctrl Pts',(-3.35755805936012,-2.38566174720256,
5.01106558603434));
#17949=CARTESIAN_POINT('Ctrl Pts',(-3.45646661470834,-2.59591285074103,
4.99995179697752));
#17950=CARTESIAN_POINT('Ctrl Pts',(-3.68675290044432,-2.62684270619768,
4.98883800792072));
#17951=CARTESIAN_POINT('Ctrl Pts',(-3.83763327503031,-2.45014085710183,
4.97772421886392));
#17952=CARTESIAN_POINT('Ctrl Pts',(-3.77100521680217,-2.22754451436212,
4.96661042980711));
#17953=CARTESIAN_POINT('Ctrl Pts',(-3.54785414492032,-2.16279863265717,
4.9554966407503));
#17954=CARTESIAN_POINT('Ctrl Pts',(-3.37243276525931,-2.31516585290104,
4.94438285169351));
#17955=CARTESIAN_POINT('Ctrl Pts',(-3.40530625649813,-2.54518272988275,
4.9332690626367));
#17956=CARTESIAN_POINT('Ctrl Pts',(-3.61638513906469,-2.64231220781178,
4.9221552735799));
#17957=CARTESIAN_POINT('Ctrl Pts',(-3.81246651806354,-2.51765057387683,
4.91104148452309));
#17958=CARTESIAN_POINT('Ctrl Pts',(-3.81407488352551,-2.2853020354474,4.89992769546629));
#17959=CARTESIAN_POINT('Ctrl Pts',(-3.61973808033182,-2.15793784472475,
4.88881390640949));
#17960=CARTESIAN_POINT('Ctrl Pts',(-3.4073347883606,-2.25213588990288,4.87770011735268));
#17961=CARTESIAN_POINT('Ctrl Pts',(-3.37128014957741,-2.48167563194308,
4.86658632829587));
#17962=CARTESIAN_POINT('Ctrl Pts',(-3.54457538374435,-2.63645674180255,
4.85547253923907));
#17963=CARTESIAN_POINT('Ctrl Pts',(-3.76860139772859,-2.57480631428759,
4.84435875018227));
#17964=CARTESIAN_POINT('Ctrl Pts',(-3.83830464030165,-2.35315368486712,
4.83324496112546));
#17965=CARTESIAN_POINT('Ctrl Pts',(-3.68988494304833,-2.17438001896094,
4.82213117206866));
#17966=CARTESIAN_POINT('Ctrl Pts',(-3.45919253805822,-2.20211888040452,
4.81101738301185));
#17967=CARTESIAN_POINT('Ctrl Pts',(-3.35738279984868,-2.41098057473832,
4.79990359395505));
#17968=CARTESIAN_POINT('Ctrl Pts',(-3.47764333640382,-2.60979162448597,
4.78878980489824));
#17969=CARTESIAN_POINT('Ctrl Pts',(-3.7098983147675,-2.61657802114276,4.77767601584144));
#17970=CARTESIAN_POINT('Ctrl Pts',(-3.84156211929281,-2.42512809888577,
4.76656222678463));
#17971=CARTESIAN_POINT('Ctrl Pts',(-3.75212137652867,-2.21067814274661,
4.75544843772783));
#17972=CARTESIAN_POINT('Ctrl Pts',(-3.52344221265408,-2.16951662960737,
4.74433464867103));
#17973=CARTESIAN_POINT('Ctrl Pts',(-3.36483725976158,-2.33931915924769,
4.73322085961422));
#17974=CARTESIAN_POINT('Ctrl Pts',(-3.42147942993616,-2.56466355059616,
4.72210707055742));
#17975=CARTESIAN_POINT('Ctrl Pts',(-3.64152350245114,-2.63928952667227,
4.71099328150061));
#17976=CARTESIAN_POINT('Ctrl Pts',(-3.82356064226404,-2.49489108525746,
4.69987949244381));
#17977=CARTESIAN_POINT('Ctrl Pts',(-3.80097019086255,-2.26363775736839,
4.688765703387));
#17978=CARTESIAN_POINT('Ctrl Pts',(-3.59442944460758,-2.15719833661306,
4.6776519143302));
#17979=CARTESIAN_POINT('Ctrl Pts',(-3.3929874908777,-2.27299803191391,4.6665381252734));
#17980=CARTESIAN_POINT('Ctrl Pts',(-3.38102643442896,-2.50504406890429,
4.65542433621659));
#17981=CARTESIAN_POINT('Ctrl Pts',(-3.5694943658766,-2.64094207834572,4.64431054715979));
#17982=CARTESIAN_POINT('Ctrl Pts',(-3.78588445019465,-2.55630307100846,
4.63319675810299));
#17983=CARTESIAN_POINT('Ctrl Pts',(-3.83213238917682,-2.32859809017945,
4.62208296904618));
#17984=CARTESIAN_POINT('Ctrl Pts',(-3.66590691978443,-2.16624808716256,
4.61096917998938));
#17985=CARTESIAN_POINT('Ctrl Pts',(-3.4393560992794,-2.21785386089149,4.59985539093257));
#17986=CARTESIAN_POINT('Ctrl Pts',(-3.35984446292695,-2.43618006142673,
4.58874160187577));
#17987=CARTESIAN_POINT('Ctrl Pts',(-3.50014991321196,-2.62139024142312,
4.57762781281897));
#17988=CARTESIAN_POINT('Ctrl Pts',(-3.73184928030013,-2.60395942271916,
4.56651402376216));
#17989=CARTESIAN_POINT('Ctrl Pts',(-3.84286550587893,-2.3998422313225,4.55540023470536));
#17990=CARTESIAN_POINT('Ctrl Pts',(-3.73158417960078,-2.19586944742698,
4.54428644564855));
#17991=CARTESIAN_POINT('Ctrl Pts',(-3.49986236155564,-2.17873967321655,
4.53317265659175));
#17992=CARTESIAN_POINT('Ctrl Pts',(-3.35979765944108,-2.36413198553984,
4.52205886753494));
#17993=CARTESIAN_POINT('Ctrl Pts',(-3.43959288407154,-2.58235469793693,
4.51094507847814));
#17994=CARTESIAN_POINT('Ctrl Pts',(-3.66621056034765,-2.6336660879353,4.49983128942134));
#17995=CARTESIAN_POINT('Ctrl Pts',(-3.83222496126862,-2.47110025635944,
4.48871750036453));
#17996=CARTESIAN_POINT('Ctrl Pts',(-3.78568121870704,-2.24345555647604,
4.47760371130773));
#17997=CARTESIAN_POINT('Ctrl Pts',(-3.56918135654791,-2.15909775573836,
4.46648992225092));
#17998=CARTESIAN_POINT('Ctrl Pts',(-3.38089013692747,-2.29524052189659,
4.45537613319412));
#17999=CARTESIAN_POINT('Ctrl Pts',(-3.39315268252002,-2.52727080497827,
4.44426234413731));
#18000=CARTESIAN_POINT('Ctrl Pts',(-3.59474487821944,-2.64280871984201,
4.43314855508051));
#18001=CARTESIAN_POINT('Ctrl Pts',(-3.80114723737323,-2.53610097383652,
4.42203476602371));
#18002=CARTESIAN_POINT('Ctrl Pts',(-3.82343706699101,-2.30481863511631,
4.4109209769669));
#18003=CARTESIAN_POINT('Ctrl Pts',(-3.64121277969171,-2.16065653443092,
4.3998071879101));
#18004=CARTESIAN_POINT('Ctrl Pts',(-3.42126523797479,-2.23556891230323,
4.38869339885329));
#18005=CARTESIAN_POINT('Ctrl Pts',(-3.36491711226222,-2.46098554747977,
4.37757960979649));
#18006=CARTESIAN_POINT('Ctrl Pts',(-3.52374009350676,-2.63058418685777,
4.36646582073969));
#18007=CARTESIAN_POINT('Ctrl Pts',(-3.7523704915333,-2.58912096342209,4.35535203168288));
#18008=CARTESIAN_POINT('Ctrl Pts',(-3.84152271736619,-2.3745642740037,4.34423824262608));
#18009=CARTESIAN_POINT('Ctrl Pts',(-3.70962995644976,-2.18326697275372,
4.33312445356927));
#18010=CARTESIAN_POINT('Ctrl Pts',(-3.47734459894833,-2.19039236572141,
4.32201066451247));
#18011=CARTESIAN_POINT('Ctrl Pts',(-3.35742142491826,-2.38928487622609,
4.31089687545566));
#18012=CARTESIAN_POINT('Ctrl Pts',(-3.45934320255763,-2.59816388104693,
4.29978308639886));
#18013=CARTESIAN_POINT('Ctrl Pts',(-3.69040341475663,-2.62529829024268,
4.28866929734205));
#18014=CARTESIAN_POINT('Ctrl Pts',(-3.7885754343637,-2.50643134569448,4.28126010463752));
#18015=CARTESIAN_POINT('Ctrl Pts',(-3.80166758614466,-2.43937207542898,
4.27755550828525));
#18016=CARTESIAN_POINT('Ctrl Pts',(-3.64967348970877,-2.58599788000028,
5.20748149723825));
#18017=CARTESIAN_POINT('Ctrl Pts',(-3.71152220988337,-2.5694802628904,5.20377690088598));
#18018=CARTESIAN_POINT('Ctrl Pts',(-3.81636894835099,-2.47012721287082,
5.19636770818145));
#18019=CARTESIAN_POINT('Ctrl Pts',(-3.77625893469146,-2.25587333035667,
5.18525391912464));
#18020=CARTESIAN_POINT('Ctrl Pts',(-3.57450297395432,-2.17393137483105,
5.17414013006784));
#18021=CARTESIAN_POINT('Ctrl Pts',(-3.39623976035988,-2.29872360840445,
5.16302634101103));
#18022=CARTESIAN_POINT('Ctrl Pts',(-3.40440331076774,-2.5163091110919,5.15191255195424));
#18023=CARTESIAN_POINT('Ctrl Pts',(-3.59163731958239,-2.62738874138378,
5.14079876289742));
#18024=CARTESIAN_POINT('Ctrl Pts',(-3.78650651345082,-2.53036025862013,
5.12968497384062));
#18025=CARTESIAN_POINT('Ctrl Pts',(-3.81067380428838,-2.31399987678807,
5.11857118478382));
#18026=CARTESIAN_POINT('Ctrl Pts',(-3.64200416676191,-2.17636221393428,
5.10745739572701));
#18027=CARTESIAN_POINT('Ctrl Pts',(-3.43489003917469,-2.24341984097745,
5.09634360667021));
#18028=CARTESIAN_POINT('Ctrl Pts',(-3.37890173259108,-2.45379851750672,
5.08522981761341));
#18029=CARTESIAN_POINT('Ctrl Pts',(-3.52528777617272,-2.61493407462981,
5.07411602855659));
#18030=CARTESIAN_POINT('Ctrl Pts',(-3.74005846658983,-2.57933839839392,
5.0630022394998));
#18031=CARTESIAN_POINT('Ctrl Pts',(-3.82663220344909,-2.37959207115806,
5.05188845044299));
#18032=CARTESIAN_POINT('Ctrl Pts',(-3.7057668397564,-2.19852544308029,5.04077466138619));
#18033=CARTESIAN_POINT('Ctrl Pts',(-3.48809192538747,-2.20187071665909,
5.02966087232937));
#18034=CARTESIAN_POINT('Ctrl Pts',(-3.37284772224266,-2.38656599277582,
5.01854708327259));
#18035=CARTESIAN_POINT('Ctrl Pts',(-3.46551858429622,-2.58355755679196,
5.00743329421577));
#18036=CARTESIAN_POINT('Ctrl Pts',(-3.68128180662955,-2.61253681301776,
4.99631950515897));
#18037=CARTESIAN_POINT('Ctrl Pts',(-3.82264687187209,-2.44697871114761,
4.98520571610216));
#18038=CARTESIAN_POINT('Ctrl Pts',(-3.76022072914644,-2.23842046359223,
4.97409192704536));
#18039=CARTESIAN_POINT('Ctrl Pts',(-3.5511427365839,-2.17775779744681,4.96297813798855));
#18040=CARTESIAN_POINT('Ctrl Pts',(-3.38678435101677,-2.32051594004622,
4.95186434893176));
#18041=CARTESIAN_POINT('Ctrl Pts',(-3.41758466713793,-2.53602674395714,
4.94075055987494));
#18042=CARTESIAN_POINT('Ctrl Pts',(-3.6153518060864,-2.62703072656315,4.92963677081815));
#18043=CARTESIAN_POINT('Ctrl Pts',(-3.79906726285858,-2.51023091039877,
4.91852298176134));
#18044=CARTESIAN_POINT('Ctrl Pts',(-3.80057419634206,-2.29253549186461,
4.90740919270453));
#18045=CARTESIAN_POINT('Ctrl Pts',(-3.61849329325651,-2.17320355634632,
4.89629540364773));
#18046=CARTESIAN_POINT('Ctrl Pts',(-3.41948526912059,-2.26146097775627,
4.88518161459093));
#18047=CARTESIAN_POINT('Ctrl Pts',(-3.38570442533712,-2.47652473736257,
4.87406782553412));
#18048=CARTESIAN_POINT('Ctrl Pts',(-3.54807075131856,-2.62154453701271,
4.86295403647732));
#18049=CARTESIAN_POINT('Ctrl Pts',(-3.75796850753643,-2.56378210944851,
4.85184024742052));
#18050=CARTESIAN_POINT('Ctrl Pts',(-3.82327589732119,-2.35610805969097,
4.84072645836371));
#18051=CARTESIAN_POINT('Ctrl Pts',(-3.68421632616712,-2.18860880066658,
4.8296126693069));
#18052=CARTESIAN_POINT('Ctrl Pts',(-3.46807259659411,-2.2145983037314,4.81849888025011));
#18053=CARTESIAN_POINT('Ctrl Pts',(-3.37268351551706,-2.41028808198908,
4.80738509119329));
#18054=CARTESIAN_POINT('Ctrl Pts',(-3.48535979063151,-2.59656106212739,
4.79627130213649));
#18055=CARTESIAN_POINT('Ctrl Pts',(-3.70296754948933,-2.60291947294643,
4.78515751307969));
#18056=CARTESIAN_POINT('Ctrl Pts',(-3.82632794256814,-2.42354338891427,
4.77404372402288));
#18057=CARTESIAN_POINT('Ctrl Pts',(-3.74252780308088,-2.22261777400868,
4.76292993496608));
#18058=CARTESIAN_POINT('Ctrl Pts',(-3.52827034905847,-2.18405212220422,
4.75181614590928));
#18059=CARTESIAN_POINT('Ctrl Pts',(-3.37966785801241,-2.34314601196173,
4.74070235685247));
#18060=CARTESIAN_POINT('Ctrl Pts',(-3.43273787526403,-2.55427900173875,
4.72958856779567));
#18061=CARTESIAN_POINT('Ctrl Pts',(-3.63890481216799,-2.62419867158141,
4.71847477873886));
#18062=CARTESIAN_POINT('Ctrl Pts',(-3.80946173328402,-2.48890675473974,
4.70736098968206));
#18063=CARTESIAN_POINT('Ctrl Pts',(-3.78829595446756,-2.27223747701361,
4.69624720062526));
#18064=CARTESIAN_POINT('Ctrl Pts',(-3.59478075310558,-2.17251068550248,
4.68513341156845));
#18065=CARTESIAN_POINT('Ctrl Pts',(-3.40604278761636,-2.28100744345521,
4.67401962251164));
#18066=CARTESIAN_POINT('Ctrl Pts',(-3.39483605824625,-2.4984194378808,4.66290583345485));
#18067=CARTESIAN_POINT('Ctrl Pts',(-3.57141821148077,-2.62574700466167,
4.65179204439804));
#18068=CARTESIAN_POINT('Ctrl Pts',(-3.77416159988632,-2.54644577793071,
4.64067825534124));
#18069=CARTESIAN_POINT('Ctrl Pts',(-3.81749290078935,-2.33310106985138,
4.62956446628443));
#18070=CARTESIAN_POINT('Ctrl Pts',(-3.66175048306201,-2.18098971122316,
4.61845067722763));
#18071=CARTESIAN_POINT('Ctrl Pts',(-3.44948714789117,-2.22934095365678,
4.60733688817083));
#18072=CARTESIAN_POINT('Ctrl Pts',(-3.37498993318483,-2.43389835661598,
4.59622309911401));
#18073=CARTESIAN_POINT('Ctrl Pts',(-3.50644698442724,-2.60742820932623,
4.58510931005722));
#18074=CARTESIAN_POINT('Ctrl Pts',(-3.72353417177652,-2.59109666965397,
4.57399552100041));
#18075=CARTESIAN_POINT('Ctrl Pts',(-3.82754913074644,-2.39985218104442,
4.56288173194361));
#18076=CARTESIAN_POINT('Ctrl Pts',(-3.72328578972046,-2.20874299284009,
4.5517679428868));
#18077=CARTESIAN_POINT('Ctrl Pts',(-3.50617756728955,-2.19269351221351,
4.54065415383));
#18078=CARTESIAN_POINT('Ctrl Pts',(-3.37494608137275,-2.36639401102897,
4.52954036477319));
#18079=CARTESIAN_POINT('Ctrl Pts',(-3.44970899978995,-2.57085445235588,
4.51842657571639));
#18080=CARTESIAN_POINT('Ctrl Pts',(-3.66203497445559,-2.61892987644406,
4.50731278665958));
#18081=CARTESIAN_POINT('Ctrl Pts',(-3.81757963479854,-2.46661630054004,
4.49619899760278));
#18082=CARTESIAN_POINT('Ctrl Pts',(-3.77397118524436,-2.2533280717731,4.48508520854598));
#18083=CARTESIAN_POINT('Ctrl Pts',(-3.5711249421653,-2.17429031727573,4.47397141948917));
#18084=CARTESIAN_POINT('Ctrl Pts',(-3.39470835638149,-2.30184720512856,
4.46285763043237));
#18085=CARTESIAN_POINT('Ctrl Pts',(-3.40619756140558,-2.51924443916973,
4.45174384137556));
#18086=CARTESIAN_POINT('Ctrl Pts',(-3.59507629381618,-2.62749592593544,
4.44063005231876));
#18087=CARTESIAN_POINT('Ctrl Pts',(-3.78846183549484,-2.52751773117457,
4.42951626326196));
#18088=CARTESIAN_POINT('Ctrl Pts',(-3.80934595131713,-2.31082127219277,
4.41840247420515));
#18089=CARTESIAN_POINT('Ctrl Pts',(-3.63861368521871,-2.17575079119208,
4.40728868514835));
#18090=CARTESIAN_POINT('Ctrl Pts',(-3.43253719137339,-2.24593880082853,
4.39617489609154));
#18091=CARTESIAN_POINT('Ctrl Pts',(-3.37974267459471,-2.45713947835818,
4.38506110703474));
#18092=CARTESIAN_POINT('Ctrl Pts',(-3.52854944397912,-2.61604233624481,
4.37394731797793));
#18093=CARTESIAN_POINT('Ctrl Pts',(-3.74276120758414,-2.57719400158078,
4.36283352892113));
#18094=CARTESIAN_POINT('Ctrl Pts',(-3.82629102553408,-2.37616838455746,
4.35171973986432));
#18095=CARTESIAN_POINT('Ctrl Pts',(-3.70271611525743,-2.19693529644954,
4.34060595080753));
#18096=CARTESIAN_POINT('Ctrl Pts',(-3.48507989312992,-2.2036113246906,4.32949216175072));
#18097=CARTESIAN_POINT('Ctrl Pts',(-3.37271970468676,-2.38996062824249,
4.31837837269391));
#18098=CARTESIAN_POINT('Ctrl Pts',(-3.4682137593984,-2.58566662529692,4.30726458363711));
#18099=CARTESIAN_POINT('Ctrl Pts',(-3.68470210032476,-2.61108979604925,
4.2961507945803));
#18100=CARTESIAN_POINT('Ctrl Pts',(-3.77668287645173,-2.49971922570604,
4.28874160187577));
#18101=CARTESIAN_POINT('Ctrl Pts',(-3.78894936833816,-2.43688906544025,
4.2850370055235));
#18102=CARTESIAN_POINT('Ctrl Pts',(-3.64632995769868,-2.57347832743338,
5.2149629944765));
#18103=CARTESIAN_POINT('Ctrl Pts',(-3.70401562879218,-2.55807251426281,
5.21125839812423));
#18104=CARTESIAN_POINT('Ctrl Pts',(-3.80180511341523,-2.46540693687679,
5.20384920541969));
#18105=CARTESIAN_POINT('Ctrl Pts',(-3.76439491237975,-2.26557452381591,
5.19273541636289));
#18106=CARTESIAN_POINT('Ctrl Pts',(-3.57621918361154,-2.18914809685241,
5.18162162730608));
#18107=CARTESIAN_POINT('Ctrl Pts',(-3.40995490072177,-2.30554054152415,
5.17050783824929));
#18108=CARTESIAN_POINT('Ctrl Pts',(-3.41756896100391,-2.5084803227728,5.15939404919247));
#18109=CARTESIAN_POINT('Ctrl Pts',(-3.59220021318681,-2.6120831620897,5.14828026013568));
#18110=CARTESIAN_POINT('Ctrl Pts',(-3.77395272466994,-2.52158568489689,
5.13716647107886));
#18111=CARTESIAN_POINT('Ctrl Pts',(-3.79649331057924,-2.31978856138657,
5.12605268202207));
#18112=CARTESIAN_POINT('Ctrl Pts',(-3.63917685833343,-2.19141531571474,
5.11493889296526));
#18113=CARTESIAN_POINT('Ctrl Pts',(-3.44600362194169,-2.25395928116791,
5.10382510390846));
#18114=CARTESIAN_POINT('Ctrl Pts',(-3.39378389888927,-2.45017732909347,
5.09271131485166));
#18115=CARTESIAN_POINT('Ctrl Pts',(-3.53031667012352,-2.60046682131627,
5.08159752579484));
#18116=CARTESIAN_POINT('Ctrl Pts',(-3.73063110464943,-2.56726709679655,
5.07048373673805));
#18117=CARTESIAN_POINT('Ctrl Pts',(-3.81137754686683,-2.38096573271764,
5.05936994768124));
#18118=CARTESIAN_POINT('Ctrl Pts',(-3.69864765371964,-2.21208673370492,
5.04825615862444));
#18119=CARTESIAN_POINT('Ctrl Pts',(-3.49562447910673,-2.21520683628489,
5.03714236956762));
#18120=CARTESIAN_POINT('Ctrl Pts',(-3.38813738512521,-2.38747023834909,
5.02602858051084));
#18121=CARTESIAN_POINT('Ctrl Pts',(-3.47457055388411,-2.57120226284288,
5.01491479145402));
#18122=CARTESIAN_POINT('Ctrl Pts',(-3.67581071281477,-2.59823091983783,
5.00380100239722));
#18123=CARTESIAN_POINT('Ctrl Pts',(-3.80766046871388,-2.44381656519338,
4.99268721334042));
#18124=CARTESIAN_POINT('Ctrl Pts',(-3.74943624149071,-2.24929641282234,
4.9815734242836));
#18125=CARTESIAN_POINT('Ctrl Pts',(-3.55443132824748,-2.19271696223645,
4.97045963522681));
#18126=CARTESIAN_POINT('Ctrl Pts',(-3.40113593677424,-2.32586602719142,
4.95934584617));
#18127=CARTESIAN_POINT('Ctrl Pts',(-3.42986307777772,-2.52687075803154,
4.94823205711319));
#18128=CARTESIAN_POINT('Ctrl Pts',(-3.61431847310812,-2.61174924531453,
4.9371182680564));
#18129=CARTESIAN_POINT('Ctrl Pts',(-3.78566800765362,-2.50281124692072,
4.92600447899958));
#18130=CARTESIAN_POINT('Ctrl Pts',(-3.78707350915862,-2.29976894828182,
4.91489068994279));
#18131=CARTESIAN_POINT('Ctrl Pts',(-3.6172485061812,-2.18846926796789,4.90377690088598));
#18132=CARTESIAN_POINT('Ctrl Pts',(-3.43163574988059,-2.27078606560966,
4.89266311182917));
#18133=CARTESIAN_POINT('Ctrl Pts',(-3.40012870109683,-2.47137384278207,
4.88154932277237));
#18134=CARTESIAN_POINT('Ctrl Pts',(-3.55156611889279,-2.60663233222288,
4.87043553371556));
#18135=CARTESIAN_POINT('Ctrl Pts',(-3.74733561734428,-2.55275790460943,
4.85932174465877));
#18136=CARTESIAN_POINT('Ctrl Pts',(-3.80824715434074,-2.35906243451482,
4.84820795560196));
#18137=CARTESIAN_POINT('Ctrl Pts',(-3.6785477092859,-2.2028375823722,4.83709416654515));
#18138=CARTESIAN_POINT('Ctrl Pts',(-3.47695265513,-2.22707772705829,4.82598037748836));
#18139=CARTESIAN_POINT('Ctrl Pts',(-3.38798423118545,-2.40959558923983,
4.81486658843155));
#18140=CARTESIAN_POINT('Ctrl Pts',(-3.49307624485919,-2.5833304997688,4.80375279937474));
#18141=CARTESIAN_POINT('Ctrl Pts',(-3.69603678421119,-2.5892609247501,4.79263901031794));
#18142=CARTESIAN_POINT('Ctrl Pts',(-3.81109376584347,-2.42195867894277,
4.78152522126113));
#18143=CARTESIAN_POINT('Ctrl Pts',(-3.7329342296331,-2.23455740527076,4.77041143220433));
#18144=CARTESIAN_POINT('Ctrl Pts',(-3.53309848546286,-2.19858761480107,
4.75929764314753));
#18145=CARTESIAN_POINT('Ctrl Pts',(-3.39449845626323,-2.34697286467576,
4.74818385409072));
#18146=CARTESIAN_POINT('Ctrl Pts',(-3.4439963205919,-2.54389445288135,4.73707006503392));
#18147=CARTESIAN_POINT('Ctrl Pts',(-3.63628612188485,-2.60910781649055,
4.72595627597711));
#18148=CARTESIAN_POINT('Ctrl Pts',(-3.79536282430398,-2.48292242422203,
4.71484248692031));
#18149=CARTESIAN_POINT('Ctrl Pts',(-3.77562171807257,-2.28083719665882,
4.7037286978635));
#18150=CARTESIAN_POINT('Ctrl Pts',(-3.59513206160358,-2.18782303439192,
4.6926149088067));
#18151=CARTESIAN_POINT('Ctrl Pts',(-3.41909808435503,-2.28901685499652,
4.6815011197499));
#18152=CARTESIAN_POINT('Ctrl Pts',(-3.40864568206353,-2.49179480685731,
4.67038733069309));
#18153=CARTESIAN_POINT('Ctrl Pts',(-3.57334205708494,-2.61055193097763,
4.65927354163629));
#18154=CARTESIAN_POINT('Ctrl Pts',(-3.76243874957797,-2.53658848485295,
4.64815975257949));
#18155=CARTESIAN_POINT('Ctrl Pts',(-3.80285341240188,-2.33760404952332,
4.63704596352268));
#18156=CARTESIAN_POINT('Ctrl Pts',(-3.65759404633958,-2.19573133528376,
4.62593217446587));
#18157=CARTESIAN_POINT('Ctrl Pts',(-3.45961819650295,-2.24082804642207,
4.61481838540908));
#18158=CARTESIAN_POINT('Ctrl Pts',(-3.39013540344272,-2.43161665180523,
4.60370459635226));
#18159=CARTESIAN_POINT('Ctrl Pts',(-3.51274405564254,-2.59346617722935,
4.59259080729546));
#18160=CARTESIAN_POINT('Ctrl Pts',(-3.71521906325291,-2.57823391658879,
4.58147701823866));
#18161=CARTESIAN_POINT('Ctrl Pts',(-3.81223275561396,-2.39986213076634,
4.57036322918186));
#18162=CARTESIAN_POINT('Ctrl Pts',(-3.71498739984013,-2.2216165382532,4.55924944012505));
#18163=CARTESIAN_POINT('Ctrl Pts',(-3.51249277302345,-2.20664735121048,
4.54813565106825));
#18164=CARTESIAN_POINT('Ctrl Pts',(-3.39009450330442,-2.36865603651811,
4.53702186201144));
#18165=CARTESIAN_POINT('Ctrl Pts',(-3.45982511550835,-2.55935420677483,
4.52590807295464));
#18166=CARTESIAN_POINT('Ctrl Pts',(-3.65785938856352,-2.60419366495283,
4.51479428389783));
#18167=CARTESIAN_POINT('Ctrl Pts',(-3.80293430832847,-2.46213234472064,
4.50368049484103));
#18168=CARTESIAN_POINT('Ctrl Pts',(-3.76226115178167,-2.26320058707017,
4.49256670578422));
#18169=CARTESIAN_POINT('Ctrl Pts',(-3.57306852778269,-2.1894828788131,4.48145291672742));
#18170=CARTESIAN_POINT('Ctrl Pts',(-3.40852657583551,-2.30845388836054,
4.47033912767062));
#18171=CARTESIAN_POINT('Ctrl Pts',(-3.41924244029115,-2.51121807336119,
4.45922533861381));
#18172=CARTESIAN_POINT('Ctrl Pts',(-3.59540770941291,-2.61218313202887,
4.44811154955701));
#18173=CARTESIAN_POINT('Ctrl Pts',(-3.77577643361645,-2.51893448851262,
4.4369977605002));
#18174=CARTESIAN_POINT('Ctrl Pts',(-3.79525483564324,-2.31682390926922,
4.42588397144341));
#18175=CARTESIAN_POINT('Ctrl Pts',(-3.63601459074572,-2.19084504795324,
4.41477018238659));
#18176=CARTESIAN_POINT('Ctrl Pts',(-3.44380914477199,-2.25630868935384,
4.4036563933298));
#18177=CARTESIAN_POINT('Ctrl Pts',(-3.3945682369272,-2.45329340923659,4.39254260427298));
#18178=CARTESIAN_POINT('Ctrl Pts',(-3.53335879445148,-2.60150048563184,
4.38142881521619));
#18179=CARTESIAN_POINT('Ctrl Pts',(-3.73315192363498,-2.56526703973946,
4.37031502615937));
#18180=CARTESIAN_POINT('Ctrl Pts',(-3.81105933370197,-2.37777249511123,
4.35920123710258));
#18181=CARTESIAN_POINT('Ctrl Pts',(-3.69580227406509,-2.21060362014537,
4.34808744804577));
#18182=CARTESIAN_POINT('Ctrl Pts',(-3.49281518731151,-2.21683028365978,
4.33697365898897));
#18183=CARTESIAN_POINT('Ctrl Pts',(-3.38801798445527,-2.3906363802589,4.32585986993216));
#18184=CARTESIAN_POINT('Ctrl Pts',(-3.47708431623917,-2.57316936954691,
4.31474608087536));
#18185=CARTESIAN_POINT('Ctrl Pts',(-3.6790007858929,-2.59688130185582,4.30363229181855));
#18186=CARTESIAN_POINT('Ctrl Pts',(-3.76479031853975,-2.4930071057176,4.29622309911402));
#18187=CARTESIAN_POINT('Ctrl Pts',(-3.77623115053166,-2.43440605545153,
4.29251850276175));
#18188=CARTESIAN_POINT('Ctrl Pts',(-3.64298642568859,-2.56095877486649,
5.22244449171475));
#18189=CARTESIAN_POINT('Ctrl Pts',(-3.69650904770099,-2.54666476563522,
5.21873989536248));
#18190=CARTESIAN_POINT('Ctrl Pts',(-3.78724127847948,-2.46068666088276,
5.21133070265795));
#18191=CARTESIAN_POINT('Ctrl Pts',(-3.75253089006804,-2.27527571727515,
5.20021691360113));
#18192=CARTESIAN_POINT('Ctrl Pts',(-3.57793539326875,-2.20436481887379,
5.18910312454434));
#18193=CARTESIAN_POINT('Ctrl Pts',(-3.42367004108366,-2.31235747464383,
5.17798933548752));
#18194=CARTESIAN_POINT('Ctrl Pts',(-3.43073461124009,-2.5006515344537,5.16687554643073));
#18195=CARTESIAN_POINT('Ctrl Pts',(-3.59276310679123,-2.59677758279563,
5.15576175737392));
#18196=CARTESIAN_POINT('Ctrl Pts',(-3.76139893588905,-2.51281111117365,
5.14464796831712));
#18197=CARTESIAN_POINT('Ctrl Pts',(-3.78231281687012,-2.32557724598507,
5.13353417926031));
#18198=CARTESIAN_POINT('Ctrl Pts',(-3.63634954990495,-2.2064684174952,5.12242039020351));
#18199=CARTESIAN_POINT('Ctrl Pts',(-3.4571172047087,-2.26449872135838,5.1113066011467));
#18200=CARTESIAN_POINT('Ctrl Pts',(-3.40866606518746,-2.44655614068022,
5.10019281208991));
#18201=CARTESIAN_POINT('Ctrl Pts',(-3.53534556407432,-2.58599956800273,
5.08907902303309));
#18202=CARTESIAN_POINT('Ctrl Pts',(-3.72120374270903,-2.55519579519918,
5.0779652339763));
#18203=CARTESIAN_POINT('Ctrl Pts',(-3.79612289028458,-2.3823393942772,5.06685144491949));
#18204=CARTESIAN_POINT('Ctrl Pts',(-3.69152846768288,-2.22564802432955,
5.05573765586268));
#18205=CARTESIAN_POINT('Ctrl Pts',(-3.503157032826,-2.22854295591068,5.04462386680587));
#18206=CARTESIAN_POINT('Ctrl Pts',(-3.40342704800776,-2.38837448392236,
5.03351007774909));
#18207=CARTESIAN_POINT('Ctrl Pts',(-3.483622523472,-2.55884696889381,5.02239628869226));
#18208=CARTESIAN_POINT('Ctrl Pts',(-3.670339619,-2.58392502665791,5.01128249963547));
#18209=CARTESIAN_POINT('Ctrl Pts',(-3.79267406555566,-2.44065441923915,
5.00016871057867));
#18210=CARTESIAN_POINT('Ctrl Pts',(-3.73865175383498,-2.26017236205245,
4.98905492152186));
#18211=CARTESIAN_POINT('Ctrl Pts',(-3.55771991991106,-2.20767612702608,
4.97794113246506));
#18212=CARTESIAN_POINT('Ctrl Pts',(-3.4154875225317,-2.3312161143366,4.96682734340825));
#18213=CARTESIAN_POINT('Ctrl Pts',(-3.44214148841752,-2.51771477210593,
4.95571355435145));
#18214=CARTESIAN_POINT('Ctrl Pts',(-3.61328514012983,-2.59646776406591,
4.94459976529465));
#18215=CARTESIAN_POINT('Ctrl Pts',(-3.77226875244865,-2.49539158344266,
4.93348597623784));
#18216=CARTESIAN_POINT('Ctrl Pts',(-3.77357282197517,-2.30700240469905,
4.92237218718103));
#18217=CARTESIAN_POINT('Ctrl Pts',(-3.61600371910589,-2.20373497958946,
4.91125839812423));
#18218=CARTESIAN_POINT('Ctrl Pts',(-3.44378623064059,-2.28011115346305,
4.90014460906743));
#18219=CARTESIAN_POINT('Ctrl Pts',(-3.41455297685654,-2.46622294820157,
4.88903082001062));
#18220=CARTESIAN_POINT('Ctrl Pts',(-3.555061486467,-2.59172012743304,4.87791703095382));
#18221=CARTESIAN_POINT('Ctrl Pts',(-3.73670272715212,-2.54173369977035,
4.86680324189701));
#18222=CARTESIAN_POINT('Ctrl Pts',(-3.79321841136028,-2.36201680933867,
4.85568945284021));
#18223=CARTESIAN_POINT('Ctrl Pts',(-3.67287909240468,-2.21706636407783,
4.8445756637834));
#18224=CARTESIAN_POINT('Ctrl Pts',(-3.48583271366589,-2.23955715038517,
4.83346187472661));
#18225=CARTESIAN_POINT('Ctrl Pts',(-3.40328494685383,-2.40890309649059,
4.82234808566979));
#18226=CARTESIAN_POINT('Ctrl Pts',(-3.50079269908688,-2.57009993741021,
4.811234296613));
#18227=CARTESIAN_POINT('Ctrl Pts',(-3.68910601893303,-2.57560237655376,
4.80012050755619));
#18228=CARTESIAN_POINT('Ctrl Pts',(-3.79585958911879,-2.42037396897126,
4.78900671849938));
#18229=CARTESIAN_POINT('Ctrl Pts',(-3.72334065618531,-2.24649703653284,
4.77789292944258));
#18230=CARTESIAN_POINT('Ctrl Pts',(-3.53792662186724,-2.21312310739792,
4.76677914038578));
#18231=CARTESIAN_POINT('Ctrl Pts',(-3.40932905451407,-2.35079971738979,
4.75566535132897));
#18232=CARTESIAN_POINT('Ctrl Pts',(-3.45525476591977,-2.53350990402394,
4.74455156227217));
#18233=CARTESIAN_POINT('Ctrl Pts',(-3.6336674316017,-2.59401696139969,4.73343777321536));
#18234=CARTESIAN_POINT('Ctrl Pts',(-3.78126391532395,-2.47693809370431,
4.72232398415856));
#18235=CARTESIAN_POINT('Ctrl Pts',(-3.76294748167758,-2.28943691630404,
4.71121019510175));
#18236=CARTESIAN_POINT('Ctrl Pts',(-3.59548337010158,-2.20313538328135,
4.70009640604495));
#18237=CARTESIAN_POINT('Ctrl Pts',(-3.43215338109369,-2.29702626653782,
4.68898261698815));
#18238=CARTESIAN_POINT('Ctrl Pts',(-3.42245530588083,-2.48517017583382,
4.67786882793134));
#18239=CARTESIAN_POINT('Ctrl Pts',(-3.5752659026891,-2.59535685729358,4.66675503887453));
#18240=CARTESIAN_POINT('Ctrl Pts',(-3.75071589926964,-2.5267311917752,4.65564124981774));
#18241=CARTESIAN_POINT('Ctrl Pts',(-3.7882139240144,-2.34210702919526,4.64452746076093));
#18242=CARTESIAN_POINT('Ctrl Pts',(-3.65343760961716,-2.21047295934436,
4.63341367170412));
#18243=CARTESIAN_POINT('Ctrl Pts',(-3.46974924511472,-2.25231513918736,
4.62229988264733));
#18244=CARTESIAN_POINT('Ctrl Pts',(-3.4052808737006,-2.42933494699449,4.61118609359051));
#18245=CARTESIAN_POINT('Ctrl Pts',(-3.51904112685782,-2.57950414513246,
4.60007230453372));
#18246=CARTESIAN_POINT('Ctrl Pts',(-3.7069039547293,-2.5653711635236,4.5889585154769));
#18247=CARTESIAN_POINT('Ctrl Pts',(-3.79691638048147,-2.39987208048827,
4.57784472642011));
#18248=CARTESIAN_POINT('Ctrl Pts',(-3.7066890099598,-2.23449008366631,4.5667309373633));
#18249=CARTESIAN_POINT('Ctrl Pts',(-3.51880797875736,-2.22060119020745,
4.5556171483065));
#18250=CARTESIAN_POINT('Ctrl Pts',(-3.40524292523608,-2.37091806200724,
4.54450335924969));
#18251=CARTESIAN_POINT('Ctrl Pts',(-3.46994123122676,-2.54785396119378,
4.53338957019289));
#18252=CARTESIAN_POINT('Ctrl Pts',(-3.65368380267146,-2.5894574534616,4.52227578113609));
#18253=CARTESIAN_POINT('Ctrl Pts',(-3.78828898185839,-2.45764838890124,
4.51116199207927));
#18254=CARTESIAN_POINT('Ctrl Pts',(-3.75055111831899,-2.27307310236724,
4.50004820302248));
#18255=CARTESIAN_POINT('Ctrl Pts',(-3.57501211340008,-2.20467544035046,
4.48893441396567));
#18256=CARTESIAN_POINT('Ctrl Pts',(-3.42234479528953,-2.31506057159251,
4.47782062490887));
#18257=CARTESIAN_POINT('Ctrl Pts',(-3.43228731917671,-2.50319170755265,
4.46670683585206));
#18258=CARTESIAN_POINT('Ctrl Pts',(-3.59573912500965,-2.5968703381223,4.45559304679526));
#18259=CARTESIAN_POINT('Ctrl Pts',(-3.76309103173807,-2.51035124585066,
4.44447925773846));
#18260=CARTESIAN_POINT('Ctrl Pts',(-3.78116371996935,-2.32282654634568,
4.43336546868165));
#18261=CARTESIAN_POINT('Ctrl Pts',(-3.63341549627273,-2.20593930471439,
4.42225167962485));
#18262=CARTESIAN_POINT('Ctrl Pts',(-3.45508109817058,-2.26667857787915,
4.41113789056804));
#18263=CARTESIAN_POINT('Ctrl Pts',(-3.40939379925969,-2.449447340115,4.40002410151124));
#18264=CARTESIAN_POINT('Ctrl Pts',(-3.53816814492384,-2.58695863501888,
4.38891031245443));
#18265=CARTESIAN_POINT('Ctrl Pts',(-3.72354263968583,-2.55334007789814,
4.37779652339763));
#18266=CARTESIAN_POINT('Ctrl Pts',(-3.79582764186986,-2.379376605665,4.36668273434082));
#18267=CARTESIAN_POINT('Ctrl Pts',(-3.68888843287276,-2.22427194384119,
4.35556894528402));
#18268=CARTESIAN_POINT('Ctrl Pts',(-3.50055048149309,-2.23004924262897,
4.34445515622722));
#18269=CARTESIAN_POINT('Ctrl Pts',(-3.40331626422378,-2.3913121322753,4.33334136717041));
#18270=CARTESIAN_POINT('Ctrl Pts',(-3.48595487307994,-2.5606721137969,4.32222757811361));
#18271=CARTESIAN_POINT('Ctrl Pts',(-3.67329947146103,-2.58267280766239,
4.3111137890568));
#18272=CARTESIAN_POINT('Ctrl Pts',(-3.75289776062778,-2.48629498572916,
4.30370459635227));
#18273=CARTESIAN_POINT('Ctrl Pts',(-3.76351293272515,-2.4319230454628,4.3));
#18274=CARTESIAN_POINT('Ctrl Pts',(-3.76638442554721,-2.39990578503699,
5.13785196366098));
#18275=CARTESIAN_POINT('Ctrl Pts',(-3.76649613683224,-2.3783172805639,5.13641270219409));
#18276=CARTESIAN_POINT('Ctrl Pts',(-3.76259705167907,-2.35676746354197,
5.1349734407272));
#18277=CARTESIAN_POINT('Ctrl Pts',(-3.75449995887908,-2.33693141876819,
5.13353417926032));
#18278=CARTESIAN_POINT('Ctrl Pts',(-3.73365839454839,-2.28587430315511,
5.12982958290805));
#18279=CARTESIAN_POINT('Ctrl Pts',(-3.68500397222667,-2.24617136032516,
5.12612498655578));
#18280=CARTESIAN_POINT('Ctrl Pts',(-3.6308047035331,-2.23599160622071,5.12242039020351));
#18281=CARTESIAN_POINT('Ctrl Pts',(-3.57660543483953,-2.22581185211626,
5.11871579385124));
#18282=CARTESIAN_POINT('Ctrl Pts',(-3.51686131977411,-2.24515528673732,
5.11501119749897));
#18283=CARTESIAN_POINT('Ctrl Pts',(-3.4789140723212,-2.28516990726816,5.1113066011467));
#18284=CARTESIAN_POINT('Ctrl Pts',(-3.44096682486829,-2.32518452779899,
5.10760200479444));
#18285=CARTESIAN_POINT('Ctrl Pts',(-3.42481644502788,-2.3858703342396,5.10389740844217));
#18286=CARTESIAN_POINT('Ctrl Pts',(-3.43785450492215,-2.43945380868033,
5.1001928120899));
#18287=CARTESIAN_POINT('Ctrl Pts',(-3.45089256481642,-2.49303728312105,
5.09648821573763));
#18288=CARTESIAN_POINT('Ctrl Pts',(-3.49311906444537,-2.53951842556189,
5.09278361938536));
#18289=CARTESIAN_POINT('Ctrl Pts',(-3.54520867736563,-2.55762503464839,
5.08907902303309));
#18290=CARTESIAN_POINT('Ctrl Pts',(-3.59729829028589,-2.57573164373488,
5.08537442668083));
#18291=CARTESIAN_POINT('Ctrl Pts',(-3.65925101649746,-2.56546371946703,
5.08166983032856));
#18292=CARTESIAN_POINT('Ctrl Pts',(-3.70271390419917,-2.53152035717944,
5.07796523397629));
#18293=CARTESIAN_POINT('Ctrl Pts',(-3.74226404589835,-2.50063274572034,
5.07459414387119));
#18294=CARTESIAN_POINT('Ctrl Pts',(-3.76650359324528,-2.4501405807959,5.07122305376609));
#18295=CARTESIAN_POINT('Ctrl Pts',(-3.7668206250807,-2.39991359866148,5.06785196366098));
#18296=CARTESIAN_POINT('Ctrl Pts',(-3.65301702171886,-2.59851743256717,
5.2));
#18297=CARTESIAN_POINT('Ctrl Pts',(-3.66542047324148,-2.59392489431986,
5.2));
#18298=CARTESIAN_POINT('Ctrl Pts',(-3.67726976851323,-2.58806562778896,
5.2));
#18299=CARTESIAN_POINT('Ctrl Pts',(-3.6884471572875,-2.58110287343,5.2));
#18300=CARTESIAN_POINT('Ctrl Pts',(-3.69411332072466,-2.57757323829184,
5.2));
#18301=CARTESIAN_POINT('Ctrl Pts',(-3.69960638117381,-2.57375928297626,
5.2));
#18302=CARTESIAN_POINT('Ctrl Pts',(-3.70490756348411,-2.56967869660782,
5.2));
#18303=CARTESIAN_POINT('Ctrl Pts',(-3.7094943667238,-2.56614800370216,5.2));
#18304=CARTESIAN_POINT('Ctrl Pts',(-3.71393749668481,-2.56241764644412,
5.2));
#18305=CARTESIAN_POINT('Ctrl Pts',(-3.71822298464189,-2.55849819748795,
5.2));
#18306=CARTESIAN_POINT('Ctrl Pts',(-3.7213335990699,-2.55565327187038,5.2));
#18307=CARTESIAN_POINT('Ctrl Pts',(-3.72435497328541,-2.55271413748664,
5.2));
#18308=CARTESIAN_POINT('Ctrl Pts',(-3.72727770073803,-2.54969101779411,
5.2));
#18309=CARTESIAN_POINT('Ctrl Pts',(-3.73622270492435,-2.54043876326685,
5.2));
#18310=CARTESIAN_POINT('Ctrl Pts',(-3.7442634301432,-2.53038665580988,5.2));
#18311=CARTESIAN_POINT('Ctrl Pts',(-3.75126083636282,-2.51966573521934,
5.2));
#18312=CARTESIAN_POINT('Ctrl Pts',(-3.75579169616378,-2.51272387896453,
5.2));
#18313=CARTESIAN_POINT('Ctrl Pts',(-3.75988429343086,-2.5055010355982,5.2));
#18314=CARTESIAN_POINT('Ctrl Pts',(-3.76348914806144,-2.49803012759629,
5.2));
#18315=CARTESIAN_POINT('Ctrl Pts',(-3.76515593070928,-2.49457579140323,
5.2));
#18316=CARTESIAN_POINT('Ctrl Pts',(-3.76671430859645,-2.49107651026494,
5.2));
#18317=CARTESIAN_POINT('Ctrl Pts',(-3.76815914917795,-2.48753923965477,
5.2));
#18318=CARTESIAN_POINT('Ctrl Pts',(-3.77216127817835,-2.47774119447769,
5.2));
#18319=CARTESIAN_POINT('Ctrl Pts',(-3.77529843764987,-2.46764366345261,
5.2));
#18320=CARTESIAN_POINT('Ctrl Pts',(-3.77747651250232,-2.45732003292749,
5.2));
#18321=CARTESIAN_POINT('Ctrl Pts',(-3.779330303747,-2.44853344055707,5.2));
#18322=CARTESIAN_POINT('Ctrl Pts',(-3.78048859875581,-2.43958258054595,
5.2));
#18323=CARTESIAN_POINT('Ctrl Pts',(-3.78096402676373,-2.43054575199388,
5.2));
#18324=CARTESIAN_POINT('Ctrl Pts',(-3.78113316899519,-2.42733073453364,
5.2));
#18325=CARTESIAN_POINT('Ctrl Pts',(-3.78121551844131,-2.4241062749112,5.2));
#18326=CARTESIAN_POINT('Ctrl Pts',(-3.78121200526832,-2.42088560814198,
5.2));
#18327=CARTESIAN_POINT('Ctrl Pts',(-3.78119923320481,-2.40917694458053,
5.2));
#18328=CARTESIAN_POINT('Ctrl Pts',(-3.78005717128054,-2.39748206272171,
5.2));
#18329=CARTESIAN_POINT('Ctrl Pts',(-3.77783120534438,-2.38597327518306,
5.2));
#18330=CARTESIAN_POINT('Ctrl Pts',(-3.77668820057652,-2.38006366137664,
5.2));
#18331=CARTESIAN_POINT('Ctrl Pts',(-3.77525871074905,-2.37420329819383,
5.2));
#18332=CARTESIAN_POINT('Ctrl Pts',(-3.77354495279965,-2.36841778018193,
5.2));
#18333=CARTESIAN_POINT('Ctrl Pts',(-3.771857709037,-2.36272177207139,5.2));
#18334=CARTESIAN_POINT('Ctrl Pts',(-3.76989216970551,-2.35709287385817,
5.2));
#18335=CARTESIAN_POINT('Ctrl Pts',(-3.76766230775392,-2.35158840548752,
5.2));
#18336=CARTESIAN_POINT('Ctrl Pts',(-3.76420558159522,-2.34305539303218,
5.2));
#18337=CARTESIAN_POINT('Ctrl Pts',(-3.76011199819993,-2.33480777321703,
5.2));
#18338=CARTESIAN_POINT('Ctrl Pts',(-3.75539090007917,-2.32694141045687,
5.2));
#18339=CARTESIAN_POINT('Ctrl Pts',(-3.75297689160326,-2.32291915421652,
5.2));
#18340=CARTESIAN_POINT('Ctrl Pts',(-3.75039789394566,-2.31899648610286,
5.2));
#18341=CARTESIAN_POINT('Ctrl Pts',(-3.74766394659108,-2.31519991459367,
5.2));
#18342=CARTESIAN_POINT('Ctrl Pts',(-3.7422293448357,-2.30765300475514,5.2));
#18343=CARTESIAN_POINT('Ctrl Pts',(-3.73617584795258,-2.30058959872182,
5.2));
#18344=CARTESIAN_POINT('Ctrl Pts',(-3.7295081063639,-2.29412082362908,5.2));
#18345=CARTESIAN_POINT('Ctrl Pts',(-3.72872963705521,-2.29336558397147,
5.2));
#18346=CARTESIAN_POINT('Ctrl Pts',(-3.72794278071792,-2.29261847520289,
5.2));
#18347=CARTESIAN_POINT('Ctrl Pts',(-3.72714769448934,-2.29187956305505,
5.2));
#18348=CARTESIAN_POINT('Origin',(-3.6,-2.4,4.7));
#18349=CARTESIAN_POINT('Origin',(3.6,-2.4,4.3));
#18350=CARTESIAN_POINT('Ctrl Pts',(3.43648706727485,-2.43192304546281,4.3));
#18351=CARTESIAN_POINT('Ctrl Pts',(3.43713128683253,-2.44021936733391,4.3));
#18352=CARTESIAN_POINT('Ctrl Pts',(3.43844438912273,-2.44842976439641,4.3));
#18353=CARTESIAN_POINT('Ctrl Pts',(3.44036779101517,-2.45650290183658,4.3));
#18354=CARTESIAN_POINT('Ctrl Pts',(3.44142971550231,-2.46096014104879,4.3));
#18355=CARTESIAN_POINT('Ctrl Pts',(3.44267796071139,-2.46537560589173,4.3));
#18356=CARTESIAN_POINT('Ctrl Pts',(3.44410466214797,-2.4697408265362,4.3));
#18357=CARTESIAN_POINT('Ctrl Pts',(3.44564437628146,-2.47445182755564,4.3));
#18358=CARTESIAN_POINT('Ctrl Pts',(3.44738954450943,-2.47909640503965,4.3));
#18359=CARTESIAN_POINT('Ctrl Pts',(3.44932653760859,-2.48365784749895,4.3));
#18360=CARTESIAN_POINT('Ctrl Pts',(3.45254730792056,-2.49124246845553,4.3));
#18361=CARTESIAN_POINT('Ctrl Pts',(3.45629958145885,-2.49860290469935,4.3));
#18362=CARTESIAN_POINT('Ctrl Pts',(3.460540361967,-2.50569093557372,4.3));
#18363=CARTESIAN_POINT('Ctrl Pts',(3.46239352486579,-2.50878830781843,4.3));
#18364=CARTESIAN_POINT('Ctrl Pts',(3.46433983439221,-2.51183274422802,4.3));
#18365=CARTESIAN_POINT('Ctrl Pts',(3.46636982169588,-2.5148117549636,4.3));
#18366=CARTESIAN_POINT('Ctrl Pts',(3.4732458122516,-2.52490228589753,4.3));
#18367=CARTESIAN_POINT('Ctrl Pts',(3.48109363537456,-2.5342702737356,4.3));
#18368=CARTESIAN_POINT('Ctrl Pts',(3.4897794934809,-2.54276723354547,4.3));
#18369=CARTESIAN_POINT('Ctrl Pts',(3.49400930325249,-2.54690505426423,4.3));
#18370=CARTESIAN_POINT('Ctrl Pts',(3.49843862851918,-2.55083612678489,4.3));
#18371=CARTESIAN_POINT('Ctrl Pts',(3.50305595405548,-2.55454125034048,4.3));
#18372=CARTESIAN_POINT('Ctrl Pts',(3.50696190635494,-2.55767554004086,4.3));
#18373=CARTESIAN_POINT('Ctrl Pts',(3.51100694759131,-2.56065060854479,4.3));
#18374=CARTESIAN_POINT('Ctrl Pts',(3.51515869554757,-2.56343734237232,4.3));
#18375=CARTESIAN_POINT('Ctrl Pts',(3.52023397904373,-2.56684397118314,4.3));
#18376=CARTESIAN_POINT('Ctrl Pts',(3.52547419237578,-2.56997446151731,4.3));
#18377=CARTESIAN_POINT('Ctrl Pts',(3.53086407609141,-2.57281069688687,4.3));
#18378=CARTESIAN_POINT('Ctrl Pts',(3.53843716228638,-2.57679576522158,4.3));
#18379=CARTESIAN_POINT('Ctrl Pts',(3.5463054085634,-2.58020053156405,4.3));
#18380=CARTESIAN_POINT('Ctrl Pts',(3.55440202217605,-2.58304072456499,4.3));
#18381=CARTESIAN_POINT('Ctrl Pts',(3.56031216163472,-2.58511392918216,4.3));
#18382=CARTESIAN_POINT('Ctrl Pts',(3.5663442123363,-2.58688610080112,4.3));
#18383=CARTESIAN_POINT('Ctrl Pts',(3.57247443059928,-2.58835971156752,4.3));
#18384=CARTESIAN_POINT('Ctrl Pts',(3.57600236806727,-2.58920777380822,4.3));
#18385=CARTESIAN_POINT('Ctrl Pts',(3.57955832823423,-2.58995565186198,4.3));
#18386=CARTESIAN_POINT('Ctrl Pts',(3.58312950627136,-2.59060308036101,4.3));
#18387=CARTESIAN_POINT('Ctrl Pts',(3.59464642713376,-2.59269101400921,4.3));
#18388=CARTESIAN_POINT('Ctrl Pts',(3.6063444588111,-2.59374267077427,4.3));
#18389=CARTESIAN_POINT('Ctrl Pts',(3.61806681517941,-2.59379134323091,4.3));
#18390=CARTESIAN_POINT('Ctrl Pts',(3.62473112824741,-2.59381901415975,4.3));
#18391=CARTESIAN_POINT('Ctrl Pts',(3.63140369181744,-2.59352192189353,4.3));
#18392=CARTESIAN_POINT('Ctrl Pts',(3.63805736597901,-2.59290136699938,4.3));
#18393=CARTESIAN_POINT('Ctrl Pts',(3.64215429545284,-2.59251926688834,4.3));
#18394=CARTESIAN_POINT('Ctrl Pts',(3.64624613464129,-2.59201413768455,4.3));
#18395=CARTESIAN_POINT('Ctrl Pts',(3.65032004640889,-2.59138662655135,4.3));
#18396=CARTESIAN_POINT('Ctrl Pts',(3.6635759835922,-2.58934479338508,4.3));
#18397=CARTESIAN_POINT('Ctrl Pts',(3.67655554403262,-2.58602558677096,4.3));
#18398=CARTESIAN_POINT('Ctrl Pts',(3.68904453335804,-2.58146163637399,4.3));
#18399=CARTESIAN_POINT('Ctrl Pts',(3.69937751045428,-2.5776855746214,4.3));
#18400=CARTESIAN_POINT('Ctrl Pts',(3.70937567296629,-2.57305657585047,4.3));
#18401=CARTESIAN_POINT('Ctrl Pts',(3.7189159065364,-2.56756614624894,4.3));
#18402=CARTESIAN_POINT('Ctrl Pts',(3.72007018633274,-2.56690185517936,4.3));
#18403=CARTESIAN_POINT('Ctrl Pts',(3.72121775119647,-2.56622492375,4.3));
#18404=CARTESIAN_POINT('Ctrl Pts',(3.72235852099786,-2.56553552032368,4.3));
#18405=CARTESIAN_POINT('Ctrl Pts',(3.78826275096637,-2.48232321801033,4.3));
#18406=CARTESIAN_POINT('Ctrl Pts',(3.79091867325729,-2.4742706313139,4.3));
#18407=CARTESIAN_POINT('Ctrl Pts',(3.79302804122654,-2.46606039506531,4.3));
#18408=CARTESIAN_POINT('Ctrl Pts',(3.79460324133206,-2.45774386615892,4.3));
#18409=CARTESIAN_POINT('Ctrl Pts',(3.79578956705146,-2.45148046374845,4.3));
#18410=CARTESIAN_POINT('Ctrl Pts',(3.79667272255332,-2.44515671383718,4.3));
#18411=CARTESIAN_POINT('Ctrl Pts',(3.79725488779627,-2.43879482378833,4.3));
#18412=CARTESIAN_POINT('Ctrl Pts',(3.79769087373759,-2.43403037820329,4.3));
#18413=CARTESIAN_POINT('Ctrl Pts',(3.79795758751143,-2.42924591021267,4.3));
#18414=CARTESIAN_POINT('Ctrl Pts',(3.79805591662036,-2.4244630110418,4.3));
#18415=CARTESIAN_POINT('Ctrl Pts',(3.79826160078478,-2.41445817493456,4.3));
#18416=CARTESIAN_POINT('Ctrl Pts',(3.79773307923007,-2.40444525216584,4.3));
#18417=CARTESIAN_POINT('Ctrl Pts',(3.7964780509907,-2.39451257334247,4.3));
#18418=CARTESIAN_POINT('Ctrl Pts',(3.79582248849211,-2.38932425044823,4.3));
#18419=CARTESIAN_POINT('Ctrl Pts',(3.7949674129287,-2.38415491083777,4.3));
#18420=CARTESIAN_POINT('Ctrl Pts',(3.79391844712734,-2.37904222861684,4.3));
#18421=CARTESIAN_POINT('Ctrl Pts',(3.79135149974265,-2.3665308710123,4.3));
#18422=CARTESIAN_POINT('Ctrl Pts',(3.78762424888679,-2.35432630792998,4.3));
#18423=CARTESIAN_POINT('Ctrl Pts',(3.78275036269461,-2.34261709433331,4.3));
#18424=CARTESIAN_POINT('Ctrl Pts',(3.78051279286925,-2.33724146962858,4.3));
#18425=CARTESIAN_POINT('Ctrl Pts',(3.77803293300414,-2.33197059787363,4.3));
#18426=CARTESIAN_POINT('Ctrl Pts',(3.77530918258224,-2.32682518237142,4.3));
#18427=CARTESIAN_POINT('Ctrl Pts',(3.77352855433059,-2.32346141154425,4.3));
#18428=CARTESIAN_POINT('Ctrl Pts',(3.77164258388613,-2.32014955771335,4.3));
#18429=CARTESIAN_POINT('Ctrl Pts',(3.76965386637616,-2.31690144569075,4.3));
#18430=CARTESIAN_POINT('Ctrl Pts',(3.76538144816038,-2.30992343453397,4.3));
#18431=CARTESIAN_POINT('Ctrl Pts',(3.76065257819642,-2.3032660772289,4.3));
#18432=CARTESIAN_POINT('Ctrl Pts',(3.7554693784929,-2.29698171698016,4.3));
#18433=CARTESIAN_POINT('Ctrl Pts',(3.74976402854315,-2.29006427669614,4.3));
#18434=CARTESIAN_POINT('Ctrl Pts',(3.74350800901797,-2.28359846633093,4.3));
#18435=CARTESIAN_POINT('Ctrl Pts',(3.73677358655615,-2.27761728545388,4.3));
#18436=CARTESIAN_POINT('Ctrl Pts',(3.73252958089122,-2.2738479695743,4.3));
#18437=CARTESIAN_POINT('Ctrl Pts',(3.72809540845025,-2.27027136680987,4.3));
#18438=CARTESIAN_POINT('Ctrl Pts',(3.72348829039508,-2.26689850911598,4.3));
#18439=CARTESIAN_POINT('Ctrl Pts',(3.72067474538276,-2.26483872101672,4.3));
#18440=CARTESIAN_POINT('Ctrl Pts',(3.71780010895487,-2.26285764263401,4.3));
#18441=CARTESIAN_POINT('Ctrl Pts',(3.71487541375918,-2.26096143585197,4.3));
#18442=CARTESIAN_POINT('Ctrl Pts',(3.70626359340869,-2.25537801909854,4.3));
#18443=CARTESIAN_POINT('Ctrl Pts',(3.69720132775591,-2.25051601191126,4.3));
#18444=CARTESIAN_POINT('Ctrl Pts',(3.6877975535831,-2.24642648892188,4.3));
#18445=CARTESIAN_POINT('Ctrl Pts',(3.67897161991428,-2.24258825780551,4.3));
#18446=CARTESIAN_POINT('Ctrl Pts',(3.66984418789588,-2.23943054868187,4.3));
#18447=CARTESIAN_POINT('Ctrl Pts',(3.66050482692203,-2.23701743659906,4.3));
#18448=CARTESIAN_POINT('Ctrl Pts',(3.65701754284817,-2.23611638915498,4.3));
#18449=CARTESIAN_POINT('Ctrl Pts',(3.65350925028094,-2.23532164136865,4.3));
#18450=CARTESIAN_POINT('Ctrl Pts',(3.64998794572223,-2.2346361398089,4.3));
#18451=CARTESIAN_POINT('Ctrl Pts',(3.63890673460959,-2.23247893148594,4.3));
#18452=CARTESIAN_POINT('Ctrl Pts',(3.62768565700141,-2.23139728883196,4.3));
#18453=CARTESIAN_POINT('Ctrl Pts',(3.61647532022068,-2.23148774583768,4.3));
#18454=CARTESIAN_POINT('Ctrl Pts',(3.61029342610439,-2.23153762798149,4.3));
#18455=CARTESIAN_POINT('Ctrl Pts',(3.60411490309515,-2.23194477515726,4.3));
#18456=CARTESIAN_POINT('Ctrl Pts',(3.59796731355722,-2.23273189751379,4.3));
#18457=CARTESIAN_POINT('Ctrl Pts',(3.59689164899642,-2.23286962297817,4.3));
#18458=CARTESIAN_POINT('Ctrl Pts',(3.59581693782457,-2.2330189937725,4.3));
#18459=CARTESIAN_POINT('Ctrl Pts',(3.5947433329992,-2.23317993884958,4.3));
#18460=CARTESIAN_POINT('Origin',(3.6,-2.4,5.35459252805377));
#18461=CARTESIAN_POINT('Ctrl Pts',(3.39434265963601,-2.39985006386652,5.17959252805377));
#18462=CARTESIAN_POINT('Ctrl Pts',(3.39426084301402,-2.39002096866549,5.17905813053169));
#18463=CARTESIAN_POINT('Ctrl Pts',(3.39937061245186,-2.31213684688635,5.17481913665734));
#18464=CARTESIAN_POINT('Ctrl Pts',(3.49890445172815,-2.1791570162937,5.16687554643073));
#18465=CARTESIAN_POINT('Ctrl Pts',(3.73070050348011,-2.19531101338576,5.15576175737392));
#18466=CARTESIAN_POINT('Ctrl Pts',(3.84286217522106,-2.398786946145,5.14464796831712));
#18467=CARTESIAN_POINT('Ctrl Pts',(3.73273070558319,-2.60338928804541,5.13353417926031));
#18468=CARTESIAN_POINT('Ctrl Pts',(3.50110863577888,-2.62181907448596,5.12242039020351));
#18469=CARTESIAN_POINT('Ctrl Pts',(3.39978420932204,-2.4892623620427,5.11443983980132));
#18470=CARTESIAN_POINT('Ctrl Pts',(3.3942709677865,-2.41067410874191,5.11016388575141));
#18471=CARTESIAN_POINT('Ctrl Pts',(3.39436118987868,-2.40016037422423,5.10959252805377));
#18472=CARTESIAN_POINT('Ctrl Pts',(3.39473290683218,-2.40022967700174,5.18540747194623));
#18473=CARTESIAN_POINT('Ctrl Pts',(3.39508769549541,-2.35320983503088,5.18286245525962));
#18474=CARTESIAN_POINT('Ctrl Pts',(3.4343446160921,-2.23704698664849,5.17661284222074));
#18475=CARTESIAN_POINT('Ctrl Pts',(3.62721323091929,-2.15871475485289,5.16665863282959));
#18476=CARTESIAN_POINT('Ctrl Pts',(3.81747535364037,-2.29190664293025,5.15554484377279));
#18477=CARTESIAN_POINT('Ctrl Pts',(3.80876232171537,-2.52413791100821,5.14443105471598));
#18478=CARTESIAN_POINT('Ctrl Pts',(3.60892556988421,-2.64269428158759,5.13331726565918));
#18479=CARTESIAN_POINT('Ctrl Pts',(3.42787437077081,-2.55254601515802,5.12364273806926));
#18480=CARTESIAN_POINT('Ctrl Pts',(3.39500775643356,-2.44179202298147,5.11767280683161));
#18481=CARTESIAN_POINT('Ctrl Pts',(3.39479089893477,-2.39988380139174,5.11540747194623));
#18482=CARTESIAN_POINT('Ctrl Pts',(3.72690708798524,-2.29206413469515,5.2));
#18483=CARTESIAN_POINT('Ctrl Pts',(3.76279833110066,-2.33426376069605,5.19629540364773));
#18484=CARTESIAN_POINT('Ctrl Pts',(3.78852079223234,-2.45658683270444,5.18888621094319));
#18485=CARTESIAN_POINT('Ctrl Pts',(3.65451255926051,-2.58934148319728,5.1777724218864));
#18486=CARTESIAN_POINT('Ctrl Pts',(3.47057723832131,-2.54835675254144,5.16665863282959));
#18487=CARTESIAN_POINT('Ctrl Pts',(3.40512138630522,-2.37179019391731,5.15554484377279));
#18488=CARTESIAN_POINT('Ctrl Pts',(3.51803130141336,-2.22093957374148,5.14443105471598));
#18489=CARTESIAN_POINT('Ctrl Pts',(3.7059725216196,-2.23403730298123,5.13331726565917));
#18490=CARTESIAN_POINT('Ctrl Pts',(3.79691367996997,-2.39901645079819,5.12220347660237));
#18491=CARTESIAN_POINT('Ctrl Pts',(3.70761861808084,-2.56490889591613,5.11108968754556));
#18492=CARTESIAN_POINT('Ctrl Pts',(3.5198184631744,-2.57985184479553,5.09997589848876));
#18493=CARTESIAN_POINT('Ctrl Pts',(3.40540965360542,-2.43017761320763,5.08886210943196));
#18494=CARTESIAN_POINT('Ctrl Pts',(3.46911145738791,-2.25287984568082,5.07774832037515));
#18495=CARTESIAN_POINT('Ctrl Pts',(3.65261709726835,-2.21024363500907,5.06663453131835));
#18496=CARTESIAN_POINT('Ctrl Pts',(3.7879616770095,-2.34129317212888,5.05552074226154));
#18497=CARTESIAN_POINT('Ctrl Pts',(3.75126281927757,-2.52607793686066,5.04440695320475));
#18498=CARTESIAN_POINT('Ctrl Pts',(3.57611137907248,-2.59546203514889,5.03329316414793));
#18499=CARTESIAN_POINT('Ctrl Pts',(3.42282546878807,-2.4859375664189,5.02217937509114));
#18500=CARTESIAN_POINT('Ctrl Pts',(3.43170941408529,-2.29775344335704,5.01106558603433));
#18501=CARTESIAN_POINT('Ctrl Pts',(3.59463164228021,-2.20315676572473,4.99995179697753));
#18502=CARTESIAN_POINT('Ctrl Pts',(3.76246758864558,-2.28873292649683,4.98883800792072));
#18503=CARTESIAN_POINT('Ctrl Pts',(3.78159510888145,-2.47615310463782,4.97772421886392));
#18504=CARTESIAN_POINT('Ctrl Pts',(3.63450656639691,-2.59386948090233,4.96661042980711));
#18505=CARTESIAN_POINT('Ctrl Pts',(3.45583377242442,-2.53413492344978,4.95549664075031));
#18506=CARTESIAN_POINT('Ctrl Pts',(3.40911796147502,-2.3516251489795,4.94438285169351));
#18507=CARTESIAN_POINT('Ctrl Pts',(3.53711864515359,-2.21339342445149,4.93326906263669));
#18508=CARTESIAN_POINT('Ctrl Pts',(3.7226753460379,-2.24596481468812,4.9221552735799));
#18509=CARTESIAN_POINT('Ctrl Pts',(3.7959459114648,-2.41952635696717,4.91104148452308));
#18510=CARTESIAN_POINT('Ctrl Pts',(3.68986496194813,-2.57521520324594,4.89992769546629));
#18511=CARTESIAN_POINT('Ctrl Pts',(3.50152959362338,-2.57052758693027,4.88881390640948));
#18512=CARTESIAN_POINT('Ctrl Pts',(3.403325304985,-2.4097541363769,4.87770011735268));
#18513=CARTESIAN_POINT('Ctrl Pts',(3.48513959513685,-2.24005261418135,4.86658632829587));
#18514=CARTESIAN_POINT('Ctrl Pts',(3.6720869164654,-2.21675274815082,4.85547253923907));
#18515=CARTESIAN_POINT('Ctrl Pts',(3.79305226563199,-2.36118116990379,4.84435875018227));
#18516=CARTESIAN_POINT('Ctrl Pts',(3.73731468670399,-2.54114090707891,4.83324496112546));
#18517=CARTESIAN_POINT('Ctrl Pts',(3.55589141778138,-2.59191277135814,4.82213117206866));
#18518=CARTESIAN_POINT('Ctrl Pts',(3.41484123438881,-2.46702469957432,4.81101738301185));
#18519=CARTESIAN_POINT('Ctrl Pts',(3.44326896900338,-2.28078816015838,4.79990359395505));
#18520=CARTESIAN_POINT('Ctrl Pts',(3.61515439373994,-2.20366756970366,4.78878980489824));
#18521=CARTESIAN_POINT('Ctrl Pts',(3.77316883002382,-2.3062522792604,4.77767601584144));
#18522=CARTESIAN_POINT('Ctrl Pts',(3.77267987231879,-2.49464534078155,4.76656222678464));
#18523=CARTESIAN_POINT('Ctrl Pts',(3.61413506915742,-2.59640844853418,4.75544843772783));
#18524=CARTESIAN_POINT('Ctrl Pts',(3.44265227689368,-2.51839667592017,4.74433464867102));
#18525=CARTESIAN_POINT('Ctrl Pts',(3.4151916400337,-2.33201508312681,4.73322085961423));
#18526=CARTESIAN_POINT('Ctrl Pts',(3.55688819092022,-2.20786085574886,4.72210707055742));
#18527=CARTESIAN_POINT('Ctrl Pts',(3.73804546957863,-2.25957376611009,4.71099328150061));
#18528=CARTESIAN_POINT('Ctrl Pts',(3.79284816438962,-2.43982040089255,4.69987949244382));
#18529=CARTESIAN_POINT('Ctrl Pts',(3.67113474728785,-2.58361897114401,4.688765703387));
#18530=CARTESIAN_POINT('Ctrl Pts',(3.48431088927061,-2.55934901472658,4.67765191433021));
#18531=CARTESIAN_POINT('Ctrl Pts',(3.40337858630773,-2.38922509798919,4.66653812527339));
#18532=CARTESIAN_POINT('Ctrl Pts',(3.50241609313587,-2.22896357125796,4.6554243362166));
#18533=CARTESIAN_POINT('Ctrl Pts',(3.69077325659353,-2.22525362743943,4.64431054715978));
#18534=CARTESIAN_POINT('Ctrl Pts',(3.79604462885236,-2.38149102018406,4.63319675810299));
#18535=CARTESIAN_POINT('Ctrl Pts',(3.72187412902538,-2.5546698920607,4.62208296904618));
#18536=CARTESIAN_POINT('Ctrl Pts',(3.53615085675469,-2.58627765765756,4.61096917998938));
#18537=CARTESIAN_POINT('Ctrl Pts',(3.40886942939528,-2.44738337066962,4.59985539093257));
#18538=CARTESIAN_POINT('Ctrl Pts',(3.45653198087784,-2.26511854714084,4.58874160187577));
#18539=CARTESIAN_POINT('Ctrl Pts',(3.63551243730216,-2.20631224707971,4.57762781281896));
#18540=CARTESIAN_POINT('Ctrl Pts',(3.78198795712288,-2.32479054382313,4.56651402376216));
#18541=CARTESIAN_POINT('Ctrl Pts',(3.76188783591025,-2.51210890876234,4.55540023470536));
#18542=CARTESIAN_POINT('Ctrl Pts',(3.59360994254596,-2.59681271806211,4.54428644564855));
#18543=CARTESIAN_POINT('Ctrl Pts',(3.43118094125773,-2.50137161460726,4.53317265659175));
#18544=CARTESIAN_POINT('Ctrl Pts',(3.42327393893419,-2.31314392247853,4.52205886753494));
#18545=CARTESIAN_POINT('Ctrl Pts',(3.57712630459504,-2.2044165835037,4.51094507847814));
#18546=CARTESIAN_POINT('Ctrl Pts',(3.75191522290318,-2.2747089629466,4.49983128942133));
#18547=CARTESIAN_POINT('Ctrl Pts',(3.78765441517707,-2.45968165103968,4.48871750036453));
#18548=CARTESIAN_POINT('Ctrl Pts',(3.6516313924431,-2.59002704401991,4.47760371130773));
#18549=CARTESIAN_POINT('Ctrl Pts',(3.46834957196871,-2.54643853472375,4.46648992225092));
#18550=CARTESIAN_POINT('Ctrl Pts',(3.40556887868038,-2.36881316151698,4.45537613319412));
#18551=CARTESIAN_POINT('Ctrl Pts',(3.52075320095807,-2.21973347999151,4.44426234413732));
#18552=CARTESIAN_POINT('Ctrl Pts',(3.70847300665902,-2.23565373905929,4.43314855508051));
#18553=CARTESIAN_POINT('Ctrl Pts',(3.79690626014289,-2.40200209376731,4.4220347660237));
#18554=CARTESIAN_POINT('Ctrl Pts',(3.70510893870568,-2.56651771072077,4.4109209769669));
#18555=CARTESIAN_POINT('Ctrl Pts',(3.51710429764661,-2.57861817635772,4.3998071879101));
#18556=CARTESIAN_POINT('Ctrl Pts',(3.4049748648587,-2.42722660301959,4.3886933988533));
#18557=CARTESIAN_POINT('Ctrl Pts',(3.47135448681048,-2.25091580613535,4.37757960979649));
#18558=CARTESIAN_POINT('Ctrl Pts',(3.65548413146169,-2.21106026869437,4.36646582073969));
#18559=CARTESIAN_POINT('Ctrl Pts',(3.78882987196794,-2.34414980590083,4.35535203168288));
#18560=CARTESIAN_POINT('Ctrl Pts',(3.74933478455633,-2.5283468513898,4.34423824262608));
#18561=CARTESIAN_POINT('Ctrl Pts',(3.57315729153603,-2.59509221614966,4.33312445356927));
#18562=CARTESIAN_POINT('Ctrl Pts',(3.42153838470822,-2.4832160988167,4.32201066451247));
#18563=CARTESIAN_POINT('Ctrl Pts',(3.43328918604681,-2.2952742544727,4.31089687545567));
#18564=CARTESIAN_POINT('Ctrl Pts',(3.59758810222901,-2.20298223652265,4.29978308639886));
#18565=CARTESIAN_POINT('Ctrl Pts',(3.76418972838082,-2.29144636425406,4.28866929734206));
#18566=CARTESIAN_POINT('Ctrl Pts',(3.77483953817107,-2.41599017382994,4.28126010463752));
#18567=CARTESIAN_POINT('Ctrl Pts',(3.75264423560529,-2.46674801372684,4.27755550828525));
#18568=CARTESIAN_POINT('Ctrl Pts',(3.73677806246588,-2.28366876301903,5.20748149723825));
#18569=CARTESIAN_POINT('Ctrl Pts',(3.77546096639785,-2.32915072287504,5.20377690088598));
#18570=CARTESIAN_POINT('Ctrl Pts',(3.80318414917118,-2.46098821950194,5.19636770818144));
#18571=CARTESIAN_POINT('Ctrl Pts',(3.65875260676202,-2.60406867439235,5.18525391912464));
#18572=CARTESIAN_POINT('Ctrl Pts',(3.46051059194224,-2.55989610579284,5.17414013006784));
#18573=CARTESIAN_POINT('Ctrl Pts',(3.38996351094031,-2.36959600381834,5.16302634101104));
#18574=CARTESIAN_POINT('Ctrl Pts',(3.51165568485162,-2.20701205459222,5.15191255195423));
#18575=CARTESIAN_POINT('Ctrl Pts',(3.71421518223977,-2.22112853978274,5.14079876289742));
#18576=CARTESIAN_POINT('Ctrl Pts',(3.81222984505367,-2.39893994924713,5.12968497384063));
#18577=CARTESIAN_POINT('Ctrl Pts',(3.71598931391495,-2.57773569329255,5.11857118478381));
#18578=CARTESIAN_POINT('Ctrl Pts',(3.51358185404256,-2.59384092135901,5.10745739572702));
#18579=CARTESIAN_POINT('Ctrl Pts',(3.3902741999918,-2.43252486153385,5.0963436066702));
#18580=CARTESIAN_POINT('Ctrl Pts',(3.45893080093723,-2.2414366764148,5.08522981761341));
#18581=CARTESIAN_POINT('Ctrl Pts',(3.65670971362751,-2.19548417384656,5.07411602855659));
#18582=CARTESIAN_POINT('Ctrl Pts',(3.80258154534432,-2.33672688974895,5.0630022394998));
#18583=CARTESIAN_POINT('Ctrl Pts',(3.76302820963254,-2.53588441904446,5.05188845044299));
#18584=CARTESIAN_POINT('Ctrl Pts',(3.57425329556196,-2.61066528968353,5.04077466138618));
#18585=CARTESIAN_POINT('Ctrl Pts',(3.40904463665349,-2.49262188593578,5.02966087232938));
#18586=CARTESIAN_POINT('Ctrl Pts',(3.41861958509882,-2.28980059243768,5.01854708327258));
#18587=CARTESIAN_POINT('Ctrl Pts',(3.59421408544476,-2.18784607998553,5.00743329421577));
#18588=CARTESIAN_POINT('Ctrl Pts',(3.77510449842668,-2.28007844974125,4.99631950515897));
#18589=CARTESIAN_POINT('Ctrl Pts',(3.79571977846481,-2.48207637783269,4.98520571610217));
#18590=CARTESIAN_POINT('Ctrl Pts',(3.63719052551791,-2.60894886479604,4.97409192704536));
#18591=CARTESIAN_POINT('Ctrl Pts',(3.4446203628666,-2.54456808701342,4.96297813798855));
#18592=CARTESIAN_POINT('Ctrl Pts',(3.39427094417278,-2.34786249925276,4.95186434893176));
#18593=CARTESIAN_POINT('Ctrl Pts',(3.53222766342159,-2.19887895741578,4.94075055987495));
#18594=CARTESIAN_POINT('Ctrl Pts',(3.73221717092231,-2.23398378661889,4.92963677081814));
#18595=CARTESIAN_POINT('Ctrl Pts',(3.81118680243757,-2.42104513873408,4.91852298176134));
#18596=CARTESIAN_POINT('Ctrl Pts',(3.69685475865827,-2.58884363667168,4.90740919270454));
#18597=CARTESIAN_POINT('Ctrl Pts',(3.4938704558725,-2.58379141234426,4.89629540364773));
#18598=CARTESIAN_POINT('Ctrl Pts',(3.38802772841696,-2.41051282395524,4.88518161459093));
#18599=CARTESIAN_POINT('Ctrl Pts',(3.47620562507071,-2.22761172857971,4.87406782553412));
#18600=CARTESIAN_POINT('Ctrl Pts',(3.67769391702081,-2.20249957304951,4.86295403647733));
#18601=CARTESIAN_POINT('Ctrl Pts',(3.80806808561287,-2.35816179811509,4.85184024742051));
#18602=CARTESIAN_POINT('Ctrl Pts',(3.74799517579086,-2.552119003843,4.84072645836372));
#18603=CARTESIAN_POINT('Ctrl Pts',(3.55246060318804,-2.60683996020677,4.8296126693069));
#18604=CARTESIAN_POINT('Ctrl Pts',(3.40043937962063,-2.4722379552685,4.8184988802501));
#18605=CARTESIAN_POINT('Ctrl Pts',(3.43107825505782,-2.27151573063888,4.8073850911933));
#18606=CARTESIAN_POINT('Ctrl Pts',(3.61633311934347,-2.18839661486619,4.79627130213649));
#18607=CARTESIAN_POINT('Ctrl Pts',(3.78663809426387,-2.29896047725209,4.78515751307969));
#18608=CARTESIAN_POINT('Ctrl Pts',(3.7861111048846,-2.50200696067527,4.77404372402288));
#18609=CARTESIAN_POINT('Ctrl Pts',(3.61523451056097,-2.61168531615476,4.76292993496608));
#18610=CARTESIAN_POINT('Ctrl Pts',(3.43041359594979,-2.52760570108303,4.75181614590928));
#18611=CARTESIAN_POINT('Ctrl Pts',(3.40081704020639,-2.32672714066293,4.74070235685248));
#18612=CARTESIAN_POINT('Ctrl Pts',(3.55353490645048,-2.19291605936479,4.72958856779566));
#18613=CARTESIAN_POINT('Ctrl Pts',(3.74878279977045,-2.24865125742167,4.71847477873887));
#18614=CARTESIAN_POINT('Ctrl Pts',(3.80784810914882,-2.44291767597198,4.70736098968206));
#18615=CARTESIAN_POINT('Ctrl Pts',(3.67666768706539,-2.59790105898559,4.69624720062525));
#18616=CARTESIAN_POINT('Ctrl Pts',(3.47531246154031,-2.57174335835902,4.68513341156846));
#18617=CARTESIAN_POINT('Ctrl Pts',(3.38808515402025,-2.38838701412431,4.67401962251165));
#18618=CARTESIAN_POINT('Ctrl Pts',(3.49482590830325,-2.21566016756178,4.66290583345484));
#18619=CARTESIAN_POINT('Ctrl Pts',(3.69783370147164,-2.21166166018595,4.65179204439804));
#18620=CARTESIAN_POINT('Ctrl Pts',(3.81129319817336,-2.38005137114376,4.64067825534124));
#18621=CARTESIAN_POINT('Ctrl Pts',(3.73135363435924,-2.56670028832692,4.62956446628443));
#18622=CARTESIAN_POINT('Ctrl Pts',(3.53118459936441,-2.60076654109381,4.61845067722763));
#18623=CARTESIAN_POINT('Ctrl Pts',(3.3940030809914,-2.45106890195169,4.60733688817082));
#18624=CARTESIAN_POINT('Ctrl Pts',(3.44537287875023,-2.25462731768926,4.59622309911402));
#18625=CARTESIAN_POINT('Ctrl Pts',(3.63827463418116,-2.1912469981906,4.58510931005721));
#18626=CARTESIAN_POINT('Ctrl Pts',(3.79614318287948,-2.31894066865531,4.57399552100041));
#18627=CARTESIAN_POINT('Ctrl Pts',(3.77447965187866,-2.52082886440086,4.56288173194361));
#18628=CARTESIAN_POINT('Ctrl Pts',(3.59311291676859,-2.6121210302163,4.55176794288681));
#18629=CARTESIAN_POINT('Ctrl Pts',(3.41805000706685,-2.50925641156176,4.54065415383));
#18630=CARTESIAN_POINT('Ctrl Pts',(3.40952798930647,-2.3063881601463,4.52954036477319));
#18631=CARTESIAN_POINT('Ctrl Pts',(3.57534716312072,-2.18920388779283,4.51842657571639));
#18632=CARTESIAN_POINT('Ctrl Pts',(3.76373135793792,-2.26496368670519,4.50731278665958));
#18633=CARTESIAN_POINT('Ctrl Pts',(3.80225038434475,-2.46432375625011,4.49619899760278));
#18634=CARTESIAN_POINT('Ctrl Pts',(3.65564733958441,-2.60480755889841,4.48508520854597));
#18635=CARTESIAN_POINT('Ctrl Pts',(3.45810965522258,-2.55782868685937,4.47397141948917));
#18636=CARTESIAN_POINT('Ctrl Pts',(3.39044580977021,-2.36638741452612,4.46285763043237));
#18637=CARTESIAN_POINT('Ctrl Pts',(3.51458929677089,-2.20571214952866,4.45174384137556));
#18638=CARTESIAN_POINT('Ctrl Pts',(3.71691015778721,-2.22287070405714,4.44063005231876));
#18639=CARTESIAN_POINT('Ctrl Pts',(3.81222184810419,-2.40215781884775,4.42951626326195));
#18640=CARTESIAN_POINT('Ctrl Pts',(3.71328442888611,-2.57946964350242,4.41840247420515));
#18641=CARTESIAN_POINT('Ctrl Pts',(3.51065657770066,-2.59251129681771,4.40728868514835));
#18642=CARTESIAN_POINT('Ctrl Pts',(3.38980559289267,-2.42934431849055,4.39617489609154));
#18643=CARTESIAN_POINT('Ctrl Pts',(3.46134829568354,-2.23931987168859,4.38506110703474));
#18644=CARTESIAN_POINT('Ctrl Pts',(3.65979974892982,-2.19636432620836,4.37394731797793));
#18645=CARTESIAN_POINT('Ctrl Pts',(3.80351726947246,-2.33980571567353,4.36283352892113));
#18646=CARTESIAN_POINT('Ctrl Pts',(3.76095021022585,-2.5383298122697,4.35171973986433));
#18647=CARTESIAN_POINT('Ctrl Pts',(3.57106943581066,-2.61026670575114,4.34060595080752));
#18648=CARTESIAN_POINT('Ctrl Pts',(3.4076574417421,-2.48968873955599,4.32949216175071));
#18649=CARTESIAN_POINT('Ctrl Pts',(3.42032223348093,-2.28712856948396,4.31837837269392));
#18650=CARTESIAN_POINT('Ctrl Pts',(3.59740050213728,-2.18765797570795,4.30726458363711));
#18651=CARTESIAN_POINT('Ctrl Pts',(3.77696058810632,-2.28300294170579,4.29615079458031));
#18652=CARTESIAN_POINT('Ctrl Pts',(3.78843875194939,-2.41723390733862,4.28874160187577));
#18653=CARTESIAN_POINT('Ctrl Pts',(3.76451707405898,-2.471939748488,4.2850370055235));
#18654=CARTESIAN_POINT('Ctrl Pts',(3.74664903694653,-2.2752733913429,5.2149629944765));
#18655=CARTESIAN_POINT('Ctrl Pts',(3.78812360169505,-2.32403768505403,5.21125839812423));
#18656=CARTESIAN_POINT('Ctrl Pts',(3.81784750611002,-2.46538960629943,5.20384920541969));
#18657=CARTESIAN_POINT('Ctrl Pts',(3.66299265426352,-2.61879586558741,5.19273541636289));
#18658=CARTESIAN_POINT('Ctrl Pts',(3.45044394556317,-2.57143545904423,5.18162162730609));
#18659=CARTESIAN_POINT('Ctrl Pts',(3.37480563557539,-2.36740181371937,5.17050783824928));
#18660=CARTESIAN_POINT('Ctrl Pts',(3.50528006828989,-2.19308453544296,5.15939404919248));
#18661=CARTESIAN_POINT('Ctrl Pts',(3.72245784285994,-2.20821977658425,5.14828026013567));
#18662=CARTESIAN_POINT('Ctrl Pts',(3.82754601013736,-2.39886344769606,5.13716647107887));
#18663=CARTESIAN_POINT('Ctrl Pts',(3.72436000974907,-2.59056249066898,5.12605268202206));
#18664=CARTESIAN_POINT('Ctrl Pts',(3.50734524491072,-2.60782999792249,5.11493889296526));
#18665=CARTESIAN_POINT('Ctrl Pts',(3.37513874637818,-2.43487210986008,5.10382510390845));
#18666=CARTESIAN_POINT('Ctrl Pts',(3.44875014448657,-2.22999350714877,5.09271131485166));
#18667=CARTESIAN_POINT('Ctrl Pts',(3.66080232998667,-2.18072471268405,5.08159752579485));
#18668=CARTESIAN_POINT('Ctrl Pts',(3.81720141367915,-2.33216060736901,5.07048373673804));
#18669=CARTESIAN_POINT('Ctrl Pts',(3.77479359998752,-2.54569090122825,5.05936994768124));
#18670=CARTESIAN_POINT('Ctrl Pts',(3.57239521205144,-2.62586854421817,5.04825615862443));
#18671=CARTESIAN_POINT('Ctrl Pts',(3.39526380451891,-2.49930620545266,5.03714236956763));
#18672=CARTESIAN_POINT('Ctrl Pts',(3.40552975611236,-2.28184774151832,5.02602858051083));
#18673=CARTESIAN_POINT('Ctrl Pts',(3.59379652860931,-2.17253539424633,5.01491479145402));
#18674=CARTESIAN_POINT('Ctrl Pts',(3.78774140820779,-2.27142397298568,5.00380100239722));
#18675=CARTESIAN_POINT('Ctrl Pts',(3.80984444804818,-2.48799965102756,4.99268721334042));
#18676=CARTESIAN_POINT('Ctrl Pts',(3.63987448463892,-2.62402824868975,4.98157342428361));
#18677=CARTESIAN_POINT('Ctrl Pts',(3.43340695330878,-2.55500125057707,4.9704596352268));
#18678=CARTESIAN_POINT('Ctrl Pts',(3.37942392687054,-2.34409984952602,4.95934584617001));
#18679=CARTESIAN_POINT('Ctrl Pts',(3.52733668168959,-2.18436449038006,4.94823205711319));
#18680=CARTESIAN_POINT('Ctrl Pts',(3.74175899580671,-2.22200275854966,4.9371182680564));
#18681=CARTESIAN_POINT('Ctrl Pts',(3.82642769341035,-2.42256392050098,4.92600447899958));
#18682=CARTESIAN_POINT('Ctrl Pts',(3.70384455536842,-2.60247207009742,4.91489068994279));
#18683=CARTESIAN_POINT('Ctrl Pts',(3.48621131812161,-2.59705523775825,4.90377690088598));
#18684=CARTESIAN_POINT('Ctrl Pts',(3.37273015184892,-2.41127151153357,4.89266311182918));
#18685=CARTESIAN_POINT('Ctrl Pts',(3.46727165500458,-2.21517084297807,4.88154932277238));
#18686=CARTESIAN_POINT('Ctrl Pts',(3.68330091757622,-2.1882463979482,4.87043553371556));
#18687=CARTESIAN_POINT('Ctrl Pts',(3.82308390559375,-2.3551424263264,4.85932174465877));
#18688=CARTESIAN_POINT('Ctrl Pts',(3.75867566487773,-2.56309710060709,4.84820795560196));
#18689=CARTESIAN_POINT('Ctrl Pts',(3.54902978859471,-2.62176714905541,4.83709416654515));
#18690=CARTESIAN_POINT('Ctrl Pts',(3.38603752485245,-2.47745121096268,4.82598037748835));
#18691=CARTESIAN_POINT('Ctrl Pts',(3.41888754111225,-2.26224330111939,4.81486658843154));
#18692=CARTESIAN_POINT('Ctrl Pts',(3.61751184494699,-2.17312566002871,4.80375279937474));
#18693=CARTESIAN_POINT('Ctrl Pts',(3.80010735850391,-2.29166867524379,4.79263901031795));
#18694=CARTESIAN_POINT('Ctrl Pts',(3.79954233745042,-2.50936858056899,4.78152522126113));
#18695=CARTESIAN_POINT('Ctrl Pts',(3.61633395196453,-2.62696218377534,4.77041143220433));
#18696=CARTESIAN_POINT('Ctrl Pts',(3.4181749150059,-2.53681472624589,4.75929764314752));
#18697=CARTESIAN_POINT('Ctrl Pts',(3.38644244037908,-2.32143919819905,4.74818385409072));
#18698=CARTESIAN_POINT('Ctrl Pts',(3.55018162198074,-2.1779712629807,4.73707006503392));
#18699=CARTESIAN_POINT('Ctrl Pts',(3.75952012996226,-2.23772874873326,4.72595627597711));
#18700=CARTESIAN_POINT('Ctrl Pts',(3.82284805390801,-2.44601495105141,4.71484248692031));
#18701=CARTESIAN_POINT('Ctrl Pts',(3.68220062684293,-2.61218314682717,4.7037286978635));
#18702=CARTESIAN_POINT('Ctrl Pts',(3.46631403381001,-2.58413770199147,4.69261490880671));
#18703=CARTESIAN_POINT('Ctrl Pts',(3.37279172173275,-2.38754893025942,4.68150111974989));
#18704=CARTESIAN_POINT('Ctrl Pts',(3.48723572347063,-2.20235676386561,4.6703873306931));
#18705=CARTESIAN_POINT('Ctrl Pts',(3.70489414634973,-2.19806969293246,4.65927354163628));
#18706=CARTESIAN_POINT('Ctrl Pts',(3.82654176749436,-2.37861172210345,4.64815975257949));
#18707=CARTESIAN_POINT('Ctrl Pts',(3.7408331396931,-2.57873068459315,4.63704596352267));
#18708=CARTESIAN_POINT('Ctrl Pts',(3.52621834197413,-2.61525542453006,4.62593217446588));
#18709=CARTESIAN_POINT('Ctrl Pts',(3.37913673258752,-2.45475443323377,4.61481838540907));
#18710=CARTESIAN_POINT('Ctrl Pts',(3.43421377662264,-2.24413608823767,4.60370459635227));
#18711=CARTESIAN_POINT('Ctrl Pts',(3.64103683106015,-2.17618174930149,4.59259080729546));
#18712=CARTESIAN_POINT('Ctrl Pts',(3.81029840863609,-2.31309079348749,4.58147701823866));
#18713=CARTESIAN_POINT('Ctrl Pts',(3.78707146784707,-2.52954882003939,4.57036322918186));
#18714=CARTESIAN_POINT('Ctrl Pts',(3.59261589099123,-2.62742934237049,4.55924944012505));
#18715=CARTESIAN_POINT('Ctrl Pts',(3.40491907287596,-2.51714120851626,4.54813565106824));
#18716=CARTESIAN_POINT('Ctrl Pts',(3.39578203967876,-2.29963239781408,4.53702186201144));
#18717=CARTESIAN_POINT('Ctrl Pts',(3.57356802164639,-2.17399119208196,4.52590807295464));
#18718=CARTESIAN_POINT('Ctrl Pts',(3.77554749297266,-2.2552184104638,4.51479428389784));
#18719=CARTESIAN_POINT('Ctrl Pts',(3.81684635351243,-2.46896586146052,4.50368049484103));
#18720=CARTESIAN_POINT('Ctrl Pts',(3.65966328672572,-2.61958807377691,4.49256670578423));
#18721=CARTESIAN_POINT('Ctrl Pts',(3.44786973847645,-2.56921883899499,4.48145291672742));
#18722=CARTESIAN_POINT('Ctrl Pts',(3.37532274086005,-2.36396166753528,4.47033912767061));
#18723=CARTESIAN_POINT('Ctrl Pts',(3.5084253925837,-2.19169081906581,4.45922533861382));
#18724=CARTESIAN_POINT('Ctrl Pts',(3.7253473089154,-2.21008766905501,4.44811154955701));
#18725=CARTESIAN_POINT('Ctrl Pts',(3.82753743606548,-2.40231354392819,4.43699776050021));
#18726=CARTESIAN_POINT('Ctrl Pts',(3.72145991906655,-2.59242157628407,4.4258839714434));
#18727=CARTESIAN_POINT('Ctrl Pts',(3.5042088577547,-2.60640441727771,4.41477018238659));
#18728=CARTESIAN_POINT('Ctrl Pts',(3.37463632092665,-2.43146203396151,4.4036563933298));
#18729=CARTESIAN_POINT('Ctrl Pts',(3.45134210455661,-2.22772393724184,4.39254260427299));
#18730=CARTESIAN_POINT('Ctrl Pts',(3.66411536639796,-2.18166838372235,4.38142881521618));
#18731=CARTESIAN_POINT('Ctrl Pts',(3.81820466697696,-2.33546162544623,4.37031502615938));
#18732=CARTESIAN_POINT('Ctrl Pts',(3.77256563589538,-2.54831277314961,4.35920123710258));
#18733=CARTESIAN_POINT('Ctrl Pts',(3.5689815800853,-2.62544119535262,4.34808744804577));
#18734=CARTESIAN_POINT('Ctrl Pts',(3.39377649877598,-2.49616138029528,4.33697365898897));
#18735=CARTESIAN_POINT('Ctrl Pts',(3.40735528091504,-2.27898288449522,4.32585986993216));
#18736=CARTESIAN_POINT('Ctrl Pts',(3.59721290204555,-2.17233371489326,4.31474608087536));
#18737=CARTESIAN_POINT('Ctrl Pts',(3.78973144783182,-2.27455951915752,4.30363229181856));
#18738=CARTESIAN_POINT('Ctrl Pts',(3.8020379657277,-2.4184776408473,4.29622309911402));
#18739=CARTESIAN_POINT('Ctrl Pts',(3.77638991251267,-2.47713148324917,4.29251850276175));
#18740=CARTESIAN_POINT('Ctrl Pts',(3.75652001142717,-2.26687801966678,5.22244449171475));
#18741=CARTESIAN_POINT('Ctrl Pts',(3.80078623699225,-2.31892464723302,5.21873989536248));
#18742=CARTESIAN_POINT('Ctrl Pts',(3.83251086304886,-2.46979099309691,5.21133070265794));
#18743=CARTESIAN_POINT('Ctrl Pts',(3.66723270176503,-2.63352305678248,5.20021691360114));
#18744=CARTESIAN_POINT('Ctrl Pts',(3.4403772991841,-2.58297481229563,5.18910312454433));
#18745=CARTESIAN_POINT('Ctrl Pts',(3.35964776021048,-2.3652076236204,5.17798933548753));
#18746=CARTESIAN_POINT('Ctrl Pts',(3.49890445172815,-2.1791570162937,5.16687554643073));
#18747=CARTESIAN_POINT('Ctrl Pts',(3.73070050348011,-2.19531101338576,5.15576175737392));
#18748=CARTESIAN_POINT('Ctrl Pts',(3.84286217522106,-2.398786946145,5.14464796831712));
#18749=CARTESIAN_POINT('Ctrl Pts',(3.73273070558319,-2.60338928804541,5.13353417926031));
#18750=CARTESIAN_POINT('Ctrl Pts',(3.50110863577888,-2.62181907448596,5.12242039020351));
#18751=CARTESIAN_POINT('Ctrl Pts',(3.36000329276455,-2.4372193581863,5.1113066011467));
#18752=CARTESIAN_POINT('Ctrl Pts',(3.4385694880359,-2.21855033788275,5.10019281208991));
#18753=CARTESIAN_POINT('Ctrl Pts',(3.66489494634582,-2.16596525152154,5.08907902303309));
#18754=CARTESIAN_POINT('Ctrl Pts',(3.83182128201397,-2.32759432498908,5.07796523397629));
#18755=CARTESIAN_POINT('Ctrl Pts',(3.78655899034249,-2.55549738341204,5.06685144491949));
#18756=CARTESIAN_POINT('Ctrl Pts',(3.57053712854092,-2.64107179875281,5.05573765586268));
#18757=CARTESIAN_POINT('Ctrl Pts',(3.38148297238433,-2.50599052496954,5.04462386680588));
#18758=CARTESIAN_POINT('Ctrl Pts',(3.3924399271259,-2.27389489059897,5.03351007774908));
#18759=CARTESIAN_POINT('Ctrl Pts',(3.59337897177386,-2.15722470850713,5.02239628869227));
#18760=CARTESIAN_POINT('Ctrl Pts',(3.8003783179889,-2.26276949623011,5.01128249963547));
#18761=CARTESIAN_POINT('Ctrl Pts',(3.82396911763155,-2.49392292422242,5.00016871057867));
#18762=CARTESIAN_POINT('Ctrl Pts',(3.64255844375993,-2.63910763258347,4.98905492152186));
#18763=CARTESIAN_POINT('Ctrl Pts',(3.42219354375095,-2.56543441414071,4.97794113246505));
#18764=CARTESIAN_POINT('Ctrl Pts',(3.3645769095683,-2.34033719979929,4.96682734340826));
#18765=CARTESIAN_POINT('Ctrl Pts',(3.52244569995759,-2.16985002334435,4.95571355435144));
#18766=CARTESIAN_POINT('Ctrl Pts',(3.75130082069111,-2.21002173048044,4.94459976529465));
#18767=CARTESIAN_POINT('Ctrl Pts',(3.84166858438312,-2.42408270226789,4.93348597623783));
#18768=CARTESIAN_POINT('Ctrl Pts',(3.71083435207858,-2.61610050352316,4.92237218718104));
#18769=CARTESIAN_POINT('Ctrl Pts',(3.47855218037073,-2.61031906317225,4.91125839812423));
#18770=CARTESIAN_POINT('Ctrl Pts',(3.35743257528088,-2.4120301991119,4.90014460906743));
#18771=CARTESIAN_POINT('Ctrl Pts',(3.45833768493844,-2.20272995737643,4.88903082001062));
#18772=CARTESIAN_POINT('Ctrl Pts',(3.68890791813162,-2.17399322284688,4.87791703095382));
#18773=CARTESIAN_POINT('Ctrl Pts',(3.83809972557463,-2.3521230545377,4.86680324189701));
#18774=CARTESIAN_POINT('Ctrl Pts',(3.76935615396461,-2.57407519737118,4.85568945284021));
#18775=CARTESIAN_POINT('Ctrl Pts',(3.54559897400137,-2.63669433790405,4.8445756637834));
#18776=CARTESIAN_POINT('Ctrl Pts',(3.37163567008428,-2.48266446665686,4.8334618747266));
#18777=CARTESIAN_POINT('Ctrl Pts',(3.40669682716669,-2.25297087159989,4.8223480856698));
#18778=CARTESIAN_POINT('Ctrl Pts',(3.61869057055051,-2.15785470519124,4.81123429661299));
#18779=CARTESIAN_POINT('Ctrl Pts',(3.81357662274397,-2.28437687323548,4.80012050755619));
#18780=CARTESIAN_POINT('Ctrl Pts',(3.81297357001622,-2.51673020046272,4.78900671849938));
#18781=CARTESIAN_POINT('Ctrl Pts',(3.61743339336808,-2.64223905139592,4.77789292944258));
#18782=CARTESIAN_POINT('Ctrl Pts',(3.405936234062,-2.54602375140875,4.76677914038577));
#18783=CARTESIAN_POINT('Ctrl Pts',(3.37206784055177,-2.31615125573517,4.75566535132898));
#18784=CARTESIAN_POINT('Ctrl Pts',(3.546828337511,-2.16302646659663,4.74455156227216));
#18785=CARTESIAN_POINT('Ctrl Pts',(3.77025746015408,-2.22680624004484,4.73343777321537));
#18786=CARTESIAN_POINT('Ctrl Pts',(3.83784799866721,-2.44911222613084,4.72232398415856));
#18787=CARTESIAN_POINT('Ctrl Pts',(3.68773356662048,-2.62646523466876,4.71121019510175));
#18788=CARTESIAN_POINT('Ctrl Pts',(3.4573156060797,-2.59653204562391,4.70009640604496));
#18789=CARTESIAN_POINT('Ctrl Pts',(3.35749828944527,-2.38671084639454,4.68898261698814));
#18790=CARTESIAN_POINT('Ctrl Pts',(3.47964553863801,-2.18905336016944,4.67786882793135));
#18791=CARTESIAN_POINT('Ctrl Pts',(3.71195459122784,-2.18447772567898,4.66675503887453));
#18792=CARTESIAN_POINT('Ctrl Pts',(3.84179033681535,-2.37717207306315,4.65564124981774));
#18793=CARTESIAN_POINT('Ctrl Pts',(3.75031264502696,-2.59076108085938,4.64452746076093));
#18794=CARTESIAN_POINT('Ctrl Pts',(3.52125208458385,-2.6297443079663,4.63341367170413));
#18795=CARTESIAN_POINT('Ctrl Pts',(3.36427038418365,-2.45843996451585,4.62229988264732));
#18796=CARTESIAN_POINT('Ctrl Pts',(3.42305467449503,-2.23364485878609,4.61118609359052));
#18797=CARTESIAN_POINT('Ctrl Pts',(3.64379902793915,-2.16111650041238,4.60007230453371));
#18798=CARTESIAN_POINT('Ctrl Pts',(3.82445363439269,-2.30724091831967,4.58895851547691));
#18799=CARTESIAN_POINT('Ctrl Pts',(3.79966328381548,-2.53826877567792,4.57784472642011));
#18800=CARTESIAN_POINT('Ctrl Pts',(3.59211886521387,-2.64273765452468,4.5667309373633));
#18801=CARTESIAN_POINT('Ctrl Pts',(3.39178813868507,-2.52502600547076,4.5556171483065));
#18802=CARTESIAN_POINT('Ctrl Pts',(3.38203609005104,-2.29287663548185,4.54450335924969));
#18803=CARTESIAN_POINT('Ctrl Pts',(3.57178888017207,-2.15877849637109,4.53338957019289));
#18804=CARTESIAN_POINT('Ctrl Pts',(3.78736362800739,-2.2454731342224,4.52227578113608));
#18805=CARTESIAN_POINT('Ctrl Pts',(3.83144232268012,-2.47360796667095,4.51116199207928));
#18806=CARTESIAN_POINT('Ctrl Pts',(3.66367923386702,-2.6343685886554,4.50004820302247));
#18807=CARTESIAN_POINT('Ctrl Pts',(3.43762982173032,-2.58060899113062,4.48893441396567));
#18808=CARTESIAN_POINT('Ctrl Pts',(3.36019967194989,-2.36153592054442,4.47782062490886));
#18809=CARTESIAN_POINT('Ctrl Pts',(3.50226148839652,-2.17766948860297,4.46670683585206));
#18810=CARTESIAN_POINT('Ctrl Pts',(3.73378446004359,-2.19730463405286,4.45559304679526));
#18811=CARTESIAN_POINT('Ctrl Pts',(3.84285302402677,-2.40246926900864,4.44447925773845));
#18812=CARTESIAN_POINT('Ctrl Pts',(3.72963540924699,-2.60537350906572,4.43336546868165));
#18813=CARTESIAN_POINT('Ctrl Pts',(3.49776113780875,-2.62029753773771,4.42225167962485));
#18814=CARTESIAN_POINT('Ctrl Pts',(3.35946704896063,-2.43357974943247,4.41113789056804));
#18815=CARTESIAN_POINT('Ctrl Pts',(3.44133591342967,-2.21612800279508,4.40002410151124));
#18816=CARTESIAN_POINT('Ctrl Pts',(3.66843098386609,-2.16697244123634,4.38891031245443));
#18817=CARTESIAN_POINT('Ctrl Pts',(3.83289206448147,-2.33111753521892,4.37779652339763));
#18818=CARTESIAN_POINT('Ctrl Pts',(3.7841810615649,-2.55829573402952,4.36668273434082));
#18819=CARTESIAN_POINT('Ctrl Pts',(3.56689372435994,-2.6406156849541,4.35556894528403));
#18820=CARTESIAN_POINT('Ctrl Pts',(3.37989555580985,-2.50263402103458,4.34445515622721));
#18821=CARTESIAN_POINT('Ctrl Pts',(3.39438832834916,-2.27083719950648,4.33334136717041));
#18822=CARTESIAN_POINT('Ctrl Pts',(3.59702530195382,-2.15700945407857,4.32222757811361));
#18823=CARTESIAN_POINT('Ctrl Pts',(3.80250230755732,-2.26611609660926,4.31111378905681));
#18824=CARTESIAN_POINT('Ctrl Pts',(3.81563717950601,-2.41972137435598,4.30370459635227));
#18825=CARTESIAN_POINT('Ctrl Pts',(3.78826275096636,-2.48232321801033,4.3));
#18826=CARTESIAN_POINT('Ctrl Pts',(3.72690708798524,-2.29206413469515,5.2));
#18827=CARTESIAN_POINT('Ctrl Pts',(3.73511889692415,-2.29972488088976,5.2));
#18828=CARTESIAN_POINT('Ctrl Pts',(3.74243606331987,-2.3082260358574,5.2));
#18829=CARTESIAN_POINT('Ctrl Pts',(3.74885415883116,-2.3173733937361,5.2));
#18830=CARTESIAN_POINT('Ctrl Pts',(3.75362492547366,-2.32417290455016,5.2));
#18831=CARTESIAN_POINT('Ctrl Pts',(3.75789857922842,-2.33133076203089,5.2));
#18832=CARTESIAN_POINT('Ctrl Pts',(3.7616631192462,-2.3387816278666,5.2));
#18833=CARTESIAN_POINT('Ctrl Pts',(3.76388041855661,-2.34317015863036,5.2));
#18834=CARTESIAN_POINT('Ctrl Pts',(3.76592248852987,-2.34766555277529,5.2));
#18835=CARTESIAN_POINT('Ctrl Pts',(3.76777441807103,-2.35222602465318,5.2));
#18836=CARTESIAN_POINT('Ctrl Pts',(3.77233274722043,-2.36345114495818,5.2));
#18837=CARTESIAN_POINT('Ctrl Pts',(3.77575806540191,-2.37509440908006,5.2));
#18838=CARTESIAN_POINT('Ctrl Pts',(3.77802228391775,-2.38695732035888,5.2));
#18839=CARTESIAN_POINT('Ctrl Pts',(3.77946116292117,-2.39449603353478,5.2));
#18840=CARTESIAN_POINT('Ctrl Pts',(3.78043041033378,-2.40212433051409,5.2));
#18841=CARTESIAN_POINT('Ctrl Pts',(3.78091325285907,-2.40979638894873,5.2));
#18842=CARTESIAN_POINT('Ctrl Pts',(3.78113857897669,-2.41337667662164,5.2));
#18843=CARTESIAN_POINT('Ctrl Pts',(3.78125743502661,-2.41696304534708,5.2));
#18844=CARTESIAN_POINT('Ctrl Pts',(3.78126867486757,-2.42054069500775,5.2));
#18845=CARTESIAN_POINT('Ctrl Pts',(3.78130372190818,-2.4316961938677,5.2));
#18846=CARTESIAN_POINT('Ctrl Pts',(3.78029682789473,-2.44279407568189,5.2));
#18847=CARTESIAN_POINT('Ctrl Pts',(3.77821427386403,-2.45369318996624,5.2));
#18848=CARTESIAN_POINT('Ctrl Pts',(3.77705389172366,-2.45976608765585,5.2));
#18849=CARTESIAN_POINT('Ctrl Pts',(3.77555901526444,-2.46577751393184,5.2));
#18850=CARTESIAN_POINT('Ctrl Pts',(3.77374837416276,-2.47171132791926,5.2));
#18851=CARTESIAN_POINT('Ctrl Pts',(3.77261573055045,-2.47542321566067,5.2));
#18852=CARTESIAN_POINT('Ctrl Pts',(3.77135887218697,-2.47910625090944,5.2));
#18853=CARTESIAN_POINT('Ctrl Pts',(3.76998349987259,-2.48275161867489,5.2));
#18854=CARTESIAN_POINT('Ctrl Pts',(3.76560171320323,-2.49436536406777,5.2));
#18855=CARTESIAN_POINT('Ctrl Pts',(3.76005261276,-2.50551619028979,5.2));
#18856=CARTESIAN_POINT('Ctrl Pts',(3.75350161664164,-2.51608155564839,5.2));
#18857=CARTESIAN_POINT('Ctrl Pts',(3.74916064083137,-2.52308262764107,5.2));
#18858=CARTESIAN_POINT('Ctrl Pts',(3.7443785440277,-2.5298267716061,5.2));
#18859=CARTESIAN_POINT('Ctrl Pts',(3.73919190918146,-2.53627611456138,5.2));
#18860=CARTESIAN_POINT('Ctrl Pts',(3.73648178297727,-2.53964603241007,5.2));
#18861=CARTESIAN_POINT('Ctrl Pts',(3.73365980796544,-2.54293677988309,5.2));
#18862=CARTESIAN_POINT('Ctrl Pts',(3.73073436285314,-2.54613815029323,5.2));
#18863=CARTESIAN_POINT('Ctrl Pts',(3.72446793550896,-2.55299562131278,5.2));
#18864=CARTESIAN_POINT('Ctrl Pts',(3.71775196798206,-2.55941733778444,5.2));
#18865=CARTESIAN_POINT('Ctrl Pts',(3.71064054370859,-2.56535254658103,5.2));
#18866=CARTESIAN_POINT('Ctrl Pts',(3.70611395375814,-2.56913044752735,5.2));
#18867=CARTESIAN_POINT('Ctrl Pts',(3.70142688925274,-2.57271116046832,5.2));
#18868=CARTESIAN_POINT('Ctrl Pts',(3.69659110235036,-2.57608017868915,5.2));
#18869=CARTESIAN_POINT('Ctrl Pts',(3.69251867261816,-2.57891737773199,5.2));
#18870=CARTESIAN_POINT('Ctrl Pts',(3.68834776817108,-2.58159940125718,5.2));
#18871=CARTESIAN_POINT('Ctrl Pts',(3.68408920348942,-2.58411662981112,5.2));
#18872=CARTESIAN_POINT('Ctrl Pts',(3.67536613625436,-2.58927281635833,5.2));
#18873=CARTESIAN_POINT('Ctrl Pts',(3.6662720325658,-2.59374119323572,5.2));
#18874=CARTESIAN_POINT('Ctrl Pts',(3.65686566045376,-2.59744798255001,5.2));
#18875=CARTESIAN_POINT('Ctrl Pts',(3.6556263522049,-2.59793635942042,5.2));
#18876=CARTESIAN_POINT('Ctrl Pts',(3.65438160822106,-2.59841149615413,5.2));
#18877=CARTESIAN_POINT('Ctrl Pts',(3.65313161981588,-2.59887345085171,5.2));
#18878=CARTESIAN_POINT('Ctrl Pts',(3.43326718206005,-2.40013003210005,5.08714803633902));
#18879=CARTESIAN_POINT('Ctrl Pts',(3.4331940296057,-2.4086546125631,5.08771939403667));
#18880=CARTESIAN_POINT('Ctrl Pts',(3.43379133726061,-2.41716890764345,5.08829075173431));
#18881=CARTESIAN_POINT('Ctrl Pts',(3.43509475583067,-2.42557369055115,5.08886210943196));
#18882=CARTESIAN_POINT('Ctrl Pts',(3.44354592346175,-2.48006902373693,5.09256670578423));
#18883=CARTESIAN_POINT('Ctrl Pts',(3.48168219331808,-2.52996043426623,5.0962713021365));
#18884=CARTESIAN_POINT('Ctrl Pts',(3.53205035406398,-2.55241564805098,5.09997589848876));
#18885=CARTESIAN_POINT('Ctrl Pts',(3.58241851480988,-2.57487086183573,5.10368049484103));
#18886=CARTESIAN_POINT('Ctrl Pts',(3.64501856644536,-2.56988987887593,5.1073850911933));
#18887=CARTESIAN_POINT('Ctrl Pts',(3.69120110257795,-2.53975064654304,5.11108968754557));
#18888=CARTESIAN_POINT('Ctrl Pts',(3.73738363871054,-2.50961141421015,5.11479428389783));
#18889=CARTESIAN_POINT('Ctrl Pts',(3.76714865934026,-2.45431393250417,5.1184988802501));
#18890=CARTESIAN_POINT('Ctrl Pts',(3.76687430993005,-2.39916866701502,5.12220347660237));
#18891=CARTESIAN_POINT('Ctrl Pts',(3.76659996051984,-2.34402340152587,5.12590807295464));
#18892=CARTESIAN_POINT('Ctrl Pts',(3.73628624106972,-2.28903035225355,5.12961266930691));
#18893=CARTESIAN_POINT('Ctrl Pts',(3.68980584464362,-2.2593508727441,5.13331726565917));
#18894=CARTESIAN_POINT('Ctrl Pts',(3.64332544821752,-2.22967139323465,5.13702186201144));
#18895=CARTESIAN_POINT('Ctrl Pts',(3.58067837481544,-2.22530548348806,5.14072645836371));
#18896=CARTESIAN_POINT('Ctrl Pts',(3.53053651892971,-2.24826429864408,5.14443105471598));
#18897=CARTESIAN_POINT('Ctrl Pts',(3.48039466304398,-2.27122311380009,5.14813565106825));
#18898=CARTESIAN_POINT('Ctrl Pts',(3.4427580246746,-2.3215066538587,5.15184024742052));
#18899=CARTESIAN_POINT('Ctrl Pts',(3.43484901415926,-2.37607618365869,5.15554484377278));
#18900=CARTESIAN_POINT('Ctrl Pts',(3.4337081191144,-2.3839479782439,5.15607924129486));
#18901=CARTESIAN_POINT('Ctrl Pts',(3.43318582039731,-2.39190895914184,5.15661363881694));
#18902=CARTESIAN_POINT('Ctrl Pts',(3.43325215766083,-2.39987843114813,5.15714803633902));
#18903=CARTESIAN_POINT('Ctrl Pts',(3.54698297828114,-2.59851743256717,5.2));
#18904=CARTESIAN_POINT('Ctrl Pts',(3.48097120902544,-2.58088801151799,5.19629540364773));
#18905=CARTESIAN_POINT('Ctrl Pts',(3.36906717021742,-2.4748477879482,5.1888862109432));
#18906=CARTESIAN_POINT('Ctrl Pts',(3.41187708350278,-2.24617201703375,5.17777242188639));
#18907=CARTESIAN_POINT('Ctrl Pts',(3.62721323091929,-2.15871475485289,5.16665863282959));
#18908=CARTESIAN_POINT('Ctrl Pts',(3.81747535364037,-2.29190664293025,5.15554484377279));
#18909=CARTESIAN_POINT('Ctrl Pts',(3.80876232171537,-2.52413791100821,5.14443105471598));
#18910=CARTESIAN_POINT('Ctrl Pts',(3.60892556988421,-2.64269428158759,5.13331726565918));
#18911=CARTESIAN_POINT('Ctrl Pts',(3.40093972078443,-2.539134825312,5.12220347660237));
#18912=CARTESIAN_POINT('Ctrl Pts',(3.37514572416652,-2.30821119768585,5.11108968754557));
#18913=CARTESIAN_POINT('Ctrl Pts',(3.55516853033383,-2.16130913937078,5.09997589848876));
#18914=CARTESIAN_POINT('Ctrl Pts',(3.77622352465696,-2.23288041708187,5.08886210943196));
#18915=CARTESIAN_POINT('Ctrl Pts',(3.83598040928192,-2.457419700552,5.07774832037515));
#18916=CARTESIAN_POINT('Ctrl Pts',(3.67974110927284,-2.62940130358481,5.06663453131835));
#18917=CARTESIAN_POINT('Ctrl Pts',(3.45051418720664,-2.59140968013522,5.05552074226155));
#18918=CARTESIAN_POINT('Ctrl Pts',(3.35811316524308,-2.37821841178234,5.04440695320474));
#18919=CARTESIAN_POINT('Ctrl Pts',(3.48711398605093,-2.18496417501817,5.03329316414794));
#18920=CARTESIAN_POINT('Ctrl Pts',(3.71944061581356,-2.18853461914439,5.02217937509113));
#18921=CARTESIAN_POINT('Ctrl Pts',(3.84244191526684,-2.38566174871763,5.01106558603433));
#18922=CARTESIAN_POINT('Ctrl Pts',(3.74353337026135,-2.59591283022398,4.99995179697752));
#18923=CARTESIAN_POINT('Ctrl Pts',(3.51324710863985,-2.62684268245385,4.98883800792072));
#18924=CARTESIAN_POINT('Ctrl Pts',(3.36236674984584,-2.4501408518507,4.97772421886391));
#18925=CARTESIAN_POINT('Ctrl Pts',(3.42899480110061,-2.22754453241715,4.96661042980712));
#18926=CARTESIAN_POINT('Ctrl Pts',(3.65214584962031,-2.16279865748873,4.9554966407503));
#18927=CARTESIAN_POINT('Ctrl Pts',(3.82756721091734,-2.31516586178242,4.94438285169351));
#18928=CARTESIAN_POINT('Ctrl Pts',(3.79469372311971,-2.54518271468373,4.9332690626367));
#18929=CARTESIAN_POINT('Ctrl Pts',(3.58361486265069,-2.64231218244471,4.9221552735799));
#18930=CARTESIAN_POINT('Ctrl Pts',(3.38753350417909,-2.51765056156021,4.91104148452309));
#18931=CARTESIAN_POINT('Ctrl Pts',(3.38592513888554,-2.28530204745491,4.89992769546629));
#18932=CARTESIAN_POINT('Ctrl Pts',(3.5802619217345,-2.1579378700657,4.88881390640948));
#18933=CARTESIAN_POINT('Ctrl Pts',(3.7926651914697,-2.25213590538246,4.87770011735268));
#18934=CARTESIAN_POINT('Ctrl Pts',(3.8287198264784,-2.48167562339262,4.86658632829587));
#18935=CARTESIAN_POINT('Ctrl Pts',(3.65542461045338,-2.63645671704841,4.85547253923907));
#18936=CARTESIAN_POINT('Ctrl Pts',(3.43139861992193,-2.5748062959875,4.84435875018227));
#18937=CARTESIAN_POINT('Ctrl Pts',(3.36169538464595,-2.35315368977137,4.83324496112546));
#18938=CARTESIAN_POINT('Ctrl Pts',(3.51011506636152,-2.17438004258061,4.82213117206865));
#18939=CARTESIAN_POINT('Ctrl Pts',(3.74080744720095,-2.20211890112026,4.81101738301186));
#18940=CARTESIAN_POINT('Ctrl Pts',(3.84261717475225,-2.41098057358878,4.79990359395505));
#18941=CARTESIAN_POINT('Ctrl Pts',(3.72235665078693,-2.60979160252334,4.78878980489825));
#18942=CARTESIAN_POINT('Ctrl Pts',(3.49010169673754,-2.61657799846968,4.77767601584144));
#18943=CARTESIAN_POINT('Ctrl Pts',(3.3584379059958,-2.42512809625518,4.76656222678464));
#18944=CARTESIAN_POINT('Ctrl Pts',(3.44787863939658,-2.21067816256631,4.75544843772783));
#18945=CARTESIAN_POINT('Ctrl Pts',(3.67655777933124,-2.16951665373617,4.74433464867103));
#18946=CARTESIAN_POINT('Ctrl Pts',(3.83516271561975,-2.33931916560024,4.73322085961422));
#18947=CARTESIAN_POINT('Ctrl Pts',(3.77852055137491,-2.56466353335787,4.72210707055742));
#18948=CARTESIAN_POINT('Ctrl Pts',(3.55847650189588,-2.63928950162157,4.71099328150062));
#18949=CARTESIAN_POINT('Ctrl Pts',(3.37643938114003,-2.49489107532353,4.69987949244381));
#18950=CARTESIAN_POINT('Ctrl Pts',(3.39902983017658,-2.26363777164387,4.68876570338701));
#18951=CARTESIAN_POINT('Ctrl Pts',(3.60557055480924,-2.15719836203143,4.6776519143302));
#18952=CARTESIAN_POINT('Ctrl Pts',(3.8070124874506,-2.27299804520947,4.6665381252734));
#18953=CARTESIAN_POINT('Ctrl Pts',(3.81897354264718,-2.50504405790744,4.65542433621659));
#18954=CARTESIAN_POINT('Ctrl Pts',(3.63050563092984,-2.64094205312202,4.64431054715979));
#18955=CARTESIAN_POINT('Ctrl Pts',(3.4141155692652,-2.55630305464544,4.63319675810298));
#18956=CARTESIAN_POINT('Ctrl Pts',(3.3678676351246,-2.32859809765437,4.62208296904619));
#18957=CARTESIAN_POINT('Ctrl Pts',(3.53409308711521,-2.16624811163355,4.61096917998937));
#18958=CARTESIAN_POINT('Ctrl Pts',(3.76064388390312,-2.21785387995996,4.59985539093258));
#18959=CARTESIAN_POINT('Ctrl Pts',(3.8401555119317,-2.4361800576391,4.58874160187577));
#18960=CARTESIAN_POINT('Ctrl Pts',(3.69985007633495,-2.62139021824623,4.57762781281896));
#18961=CARTESIAN_POINT('Ctrl Pts',(3.46815073350293,-2.60395940136712,4.56651402376216));
#18962=CARTESIAN_POINT('Ctrl Pts',(3.35713451954606,-2.39984223133897,4.55540023470536));
#18963=CARTESIAN_POINT('Ctrl Pts',(3.46841583417461,-2.19586946879708,4.54428644564855));
#18964=CARTESIAN_POINT('Ctrl Pts',(3.70013762796088,-2.17873969637961,4.53317265659175));
#18965=CARTESIAN_POINT('Ctrl Pts',(3.84020231541317,-2.36413198929513,4.52205886753494));
#18966=CARTESIAN_POINT('Ctrl Pts',(3.7604070991348,-2.58235467884591,4.51094507847814));
#18967=CARTESIAN_POINT('Ctrl Pts',(3.53378944658573,-2.63366606347461,4.49983128942134));
#18968=CARTESIAN_POINT('Ctrl Pts',(3.36777506303883,-2.47110024891367,4.48871750036453));
#18969=CARTESIAN_POINT('Ctrl Pts',(3.41431880073856,-2.24345557286895,4.47760371130772));
#18970=CARTESIAN_POINT('Ctrl Pts',(3.63081864021225,-2.15909778094929,4.46648992225093));
#18971=CARTESIAN_POINT('Ctrl Pts',(3.81910984016012,-2.29524053287965,4.45537613319411));
#18972=CARTESIAN_POINT('Ctrl Pts',(3.80684729577664,-2.52727079162485,4.44426234413733));
#18973=CARTESIAN_POINT('Ctrl Pts',(3.60525512132335,-2.64280869447754,4.4331485550805));
#18974=CARTESIAN_POINT('Ctrl Pts',(3.39885278350865,-2.53610095948868,4.42203476602371));
#18975=CARTESIAN_POINT('Ctrl Pts',(3.37656295673162,-2.30481864526098,4.4109209769669));
#18976=CARTESIAN_POINT('Ctrl Pts',(3.55878722400007,-2.16065655916503,4.3998071879101));
#18977=CARTESIAN_POINT('Ctrl Pts',(3.77873474447839,-2.23556893008468,4.38869339885329));
#18978=CARTESIAN_POINT('Ctrl Pts',(3.83508286096032,-2.4609855401145,4.37757960979649));
#18979=CARTESIAN_POINT('Ctrl Pts',(3.67625990251943,-2.63058416437082,4.36646582073969));
#18980=CARTESIAN_POINT('Ctrl Pts',(3.44762951704948,-2.58912094093836,4.35535203168288));
#18981=CARTESIAN_POINT('Ctrl Pts',(3.35847732135144,-2.37456428079453,4.34423824262607));
#18982=CARTESIAN_POINT('Ctrl Pts',(3.49037003077072,-2.18326698967564,4.33312445356928));
#18983=CARTESIAN_POINT('Ctrl Pts',(3.72265543153543,-2.19039239422561,4.32201066451247));
#18984=CARTESIAN_POINT('Ctrl Pts',(3.84257847294968,-2.38928487404799,4.31089687545567));
#18985=CARTESIAN_POINT('Ctrl Pts',(3.74065691978671,-2.59816384879942,4.29978308639886));
#18986=CARTESIAN_POINT('Ctrl Pts',(3.50959628368763,-2.62529831625878,4.28866929734206));
#18987=CARTESIAN_POINT('Ctrl Pts',(3.41142456563631,-2.50643134569449,4.28126010463752));
#18988=CARTESIAN_POINT('Ctrl Pts',(3.39833241385534,-2.439372075429,4.27755550828525));
#18989=CARTESIAN_POINT('Ctrl Pts',(3.55032651029123,-2.58599788000028,5.20748149723825));
#18990=CARTESIAN_POINT('Ctrl Pts',(3.48847779011663,-2.5694802628904,5.20377690088598));
#18991=CARTESIAN_POINT('Ctrl Pts',(3.38363100808545,-2.4701274930924,5.19636770818144));
#18992=CARTESIAN_POINT('Ctrl Pts',(3.42374110325997,-2.25587321805223,5.18525391912464));
#18993=CARTESIAN_POINT('Ctrl Pts',(3.62549702156375,-2.17393147043888,5.17414013006783));
#18994=CARTESIAN_POINT('Ctrl Pts',(3.80376021494099,-2.29872357809039,5.16302634101103));
#18995=CARTESIAN_POINT('Ctrl Pts',(3.79559667259879,-2.51630912195772,5.15191255195423));
#18996=CARTESIAN_POINT('Ctrl Pts',(3.60836267654075,-2.62738870475875,5.14079876289742));
#18997=CARTESIAN_POINT('Ctrl Pts',(3.41349350811379,-2.53036025203219,5.12968497384062));
#18998=CARTESIAN_POINT('Ctrl Pts',(3.38932621647788,-2.31399988193773,5.11857118478382));
#18999=CARTESIAN_POINT('Ctrl Pts',(3.55799583841393,-2.17636223943479,5.10745739572701));
#19000=CARTESIAN_POINT('Ctrl Pts',(3.76510994308412,-2.24341985624469,5.09634360667021));
#19001=CARTESIAN_POINT('Ctrl Pts',(3.8210982445241,-2.45379851247728,5.0852298176134));
#19002=CARTESIAN_POINT('Ctrl Pts',(3.67471221585842,-2.61493405180745,5.0741160285566));
#19003=CARTESIAN_POINT('Ctrl Pts',(3.4599415481546,-2.57933837979007,5.0630022394998));
#19004=CARTESIAN_POINT('Ctrl Pts',(3.3733678202314,-2.37959207320419,5.05188845044299));
#19005=CARTESIAN_POINT('Ctrl Pts',(3.49423317134075,-2.19852546421989,5.04077466138618));
#19006=CARTESIAN_POINT('Ctrl Pts',(3.71190806288376,-2.20187073737575,5.02966087232939));
#19007=CARTESIAN_POINT('Ctrl Pts',(3.82715225398445,-2.38656599419535,5.01854708327258));
#19008=CARTESIAN_POINT('Ctrl Pts',(3.73448140162136,-2.58355753756882,5.00743329421578));
#19009=CARTESIAN_POINT('Ctrl Pts',(3.51871820188173,-2.61253679077134,4.99631950515897));
#19010=CARTESIAN_POINT('Ctrl Pts',(3.37735315143523,-2.44697870622763,4.98520571610217));
#19011=CARTESIAN_POINT('Ctrl Pts',(3.4397792876273,-2.23842048050862,4.97409192704536));
#19012=CARTESIAN_POINT('Ctrl Pts',(3.64885725830102,-2.17775782071235,4.96297813798855));
#19013=CARTESIAN_POINT('Ctrl Pts',(3.81321562666231,-2.3205159483675,4.95186434893175));
#19014=CARTESIAN_POINT('Ctrl Pts',(3.78241531376532,-2.53602672971665,4.94075055987495));
#19015=CARTESIAN_POINT('Ctrl Pts',(3.5846481955208,-2.62703070279587,4.92963677081815));
#19016=CARTESIAN_POINT('Ctrl Pts',(3.40093275798132,-2.51023089885891,4.91852298176134));
#19017=CARTESIAN_POINT('Ctrl Pts',(3.39942582465563,-2.29253550311487,4.90740919270454));
#19018=CARTESIAN_POINT('Ctrl Pts',(3.5815067086795,-2.17320358008914,4.89629540364773));
#19019=CARTESIAN_POINT('Ctrl Pts',(3.78051471198171,-2.26146099225962,4.88518161459093));
#19020=CARTESIAN_POINT('Ctrl Pts',(3.81429555222874,-2.47652472935135,4.87406782553412));
#19021=CARTESIAN_POINT('Ctrl Pts',(3.65192924324508,-2.6215445138197,4.86295403647732));
#19022=CARTESIAN_POINT('Ctrl Pts',(3.44203150900096,-2.56378209230252,4.85184024742051));
#19023=CARTESIAN_POINT('Ctrl Pts',(3.37672412605308,-2.35610806428593,4.84072645836371));
#19024=CARTESIAN_POINT('Ctrl Pts',(3.5157836826493,-2.18860882279666,4.8296126693069));
#19025=CARTESIAN_POINT('Ctrl Pts',(3.73192738959469,-2.2145983231407,4.8184988802501));
#19026=CARTESIAN_POINT('Ctrl Pts',(3.82731646068567,-2.41028808091203,4.8073850911933));
#19027=CARTESIAN_POINT('Ctrl Pts',(3.71464019736706,-2.59656104154983,4.79627130213649));
#19028=CARTESIAN_POINT('Ctrl Pts',(3.49703246129012,-2.60291945170324,4.78515751307969));
#19029=CARTESIAN_POINT('Ctrl Pts',(3.37367208112564,-2.42354338644957,4.77404372402289));
#19030=CARTESIAN_POINT('Ctrl Pts',(3.45747221184004,-2.22261779257846,4.76292993496608));
#19031=CARTESIAN_POINT('Ctrl Pts',(3.6717296434323,-2.18405214481133,4.75181614590928));
#19032=CARTESIAN_POINT('Ctrl Pts',(3.8203321189215,-2.34314601791364,4.74070235685247));
#19033=CARTESIAN_POINT('Ctrl Pts',(3.76726210722566,-2.55427898558761,4.72958856779567));
#19034=CARTESIAN_POINT('Ctrl Pts',(3.56109519190488,-2.62419864811054,4.71847477873887));
#19035=CARTESIAN_POINT('Ctrl Pts',(3.39053828864408,-2.4889067454323,4.70736098968206));
#19036=CARTESIAN_POINT('Ctrl Pts',(3.41170406524473,-2.2722374903888,4.69624720062525));
#19037=CARTESIAN_POINT('Ctrl Pts',(3.60521924634802,-2.17251070931785,4.68513341156845));
#19038=CARTESIAN_POINT('Ctrl Pts',(3.79395719207867,-2.28100745591228,4.67401962251165));
#19039=CARTESIAN_POINT('Ctrl Pts',(3.80516392027559,-2.49841942757747,4.66290583345484));
#19040=CARTESIAN_POINT('Ctrl Pts',(3.62858178552708,-2.6257469810287,4.65179204439804));
#19041=CARTESIAN_POINT('Ctrl Pts',(3.4258384183463,-2.54644576259963,4.64067825534124));
#19042=CARTESIAN_POINT('Ctrl Pts',(3.3825071219795,-2.3331010768549,4.62956446628443));
#19043=CARTESIAN_POINT('Ctrl Pts',(3.53824952340251,-2.18098973415088,4.61845067722763));
#19044=CARTESIAN_POINT('Ctrl Pts',(3.75051283635195,-2.22934097152269,4.60733688817082));
#19045=CARTESIAN_POINT('Ctrl Pts',(3.82501004325936,-2.43389835306723,4.59622309911402));
#19046=CARTESIAN_POINT('Ctrl Pts',(3.69355300577889,-2.607428187611,4.58510931005722));
#19047=CARTESIAN_POINT('Ctrl Pts',(3.47646584115605,-2.59109664964851,4.57399552100041));
#19048=CARTESIAN_POINT('Ctrl Pts',(3.37245089307511,-2.39985218105986,4.56288173194361));
#19049=CARTESIAN_POINT('Ctrl Pts',(3.47671422318619,-2.20874301286248,4.5517679428868));
#19050=CARTESIAN_POINT('Ctrl Pts',(3.69382242288812,-2.1926935339158,4.54065415383));
#19051=CARTESIAN_POINT('Ctrl Pts',(3.82505389506733,-2.36639401454743,4.52954036477319));
#19052=CARTESIAN_POINT('Ctrl Pts',(3.75029098447549,-2.57085443446884,4.51842657571639));
#19053=CARTESIAN_POINT('Ctrl Pts',(3.53796503204054,-2.61892985352599,4.50731278665959));
#19054=CARTESIAN_POINT('Ctrl Pts',(3.38242038797595,-2.46661629356384,4.49619899760278));
#19055=CARTESIAN_POINT('Ctrl Pts',(3.42602883297491,-2.25332808713219,4.48508520854598));
#19056=CARTESIAN_POINT('Ctrl Pts',(3.62887505479918,-2.17429034089672,4.47397141948917));
#19057=CARTESIAN_POINT('Ctrl Pts',(3.80529162215107,-2.30184721541898,4.46285763043237));
#19058=CARTESIAN_POINT('Ctrl Pts',(3.7938024182598,-2.51924442665844,4.45174384137557));
#19059=CARTESIAN_POINT('Ctrl Pts',(3.60492370575545,-2.62749590217058,4.44063005231876));
#19060=CARTESIAN_POINT('Ctrl Pts',(3.41153818407012,-2.52751771773158,4.42951626326196));
#19061=CARTESIAN_POINT('Ctrl Pts',(3.39065407090943,-2.31082128169766,4.41840247420515));
#19062=CARTESIAN_POINT('Ctrl Pts',(3.56138631824024,-2.17575081436632,4.40728868514835));
#19063=CARTESIAN_POINT('Ctrl Pts',(3.76746279218639,-2.24593881748859,4.39617489609154));
#19064=CARTESIAN_POINT('Ctrl Pts',(3.82025730031655,-2.4571394714574,4.38506110703474));
#19065=CARTESIAN_POINT('Ctrl Pts',(3.67145055229768,-2.61604231517601,4.37394731797793));
#19066=CARTESIAN_POINT('Ctrl Pts',(3.45723880045736,-2.57719398051498,4.36283352892113));
#19067=CARTESIAN_POINT('Ctrl Pts',(3.37370901074182,-2.37616839092003,4.35171973986433));
#19068=CARTESIAN_POINT('Ctrl Pts',(3.49728387276899,-2.19693531230428,4.34060595080752));
#19069=CARTESIAN_POINT('Ctrl Pts',(3.71492013543138,-2.20361135139717,4.32949216175072));
#19070=CARTESIAN_POINT('Ctrl Pts',(3.82728019962215,-2.38996062620176,4.31837837269391));
#19071=CARTESIAN_POINT('Ctrl Pts',(3.73178635523027,-2.58566659508311,4.30726458363711));
#19072=CARTESIAN_POINT('Ctrl Pts',(3.51529761713718,-2.61108982042464,4.29615079458031));
#19073=CARTESIAN_POINT('Ctrl Pts',(3.42331712354828,-2.49971922570605,4.28874160187577));
#19074=CARTESIAN_POINT('Ctrl Pts',(3.41105063166184,-2.43688906544027,4.2850370055235));
#19075=CARTESIAN_POINT('Ctrl Pts',(3.55367004230132,-2.57347832743338,5.2149629944765));
#19076=CARTESIAN_POINT('Ctrl Pts',(3.49598437120782,-2.55807251426281,5.21125839812423));
#19077=CARTESIAN_POINT('Ctrl Pts',(3.39819484595347,-2.4654071982366,5.2038492054197));
#19078=CARTESIAN_POINT('Ctrl Pts',(3.43560512301717,-2.2655744190707,5.19273541636288));
#19079=CARTESIAN_POINT('Ctrl Pts',(3.62378081220822,-2.18914818602487,5.18162162730609));
#19080=CARTESIAN_POINT('Ctrl Pts',(3.7900450762416,-2.30554051325052,5.17050783824928));
#19081=CARTESIAN_POINT('Ctrl Pts',(3.78243102348222,-2.50848033290724,5.15939404919248));
#19082=CARTESIAN_POINT('Ctrl Pts',(3.60779978319727,-2.6120831279299,5.14828026013567));
#19083=CARTESIAN_POINT('Ctrl Pts',(3.42604729544316,-2.52158567875239,5.13716647107887));
#19084=CARTESIAN_POINT('Ctrl Pts',(3.40350670878923,-2.3197885661896,5.12605268202206));
#19085=CARTESIAN_POINT('Ctrl Pts',(3.56082314649402,-2.19141533949881,5.11493889296526));
#19086=CARTESIAN_POINT('Ctrl Pts',(3.75399636151128,-2.25395929540751,5.10382510390846));
#19087=CARTESIAN_POINT('Ctrl Pts',(3.80621607976629,-2.45017732440257,5.09271131485166));
#19088=CARTESIAN_POINT('Ctrl Pts',(3.66968332244401,-2.60046680003009,5.08159752579485));
#19089=CARTESIAN_POINT('Ctrl Pts',(3.46936890910255,-2.56726707944493,5.07048373673804));
#19090=CARTESIAN_POINT('Ctrl Pts',(3.38862247521972,-2.38096573462603,5.05936994768124));
#19091=CARTESIAN_POINT('Ctrl Pts',(3.50135235663055,-2.21208675342161,5.04825615862443));
#19092=CARTESIAN_POINT('Ctrl Pts',(3.70437550995396,-2.2152068556071,5.03714236956763));
#19093=CARTESIAN_POINT('Ctrl Pts',(3.81186259270206,-2.38747023967307,5.02602858051083));
#19094=CARTESIAN_POINT('Ctrl Pts',(3.72542943298136,-2.57120224491366,5.01491479145402));
#19095=CARTESIAN_POINT('Ctrl Pts',(3.52418929512361,-2.59823089908883,5.00380100239722));
#19096=CARTESIAN_POINT('Ctrl Pts',(3.39233955302463,-2.44381656060457,4.99268721334042));
#19097=CARTESIAN_POINT('Ctrl Pts',(3.45056377415398,-2.24929642860009,4.98157342428361));
#19098=CARTESIAN_POINT('Ctrl Pts',(3.64556866698174,-2.19271698393598,4.97045963522681));
#19099=CARTESIAN_POINT('Ctrl Pts',(3.79886404240727,-2.32586603495258,4.95934584617));
#19100=CARTESIAN_POINT('Ctrl Pts',(3.77013690441093,-2.52687074474958,4.9482320571132));
#19101=CARTESIAN_POINT('Ctrl Pts',(3.58568152839091,-2.61174922314702,4.93711826805639));
#19102=CARTESIAN_POINT('Ctrl Pts',(3.41433201178354,-2.5028112361576,4.92600447899959));
#19103=CARTESIAN_POINT('Ctrl Pts',(3.41292651042572,-2.29976895877483,4.91489068994279));
#19104=CARTESIAN_POINT('Ctrl Pts',(3.58275149562449,-2.18846929011257,4.90377690088598));
#19105=CARTESIAN_POINT('Ctrl Pts',(3.76836423249372,-2.27078607913679,4.89266311182918));
#19106=CARTESIAN_POINT('Ctrl Pts',(3.79987127797908,-2.47137383531008,4.88154932277237));
#19107=CARTESIAN_POINT('Ctrl Pts',(3.64843387603678,-2.60663231059099,4.87043553371557));
#19108=CARTESIAN_POINT('Ctrl Pts',(3.45266439807998,-2.55275788861754,4.85932174465877));
#19109=CARTESIAN_POINT('Ctrl Pts',(3.39175286746021,-2.35906243880049,4.84820795560196));
#19110=CARTESIAN_POINT('Ctrl Pts',(3.52145229893708,-2.20283760301271,4.83709416654516));
#19111=CARTESIAN_POINT('Ctrl Pts',(3.72304733198844,-2.22707774516114,4.82598037748835));
#19112=CARTESIAN_POINT('Ctrl Pts',(3.81201574661908,-2.40959558823528,4.81486658843155));
#19113=CARTESIAN_POINT('Ctrl Pts',(3.7069237439472,-2.58333048057632,4.80375279937474));
#19114=CARTESIAN_POINT('Ctrl Pts',(3.50396322584271,-2.58926090493679,4.79263901031794));
#19115=CARTESIAN_POINT('Ctrl Pts',(3.38890625625548,-2.42195867664397,4.78152522126113));
#19116=CARTESIAN_POINT('Ctrl Pts',(3.46706578428349,-2.2345574225906,4.77041143220433));
#19117=CARTESIAN_POINT('Ctrl Pts',(3.66690150753336,-2.19858763588649,4.75929764314752));
#19118=CARTESIAN_POINT('Ctrl Pts',(3.80550152222325,-2.34697287022705,4.74818385409073));
#19119=CARTESIAN_POINT('Ctrl Pts',(3.75600366307642,-2.54389443781734,4.73707006503391));
#19120=CARTESIAN_POINT('Ctrl Pts',(3.56371388191388,-2.60910779459951,4.72595627597711));
#19121=CARTESIAN_POINT('Ctrl Pts',(3.40463719614813,-2.48292241554106,4.71484248692031));
#19122=CARTESIAN_POINT('Ctrl Pts',(3.42437830031288,-2.28083720913373,4.7037286978635));
#19123=CARTESIAN_POINT('Ctrl Pts',(3.60486793788679,-2.18782305660426,4.6926149088067));
#19124=CARTESIAN_POINT('Ctrl Pts',(3.78090189670674,-2.28901686661509,4.6815011197499));
#19125=CARTESIAN_POINT('Ctrl Pts',(3.79135429790399,-2.4917947972475,4.67038733069309));
#19126=CARTESIAN_POINT('Ctrl Pts',(3.62665794012432,-2.6105519089354,4.65927354163629));
#19127=CARTESIAN_POINT('Ctrl Pts',(3.43756126742739,-2.53658847055381,4.64815975257948));
#19128=CARTESIAN_POINT('Ctrl Pts',(3.3971466088344,-2.33760405605543,4.63704596352268));
#19129=CARTESIAN_POINT('Ctrl Pts',(3.54240595968981,-2.19573135666821,4.62593217446587));
#19130=CARTESIAN_POINT('Ctrl Pts',(3.74038178880077,-2.24082806308542,4.61481838540907));
#19131=CARTESIAN_POINT('Ctrl Pts',(3.80986457458702,-2.43161664849535,4.60370459635227));
#19132=CARTESIAN_POINT('Ctrl Pts',(3.68725593522283,-2.59346615697577,4.59259080729546));
#19133=CARTESIAN_POINT('Ctrl Pts',(3.48478094880917,-2.57823389792989,4.58147701823866));
#19134=CARTESIAN_POINT('Ctrl Pts',(3.38776726660417,-2.39986213078074,4.57036322918185));
#19135=CARTESIAN_POINT('Ctrl Pts',(3.48501261219776,-2.22161655692788,4.55924944012505));
#19136=CARTESIAN_POINT('Ctrl Pts',(3.68750721781536,-2.20664737145198,4.54813565106824));
#19137=CARTESIAN_POINT('Ctrl Pts',(3.80990547472148,-2.36865603979974,4.53702186201144));
#19138=CARTESIAN_POINT('Ctrl Pts',(3.74017486981618,-2.55935419009178,4.52590807295464));
#19139=CARTESIAN_POINT('Ctrl Pts',(3.54214061749534,-2.60419364357738,4.51479428389783));
#19140=CARTESIAN_POINT('Ctrl Pts',(3.39706571291307,-2.46213233821401,4.50368049484103));
#19141=CARTESIAN_POINT('Ctrl Pts',(3.43773886521125,-2.26320060139544,4.49256670578422));
#19142=CARTESIAN_POINT('Ctrl Pts',(3.62693146938611,-2.18948290084415,4.48145291672742));
#19143=CARTESIAN_POINT('Ctrl Pts',(3.79147340414203,-2.30845389795831,4.47033912767061));
#19144=CARTESIAN_POINT('Ctrl Pts',(3.78075754074296,-2.51121806169204,4.45922533861382));
#19145=CARTESIAN_POINT('Ctrl Pts',(3.60459229018754,-2.61218310986363,4.44811154955701));
#19146=CARTESIAN_POINT('Ctrl Pts',(3.42422358463158,-2.51893447597448,4.4369977605002));
#19147=CARTESIAN_POINT('Ctrl Pts',(3.40474518508724,-2.31682391813433,4.4258839714434));
#19148=CARTESIAN_POINT('Ctrl Pts',(3.56398541248042,-2.19084506956762,4.41477018238659));
#19149=CARTESIAN_POINT('Ctrl Pts',(3.75619083989438,-2.25630870489251,4.40365639332979));
#19150=CARTESIAN_POINT('Ctrl Pts',(3.80543173967279,-2.4532934028003,4.39254260427299));
#19151=CARTESIAN_POINT('Ctrl Pts',(3.66664120207593,-2.60150046598119,4.38142881521619));
#19152=CARTESIAN_POINT('Ctrl Pts',(3.46684808386524,-2.5652670200916,4.37031502615938));
#19153=CARTESIAN_POINT('Ctrl Pts',(3.3889407001322,-2.37777250104553,4.35920123710258));
#19154=CARTESIAN_POINT('Ctrl Pts',(3.50419771476727,-2.21060363493292,4.34808744804577));
#19155=CARTESIAN_POINT('Ctrl Pts',(3.70718483932733,-2.21683030856873,4.33697365898897));
#19156=CARTESIAN_POINT('Ctrl Pts',(3.81198192629463,-2.39063637835552,4.32585986993216));
#19157=CARTESIAN_POINT('Ctrl Pts',(3.72291579067381,-2.5731693413668,4.31474608087536));
#19158=CARTESIAN_POINT('Ctrl Pts',(3.52099895058674,-2.5968813245905,4.30363229181856));
#19159=CARTESIAN_POINT('Ctrl Pts',(3.43520968146025,-2.49300710571762,4.29622309911402));
#19160=CARTESIAN_POINT('Ctrl Pts',(3.42376884946835,-2.43440605545154,4.29251850276175));
#19161=CARTESIAN_POINT('Ctrl Pts',(3.55701357431141,-2.56095877486649,5.22244449171475));
#19162=CARTESIAN_POINT('Ctrl Pts',(3.50349095229901,-2.54666476563522,5.21873989536248));
#19163=CARTESIAN_POINT('Ctrl Pts',(3.41275868382149,-2.4606869033808,5.21133070265794));
#19164=CARTESIAN_POINT('Ctrl Pts',(3.44746914277437,-2.27527562008917,5.20021691360114));
#19165=CARTESIAN_POINT('Ctrl Pts',(3.62206460285268,-2.20436490161086,5.18910312454433));
#19166=CARTESIAN_POINT('Ctrl Pts',(3.77632993754221,-2.31235744841065,5.17798933548754));
#19167=CARTESIAN_POINT('Ctrl Pts',(3.76926537436564,-2.50065154385676,5.16687554643072));
#19168=CARTESIAN_POINT('Ctrl Pts',(3.6072368898538,-2.59677755110107,5.15576175737393));
#19169=CARTESIAN_POINT('Ctrl Pts',(3.43860108277253,-2.51281110547259,5.14464796831712));
#19170=CARTESIAN_POINT('Ctrl Pts',(3.41768720110058,-2.32557725044148,5.13353417926032));
#19171=CARTESIAN_POINT('Ctrl Pts',(3.56365045457412,-2.20646843956283,5.12242039020351));
#19172=CARTESIAN_POINT('Ctrl Pts',(3.74288277993844,-2.26449873457034,5.11130660114671));
#19173=CARTESIAN_POINT('Ctrl Pts',(3.79133391500848,-2.44655613632785,5.1001928120899));
#19174=CARTESIAN_POINT('Ctrl Pts',(3.66465442902959,-2.58599954825273,5.0890790230331));
#19175=CARTESIAN_POINT('Ctrl Pts',(3.4787962700505,-2.55519577909978,5.0779652339763));
#19176=CARTESIAN_POINT('Ctrl Pts',(3.40387713020803,-2.38233939604788,5.06685144491948));
#19177=CARTESIAN_POINT('Ctrl Pts',(3.50847154192036,-2.22564804262333,5.05573765586269));
#19178=CARTESIAN_POINT('Ctrl Pts',(3.69684295702416,-2.22854297383845,5.04462386680588));
#19179=CARTESIAN_POINT('Ctrl Pts',(3.79657293141967,-2.38837448515078,5.03351007774908));
#19180=CARTESIAN_POINT('Ctrl Pts',(3.71637746434136,-2.5588469522585,5.02239628869228));
#19181=CARTESIAN_POINT('Ctrl Pts',(3.52966038836549,-2.58392500740631,5.01128249963547));
#19182=CARTESIAN_POINT('Ctrl Pts',(3.40732595461402,-2.44065441498151,5.00016871057866));
#19183=CARTESIAN_POINT('Ctrl Pts',(3.46134826068067,-2.26017237669156,4.98905492152187));
#19184=CARTESIAN_POINT('Ctrl Pts',(3.64228007566245,-2.20767614715961,4.97794113246505));
#19185=CARTESIAN_POINT('Ctrl Pts',(3.78451245815223,-2.33121612153766,4.96682734340826));
#19186=CARTESIAN_POINT('Ctrl Pts',(3.75785849505654,-2.5177147597825,4.95571355435145));
#19187=CARTESIAN_POINT('Ctrl Pts',(3.58671486126101,-2.59646774349818,4.94459976529464));
#19188=CARTESIAN_POINT('Ctrl Pts',(3.42773126558577,-2.49539157345629,4.93348597623784));
#19189=CARTESIAN_POINT('Ctrl Pts',(3.4264271961958,-2.30700241443478,4.92237218718104));
#19190=CARTESIAN_POINT('Ctrl Pts',(3.5839962825695,-2.20373500013601,4.91125839812423));
#19191=CARTESIAN_POINT('Ctrl Pts',(3.75621375300573,-2.28011116601395,4.90014460906743));
#19192=CARTESIAN_POINT('Ctrl Pts',(3.78544700372942,-2.46622294126882,4.88903082001062));
#19193=CARTESIAN_POINT('Ctrl Pts',(3.64493850882848,-2.59172010736228,4.87791703095382));
#19194=CARTESIAN_POINT('Ctrl Pts',(3.463297287159,-2.54173368493256,4.86680324189701));
#19195=CARTESIAN_POINT('Ctrl Pts',(3.40678160886734,-2.36201681331505,4.85568945284021));
#19196=CARTESIAN_POINT('Ctrl Pts',(3.52712091522486,-2.21706638322876,4.8445756637834));
#19197=CARTESIAN_POINT('Ctrl Pts',(3.71416727438218,-2.23955716718158,4.8334618747266));
#19198=CARTESIAN_POINT('Ctrl Pts',(3.7967150325525,-2.40890309555853,4.8223480856698));
#19199=CARTESIAN_POINT('Ctrl Pts',(3.69920729052733,-2.57009991960281,4.81123429661299));
#19200=CARTESIAN_POINT('Ctrl Pts',(3.5108939903953,-2.57560235817033,4.80012050755619));
#19201=CARTESIAN_POINT('Ctrl Pts',(3.40414043138533,-2.42037396683837,4.78900671849938));
#19202=CARTESIAN_POINT('Ctrl Pts',(3.47665935672695,-2.24649705260274,4.77789292944258));
#19203=CARTESIAN_POINT('Ctrl Pts',(3.66207337163443,-2.21312312696165,4.76677914038577));
#19204=CARTESIAN_POINT('Ctrl Pts',(3.790670925525,-2.35079972254045,4.75566535132897));
#19205=CARTESIAN_POINT('Ctrl Pts',(3.74474521892717,-2.53350989004707,4.74455156227217));
#19206=CARTESIAN_POINT('Ctrl Pts',(3.56633257192288,-2.59401694108847,4.73343777321536));
#19207=CARTESIAN_POINT('Ctrl Pts',(3.41873610365217,-2.47693808564983,4.72232398415856));
#19208=CARTESIAN_POINT('Ctrl Pts',(3.43705253538103,-2.28943692787866,4.71121019510175));
#19209=CARTESIAN_POINT('Ctrl Pts',(3.60451662942557,-2.20313540389068,4.70009640604496));
#19210=CARTESIAN_POINT('Ctrl Pts',(3.76784660133481,-2.29702627731791,4.68898261698814));
#19211=CARTESIAN_POINT('Ctrl Pts',(3.7775446755324,-2.48517016691753,4.67786882793135));
#19212=CARTESIAN_POINT('Ctrl Pts',(3.62473409472155,-2.59535683684209,4.66675503887453));
#19213=CARTESIAN_POINT('Ctrl Pts',(3.44928411650849,-2.526731178508,4.65564124981774));
#19214=CARTESIAN_POINT('Ctrl Pts',(3.4117860956893,-2.34210703525596,4.64452746076092));
#19215=CARTESIAN_POINT('Ctrl Pts',(3.5465623959771,-2.21047297918554,4.63341367170413));
#19216=CARTESIAN_POINT('Ctrl Pts',(3.73025074124959,-2.25231515464815,4.62229988264732));
#19217=CARTESIAN_POINT('Ctrl Pts',(3.79471910591469,-2.42933494392347,4.61118609359052));
#19218=CARTESIAN_POINT('Ctrl Pts',(3.68095886466676,-2.57950412634054,4.60007230453372));
#19219=CARTESIAN_POINT('Ctrl Pts',(3.49309605646229,-2.56537114621128,4.5889585154769));
#19220=CARTESIAN_POINT('Ctrl Pts',(3.40308364013322,-2.39987208050163,4.57784472642011));
#19221=CARTESIAN_POINT('Ctrl Pts',(3.49331100120934,-2.23449010099328,4.56673093736329));
#19222=CARTESIAN_POINT('Ctrl Pts',(3.68119201274259,-2.22060120898816,4.5556171483065));
#19223=CARTESIAN_POINT('Ctrl Pts',(3.79475705437564,-2.37091806505204,4.54450335924969));
#19224=CARTESIAN_POINT('Ctrl Pts',(3.73005875515687,-2.5478539457147,4.53338957019289));
#19225=CARTESIAN_POINT('Ctrl Pts',(3.54631620295015,-2.58945743362876,4.52227578113609));
#19226=CARTESIAN_POINT('Ctrl Pts',(3.4117110378502,-2.45764838286418,4.51116199207927));
#19227=CARTESIAN_POINT('Ctrl Pts',(3.4494488974476,-2.27307311565868,4.50004820302248));
#19228=CARTESIAN_POINT('Ctrl Pts',(3.62498788397304,-2.20467546079158,4.48893441396567));
#19229=CARTESIAN_POINT('Ctrl Pts',(3.77765518613299,-2.31506058049763,4.47782062490887));
#19230=CARTESIAN_POINT('Ctrl Pts',(3.76771266322612,-2.50319169672563,4.46670683585206));
#19231=CARTESIAN_POINT('Ctrl Pts',(3.60426087461964,-2.59687031755667,4.45559304679526));
#19232=CARTESIAN_POINT('Ctrl Pts',(3.43690898519305,-2.51035123421737,4.44447925773846));
#19233=CARTESIAN_POINT('Ctrl Pts',(3.41883629926506,-2.32282655457101,4.43336546868165));
#19234=CARTESIAN_POINT('Ctrl Pts',(3.56658450672058,-2.20593932476892,4.42225167962485));
#19235=CARTESIAN_POINT('Ctrl Pts',(3.74491888760239,-2.26667859229642,4.41113789056804));
#19236=CARTESIAN_POINT('Ctrl Pts',(3.79060617902903,-2.4494473341432,4.40002410151123));
#19237=CARTESIAN_POINT('Ctrl Pts',(3.66183185185417,-2.58695861678637,4.38891031245443));
#19238=CARTESIAN_POINT('Ctrl Pts',(3.47645736727312,-2.55334005966823,4.37779652339763));
#19239=CARTESIAN_POINT('Ctrl Pts',(3.40417238952257,-2.37937661117104,4.36668273434082));
#19240=CARTESIAN_POINT('Ctrl Pts',(3.51111155676555,-2.22427195756156,4.35556894528402));
#19241=CARTESIAN_POINT('Ctrl Pts',(3.69944954322327,-2.2300492657403,4.34445515622722));
#19242=CARTESIAN_POINT('Ctrl Pts',(3.79668365296711,-2.39131213050928,4.33334136717041));
#19243=CARTESIAN_POINT('Ctrl Pts',(3.71404522611737,-2.56067208765049,4.32222757811361));
#19244=CARTESIAN_POINT('Ctrl Pts',(3.5267002840363,-2.58267282875636,4.31111378905681));
#19245=CARTESIAN_POINT('Ctrl Pts',(3.44710223937223,-2.48629498572918,4.30370459635227));
#19246=CARTESIAN_POINT('Ctrl Pts',(3.43648706727485,-2.43192304546281,4.3));
#19247=CARTESIAN_POINT('Ctrl Pts',(3.43361559198215,-2.39990578567643,5.13785196366098));
#19248=CARTESIAN_POINT('Ctrl Pts',(3.43350388051965,-2.378317282854,5.13641270219409));
#19249=CARTESIAN_POINT('Ctrl Pts',(3.43740296507651,-2.35676746744261,5.1349734407272));
#19250=CARTESIAN_POINT('Ctrl Pts',(3.44550005695817,-2.33693142446689,5.13353417926032));
#19251=CARTESIAN_POINT('Ctrl Pts',(3.4663416189251,-2.28587431348193,5.12982958290805));
#19252=CARTESIAN_POINT('Ctrl Pts',(3.51499603674961,-2.24617137652238,5.12612498655578));
#19253=CARTESIAN_POINT('Ctrl Pts',(3.56919529988925,-2.23599162387719,5.12242039020351));
#19254=CARTESIAN_POINT('Ctrl Pts',(3.62339456302889,-2.225811871232,5.11871579385124));
#19255=CARTESIAN_POINT('Ctrl Pts',(3.68313867148366,-2.24515530290117,5.11501119749898));
#19256=CARTESIAN_POINT('Ctrl Pts',(3.72108591488939,-2.28516991902867,5.11130660114671));
#19257=CARTESIAN_POINT('Ctrl Pts',(3.75903315829512,-2.32518453515617,5.10760200479444));
#19258=CARTESIAN_POINT('Ctrl Pts',(3.7751835366518,-2.38587033574201,5.10389740844217));
#19259=CARTESIAN_POINT('Ctrl Pts',(3.76214547816699,-2.43945380468907,5.1001928120899));
#19260=CARTESIAN_POINT('Ctrl Pts',(3.74910741968218,-2.49303727363614,5.09648821573763));
#19261=CARTESIAN_POINT('Ctrl Pts',(3.70688092435589,-2.53951841094443,5.09278361938536));
#19262=CARTESIAN_POINT('Ctrl Pts',(3.65479131686289,-2.55762501807309,5.0890790230331));
#19263=CARTESIAN_POINT('Ctrl Pts',(3.60270170936989,-2.57573162520175,5.08537442668083));
#19264=CARTESIAN_POINT('Ctrl Pts',(3.5407489897102,-2.56546370215076,5.08166983032856));
#19265=CARTESIAN_POINT('Ctrl Pts',(3.49728610657327,-2.53152034344996,5.0779652339763));
#19266=CARTESIAN_POINT('Ctrl Pts',(3.45773596902793,-2.50063273525474,5.07459414387119));
#19267=CARTESIAN_POINT('Ctrl Pts',(3.43349642418942,-2.45014057555659,5.07122305376608));
#19268=CARTESIAN_POINT('Ctrl Pts',(3.43317939237559,-2.39991359865598,5.06785196366098));
#19269=CARTESIAN_POINT('Ctrl Pts',(3.54698297828114,-2.59851743256717,5.2));
#19270=CARTESIAN_POINT('Ctrl Pts',(3.53457951946873,-2.59392489162072,5.2));
#19271=CARTESIAN_POINT('Ctrl Pts',(3.52273021669441,-2.5880656264448,5.2));
#19272=CARTESIAN_POINT('Ctrl Pts',(3.51155282078554,-2.58110287559691,5.2));
#19273=CARTESIAN_POINT('Ctrl Pts',(3.50588661273558,-2.57757321670087,5.2));
#19274=CARTESIAN_POINT('Ctrl Pts',(3.50039351027032,-2.5737592340707,5.2));
#19275=CARTESIAN_POINT('Ctrl Pts',(3.49509228904167,-2.56967861696227,5.2));
#19276=CARTESIAN_POINT('Ctrl Pts',(3.4905050126104,-2.5661475591401,5.2));
#19277=CARTESIAN_POINT('Ctrl Pts',(3.48606143928385,-2.56241679614242,5.2));
#19278=CARTESIAN_POINT('Ctrl Pts',(3.48177554227615,-2.55849690369355,5.2));
#19279=CARTESIAN_POINT('Ctrl Pts',(3.47866533036506,-2.55565229586402,5.2));
#19280=CARTESIAN_POINT('Ctrl Pts',(3.47564434245519,-2.5527135073757,5.2));
#19281=CARTESIAN_POINT('Ctrl Pts',(3.47272197556915,-2.54969075241385,5.2));
#19282=CARTESIAN_POINT('Ctrl Pts',(3.4637769959157,-2.54043849809891,5.2));
#19283=CARTESIAN_POINT('Ctrl Pts',(3.45573629551605,-2.5303863939551,5.2));
#19284=CARTESIAN_POINT('Ctrl Pts',(3.44873891503949,-2.51966547725229,5.2));
#19285=CARTESIAN_POINT('Ctrl Pts',(3.44420807340926,-2.51272362581603,5.2));
#19286=CARTESIAN_POINT('Ctrl Pts',(3.44011549441187,-2.50550078770205,5.2));
#19287=CARTESIAN_POINT('Ctrl Pts',(3.43651065828778,-2.49802988469159,5.2));
#19288=CARTESIAN_POINT('Ctrl Pts',(3.43484392828386,-2.49457564217533,5.2));
#19289=CARTESIAN_POINT('Ctrl Pts',(3.43328559790363,-2.49107645830187,5.2));
#19290=CARTESIAN_POINT('Ctrl Pts',(3.43184079842385,-2.48753928615204,5.2));
#19291=CARTESIAN_POINT('Ctrl Pts',(3.4278386851231,-2.47774127341323,5.2));
#19292=CARTESIAN_POINT('Ctrl Pts',(3.42470153714545,-2.46764377419319,5.2));
#19293=CARTESIAN_POINT('Ctrl Pts',(3.42252346903458,-2.4573201729425,5.2));
#19294=CARTESIAN_POINT('Ctrl Pts',(3.42066967900374,-2.44853358404506,5.2));
#19295=CARTESIAN_POINT('Ctrl Pts',(3.41951138514856,-2.43958272486992,5.2));
#19296=CARTESIAN_POINT('Ctrl Pts',(3.4190359581172,-2.43054589510015,5.2));
#19297=CARTESIAN_POINT('Ctrl Pts',(3.41886681623208,-2.42733087718605,5.2));
#19298=CARTESIAN_POINT('Ctrl Pts',(3.41878446710974,-2.42410641682356,5.2));
#19299=CARTESIAN_POINT('Ctrl Pts',(3.4187879805801,-2.42088574908536,5.2));
#19300=CARTESIAN_POINT('Ctrl Pts',(3.41880075373106,-2.40917707615745,5.2));
#19301=CARTESIAN_POINT('Ctrl Pts',(3.41994281751926,-2.39748218187535,5.2));
#19302=CARTESIAN_POINT('Ctrl Pts',(3.42216878576612,-2.38597338048412,5.2));
#19303=CARTESIAN_POINT('Ctrl Pts',(3.42331180295367,-2.38006370148633,5.2));
#19304=CARTESIAN_POINT('Ctrl Pts',(3.4247413109463,-2.37420327369848,5.2));
#19305=CARTESIAN_POINT('Ctrl Pts',(3.42645509270942,-2.36841769265549,5.2));
#19306=CARTESIAN_POINT('Ctrl Pts',(3.42814232412983,-2.36272174330468,5.2));
#19307=CARTESIAN_POINT('Ctrl Pts',(3.430107844827,-2.35709290248798,5.2));
#19308=CARTESIAN_POINT('Ctrl Pts',(3.43233768211765,-2.35158848883877,5.2));
#19309=CARTESIAN_POINT('Ctrl Pts',(3.43579440103488,-2.34305548471816,5.2));
#19310=CARTESIAN_POINT('Ctrl Pts',(3.4398879741905,-2.33480787202203,5.2));
#19311=CARTESIAN_POINT('Ctrl Pts',(3.44460905895211,-2.32694151527758,5.2));
#19312=CARTESIAN_POINT('Ctrl Pts',(3.44702307993388,-2.32291922989401,5.2));
#19313=CARTESIAN_POINT('Ctrl Pts',(3.44960209197192,-2.31899653386197,5.2));
#19314=CARTESIAN_POINT('Ctrl Pts',(3.45233605539852,-2.31519993624376,5.2));
#19315=CARTESIAN_POINT('Ctrl Pts',(3.45777066118573,-2.30765301327221,5.2));
#19316=CARTESIAN_POINT('Ctrl Pts',(3.46382416246759,-2.30058959612096,5.2));
#19317=CARTESIAN_POINT('Ctrl Pts',(3.47049190863519,-2.29412081302041,5.2));
#19318=CARTESIAN_POINT('Ctrl Pts',(3.47127037804276,-2.29336557285059,5.2));
#19319=CARTESIAN_POINT('Ctrl Pts',(3.472057234472,-2.29261846360327,5.2));
#19320=CARTESIAN_POINT('Ctrl Pts',(3.47285232078577,-2.29187955100915,5.2));
#19321=CARTESIAN_POINT('Origin',(3.6,-2.4,4.7));
#19322=CARTESIAN_POINT('Origin',(3.6,2.4,4.3));
#19323=CARTESIAN_POINT('Ctrl Pts',(3.43648706727485,2.36807695453719,4.3));
#19324=CARTESIAN_POINT('Ctrl Pts',(3.43713128683271,2.3597806326638,4.3));
#19325=CARTESIAN_POINT('Ctrl Pts',(3.43844439010238,2.35157023568352,4.3));
#19326=CARTESIAN_POINT('Ctrl Pts',(3.44036779366958,2.34349709838219,4.3));
#19327=CARTESIAN_POINT('Ctrl Pts',(3.44142971905211,2.33903985936946,4.3));
#19328=CARTESIAN_POINT('Ctrl Pts',(3.44267796535882,2.33462439474099,4.3));
#19329=CARTESIAN_POINT('Ctrl Pts',(3.44410466805123,2.33025917432088,4.3));
#19330=CARTESIAN_POINT('Ctrl Pts',(3.44564438355751,2.32554817349018,4.3));
#19331=CARTESIAN_POINT('Ctrl Pts',(3.44738955334548,2.3209035962062,4.3));
#19332=CARTESIAN_POINT('Ctrl Pts',(3.4493265481332,2.31634215395336,4.3));
#19333=CARTESIAN_POINT('Ctrl Pts',(3.45254731917628,2.30875753823018,4.3));
#19334=CARTESIAN_POINT('Ctrl Pts',(3.45629959311852,2.30139710694769,4.3));
#19335=CARTESIAN_POINT('Ctrl Pts',(3.46054037353588,2.29430908064149,4.3));
#19336=CARTESIAN_POINT('Ctrl Pts',(3.46239353776121,2.29121170810954,4.3));
#19337=CARTESIAN_POINT('Ctrl Pts',(3.46433984867298,2.28816727138872,4.3));
#19338=CARTESIAN_POINT('Ctrl Pts',(3.46636983737831,2.28518826034786,4.3));
#19339=CARTESIAN_POINT('Ctrl Pts',(3.47324583140019,2.27509773026055,4.3));
#19340=CARTESIAN_POINT('Ctrl Pts',(3.48109365784268,2.26572974302294,4.3));
#19341=CARTESIAN_POINT('Ctrl Pts',(3.48977951837809,2.25723278343533,4.3));
#19342=CARTESIAN_POINT('Ctrl Pts',(3.49400932884437,2.25309496330239,4.3));
#19343=CARTESIAN_POINT('Ctrl Pts',(3.49843865454892,2.24916389122995,4.3));
#19344=CARTESIAN_POINT('Ctrl Pts',(3.50305598018317,2.24545876796073,4.3));
#19345=CARTESIAN_POINT('Ctrl Pts',(3.50696193979743,2.24232447269942,4.3));
#19346=CARTESIAN_POINT('Ctrl Pts',(3.51100698863209,2.23934939909905,4.3));
#19347=CARTESIAN_POINT('Ctrl Pts',(3.51515874429581,2.23656266075085,4.3));
#19348=CARTESIAN_POINT('Ctrl Pts',(3.52023402885856,2.23315603202204,4.3));
#19349=CARTESIAN_POINT('Ctrl Pts',(3.52547424287705,2.23002554171617,4.3));
#19350=CARTESIAN_POINT('Ctrl Pts',(3.53086412680946,2.22718930631114,4.3));
#19351=CARTESIAN_POINT('Ctrl Pts',(3.53843721702836,2.22320423596943,4.3));
#19352=CARTESIAN_POINT('Ctrl Pts',(3.54630546669305,2.21979946806346,4.3));
#19353=CARTESIAN_POINT('Ctrl Pts',(3.55440208317939,2.21695927394856,4.3));
#19354=CARTESIAN_POINT('Ctrl Pts',(3.56031223293849,2.21488606564082,4.3));
#19355=CARTESIAN_POINT('Ctrl Pts',(3.56634429400461,2.21311389140606,4.3));
#19356=CARTESIAN_POINT('Ctrl Pts',(3.57247452264395,2.21164027909917,4.3));
#19357=CARTESIAN_POINT('Ctrl Pts',(3.57600246534631,2.21079221614916,4.3));
#19358=CARTESIAN_POINT('Ctrl Pts',(3.57955843058062,2.21004433773534,4.3));
#19359=CARTESIAN_POINT('Ctrl Pts',(3.58312961367547,2.20939690917763,4.3));
#19360=CARTESIAN_POINT('Ctrl Pts',(3.59464652648698,2.20730897975681,4.3));
#19361=CARTESIAN_POINT('Ctrl Pts',(3.60634454881448,2.20625732608158,4.3));
#19362=CARTESIAN_POINT('Ctrl Pts',(3.61806689528204,2.2062086557371,4.3));
#19363=CARTESIAN_POINT('Ctrl Pts',(3.62473122101744,2.20618098593309,4.3));
#19364=CARTESIAN_POINT('Ctrl Pts',(3.63140379711974,2.20647808078856,4.3));
#19365=CARTESIAN_POINT('Ctrl Pts',(3.63805748358195,2.20709863975089,4.3));
#19366=CARTESIAN_POINT('Ctrl Pts',(3.64215439115276,2.20748073961769,4.3));
#19367=CARTESIAN_POINT('Ctrl Pts',(3.64624620849006,2.20798586737994,4.3));
#19368=CARTESIAN_POINT('Ctrl Pts',(3.65032009844121,2.20861337585159,4.3));
#19369=CARTESIAN_POINT('Ctrl Pts',(3.66357602962435,2.2106552103677,4.3));
#19370=CARTESIAN_POINT('Ctrl Pts',(3.67655558408475,2.21397441829708,4.3));
#19371=CARTESIAN_POINT('Ctrl Pts',(3.68904456814691,2.21853837010126,4.3));
#19372=CARTESIAN_POINT('Ctrl Pts',(3.69937753051516,2.22231442922732,4.3));
#19373=CARTESIAN_POINT('Ctrl Pts',(3.7093756794575,2.22694342372598,4.3));
#19374=CARTESIAN_POINT('Ctrl Pts',(3.71891590137671,2.23243384744346,4.3));
#19375=CARTESIAN_POINT('Ctrl Pts',(3.72007018093634,2.23309813847615,4.3));
#19376=CARTESIAN_POINT('Ctrl Pts',(3.72121774557788,2.23377506987061,4.3));
#19377=CARTESIAN_POINT('Ctrl Pts',(3.72235851517116,2.23446447326396,4.3));
#19378=CARTESIAN_POINT('Ctrl Pts',(3.78826275096636,2.31767678198967,4.3));
#19379=CARTESIAN_POINT('Ctrl Pts',(3.79091867322995,2.32572936860323,4.3));
#19380=CARTESIAN_POINT('Ctrl Pts',(3.79302804064853,2.33393960507108,4.3));
#19381=CARTESIAN_POINT('Ctrl Pts',(3.79460323981381,2.34225613442594,4.3));
#19382=CARTESIAN_POINT('Ctrl Pts',(3.79578956453863,2.34851953566168,4.3));
#19383=CARTESIAN_POINT('Ctrl Pts',(3.79667271897105,2.35484328449916,4.3));
#19384=CARTESIAN_POINT('Ctrl Pts',(3.79725488312451,2.36120517356094,4.3));
#19385=CARTESIAN_POINT('Ctrl Pts',(3.7976908683603,2.36596961961323,4.3));
#19386=CARTESIAN_POINT('Ctrl Pts',(3.79795758133253,2.37075408813906,4.3));
#19387=CARTESIAN_POINT('Ctrl Pts',(3.79805590956906,2.3755369878883,4.3));
#19388=CARTESIAN_POINT('Ctrl Pts',(3.79826159173226,2.3855418166282,4.3));
#19389=CARTESIAN_POINT('Ctrl Pts',(3.79773306912215,2.39555473221079,4.3));
#19390=CARTESIAN_POINT('Ctrl Pts',(3.79647804098653,2.40548740413607,4.3));
#19391=CARTESIAN_POINT('Ctrl Pts',(3.79582247707096,2.41067573507037,4.3));
#19392=CARTESIAN_POINT('Ctrl Pts',(3.79496739950913,2.41584508273998,4.3));
#19393=CARTESIAN_POINT('Ctrl Pts',(3.79391843118089,2.42095777287915,4.3));
#19394=CARTESIAN_POINT('Ctrl Pts',(3.79135148096571,2.43346913351755,4.3));
#19395=CARTESIAN_POINT('Ctrl Pts',(3.78762422716575,2.44567369959671,4.3));
#19396=CARTESIAN_POINT('Ctrl Pts',(3.78275033841106,2.45738291584384,4.3));
#19397=CARTESIAN_POINT('Ctrl Pts',(3.78051276867504,2.46275853872441,4.3));
#19398=CARTESIAN_POINT('Ctrl Pts',(3.77803290925375,2.46802940870032,4.3));
#19399=CARTESIAN_POINT('Ctrl Pts',(3.77530915968311,2.47317482247228,4.3));
#19400=CARTESIAN_POINT('Ctrl Pts',(3.7735285304889,2.4765385950002,4.3));
#19401=CARTESIAN_POINT('Ctrl Pts',(3.77164255910733,2.47985045045176,4.3));
#19402=CARTESIAN_POINT('Ctrl Pts',(3.76965384065618,2.48309856403818,4.3));
#19403=CARTESIAN_POINT('Ctrl Pts',(3.76538142018115,2.49007657894212,4.3));
#19404=CARTESIAN_POINT('Ctrl Pts',(3.76065254798511,2.4967339395313,4.3));
#19405=CARTESIAN_POINT('Ctrl Pts',(3.75546934621649,2.50301830246242,4.3));
#19406=CARTESIAN_POINT('Ctrl Pts',(3.7497639943478,2.5099357452696,4.3));
#19407=CARTESIAN_POINT('Ctrl Pts',(3.74350797317419,2.51640155748529,4.3));
#19408=CARTESIAN_POINT('Ctrl Pts',(3.73677354924283,2.52238273959095,4.3));
#19409=CARTESIAN_POINT('Ctrl Pts',(3.73252952287629,2.52615207380843,4.3));
#19410=CARTESIAN_POINT('Ctrl Pts',(3.72809532803267,2.52972869286917,4.3));
#19411=CARTESIAN_POINT('Ctrl Pts',(3.72348818609076,2.53310156466662,4.3));
#19412=CARTESIAN_POINT('Ctrl Pts',(3.72067461067475,2.53516137295782,4.3));
#19413=CARTESIAN_POINT('Ctrl Pts',(3.71779994290363,2.53714246961825,4.3));
#19414=CARTESIAN_POINT('Ctrl Pts',(3.71487521534485,2.53903869288715,4.3));
#19415=CARTESIAN_POINT('Ctrl Pts',(3.70626340571031,2.54462208945595,4.3));
#19416=CARTESIAN_POINT('Ctrl Pts',(3.69720115342902,2.54948407839451,4.3));
#19417=CARTESIAN_POINT('Ctrl Pts',(3.68779739443943,2.55357358531277,4.3));
#19418=CARTESIAN_POINT('Ctrl Pts',(3.67897143105616,2.55741182046492,4.3));
#19419=CARTESIAN_POINT('Ctrl Pts',(3.66984396791867,2.56056952878093,4.3));
#19420=CARTESIAN_POINT('Ctrl Pts',(3.66050457512214,2.56298263453418,4.3));
#19421=CARTESIAN_POINT('Ctrl Pts',(3.657017355811,2.56388365981129,4.3));
#19422=CARTESIAN_POINT('Ctrl Pts',(3.65350912975721,2.56467838913094,4.3));
#19423=CARTESIAN_POINT('Ctrl Pts',(3.64998789179307,2.5653638764114,4.3));
#19424=CARTESIAN_POINT('Ctrl Pts',(3.63890668202576,2.56752108033372,4.3));
#19425=CARTESIAN_POINT('Ctrl Pts',(3.62768560566387,2.56860271836266,4.3));
#19426=CARTESIAN_POINT('Ctrl Pts',(3.61647526972934,2.56851225659508,4.3));
#19427=CARTESIAN_POINT('Ctrl Pts',(3.61029339424358,2.56846237197194,4.3));
#19428=CARTESIAN_POINT('Ctrl Pts',(3.60411488972487,2.56805522437202,4.3));
#19429=CARTESIAN_POINT('Ctrl Pts',(3.59796731823988,2.56726810386747,4.3));
#19430=CARTESIAN_POINT('Ctrl Pts',(3.5968916538024,2.56713037833848,4.3));
#19431=CARTESIAN_POINT('Ctrl Pts',(3.59581694274575,2.56698100748364,4.3));
#19432=CARTESIAN_POINT('Ctrl Pts',(3.59474333802771,2.56682006235004,4.3));
#19433=CARTESIAN_POINT('Origin',(3.6,2.4,5.35459252805377));
#19434=CARTESIAN_POINT('Ctrl Pts',(3.39434265438876,2.4001499379742,5.17959252805377));
#19435=CARTESIAN_POINT('Ctrl Pts',(3.3942608381295,2.40997903394326,5.17905813053169));
#19436=CARTESIAN_POINT('Ctrl Pts',(3.39937061019979,2.4878631610827,5.17481913665734));
#19437=CARTESIAN_POINT('Ctrl Pts',(3.4989044460774,2.62084298387434,5.16687554643073));
#19438=CARTESIAN_POINT('Ctrl Pts',(3.73070050850364,2.60468899581803,5.15576175737391));
#19439=CARTESIAN_POINT('Ctrl Pts',(3.84286218134804,2.40121305191012,5.14464796831713));
#19440=CARTESIAN_POINT('Ctrl Pts',(3.73273070961532,2.19661070737624,5.1335341792603));
#19441=CARTESIAN_POINT('Ctrl Pts',(3.50110863285869,2.17818091869864,5.12242039020352));
#19442=CARTESIAN_POINT('Ctrl Pts',(3.39978420373419,2.31073763553012,5.11443983980133));
#19443=CARTESIAN_POINT('Ctrl Pts',(3.39427096205728,2.38932589106744,5.11016388575141));
#19444=CARTESIAN_POINT('Ctrl Pts',(3.39436118415265,2.39983962587988,5.10959252805377));
#19445=CARTESIAN_POINT('Ctrl Pts',(3.39473291096846,2.39977036782444,5.18540747194623));
#19446=CARTESIAN_POINT('Ctrl Pts',(3.39508769603641,2.44679019469361,5.18286245525962));
#19447=CARTESIAN_POINT('Ctrl Pts',(3.43434460318779,2.56295297845058,5.17661284222074));
#19448=CARTESIAN_POINT('Ctrl Pts',(3.62721323264599,2.64128528195604,5.16665863282959));
#19449=CARTESIAN_POINT('Ctrl Pts',(3.81747536314189,2.50809334538988,5.15554484377278));
#19450=CARTESIAN_POINT('Ctrl Pts',(3.80876232811303,2.27586209318291,5.14443105471598));
#19451=CARTESIAN_POINT('Ctrl Pts',(3.60892557137656,2.15730570431671,5.13331726565918));
#19452=CARTESIAN_POINT('Ctrl Pts',(3.42787436374214,2.24745398081386,5.12364273806926));
#19453=CARTESIAN_POINT('Ctrl Pts',(3.39500774851697,2.35820797614884,5.11767280683161));
#19454=CARTESIAN_POINT('Ctrl Pts',(3.39479089114249,2.40011619889285,5.11540747194623));
#19455=CARTESIAN_POINT('Ctrl Pts',(3.72690708798524,2.50793586530485,5.2));
#19456=CARTESIAN_POINT('Ctrl Pts',(3.76279833110066,2.46573623930395,5.19629540364773));
#19457=CARTESIAN_POINT('Ctrl Pts',(3.78852074717293,2.34341311981147,5.1888862109432));
#19458=CARTESIAN_POINT('Ctrl Pts',(3.65451258117961,2.21065853310285,5.17777242188639));
#19459=CARTESIAN_POINT('Ctrl Pts',(3.47057722493071,2.25164322990955,5.16665863282959));
#19460=CARTESIAN_POINT('Ctrl Pts',(3.405121385579,2.4282098150683,5.15554484377278));
#19461=CARTESIAN_POINT('Ctrl Pts',(3.5180312968317,2.57906042639477,5.14443105471598));
#19462=CARTESIAN_POINT('Ctrl Pts',(3.70597252569269,2.56596270448124,5.13331726565917));
#19463=CARTESIAN_POINT('Ctrl Pts',(3.79691368493775,2.4009835476249,5.12220347660237));
#19464=CARTESIAN_POINT('Ctrl Pts',(3.70761862135009,2.23509110037173,5.11108968754557));
#19465=CARTESIAN_POINT('Ctrl Pts',(3.51981846080671,2.22014814967852,5.09997589848877));
#19466=CARTESIAN_POINT('Ctrl Pts',(3.40540964822557,2.3698223862213,5.08886210943195));
#19467=CARTESIAN_POINT('Ctrl Pts',(3.46911145369901,2.54712015828428,5.07774832037516));
#19468=CARTESIAN_POINT('Ctrl Pts',(3.65261709875363,2.58975637037653,5.06663453131834));
#19469=CARTESIAN_POINT('Ctrl Pts',(3.78796168225801,2.4587068294695,5.05552074226155));
#19470=CARTESIAN_POINT('Ctrl Pts',(3.75126282351006,2.27392205963726,5.04440695320474));
#19471=CARTESIAN_POINT('Ctrl Pts',(3.576111378403,2.20453795937386,5.03329316414794));
#19472=CARTESIAN_POINT('Ctrl Pts',(3.42282546383512,2.31406243118482,5.02217937509113));
#19473=CARTESIAN_POINT('Ctrl Pts',(3.43170940937961,2.50224655949829,5.01106558603433));
#19474=CARTESIAN_POINT('Ctrl Pts',(3.59463164213028,2.59684323978071,4.99995179697753));
#19475=CARTESIAN_POINT('Ctrl Pts',(3.762467593188,2.51126707661319,4.98883800792072));
#19476=CARTESIAN_POINT('Ctrl Pts',(3.78159511395878,2.32384689323348,4.97772421886391));
#19477=CARTESIAN_POINT('Ctrl Pts',(3.63450656736167,2.20613051367693,4.96661042980712));
#19478=CARTESIAN_POINT('Ctrl Pts',(3.45583376839362,2.26586507280002,4.95549664075031));
#19479=CARTESIAN_POINT('Ctrl Pts',(3.40911795613805,2.44837485237297,4.94438285169351));
#19480=CARTESIAN_POINT('Ctrl Pts',(3.53711864339547,2.58660658076597,4.9332690626367));
#19481=CARTESIAN_POINT('Ctrl Pts',(3.72267534946784,2.5540351896186,4.9221552735799));
#19482=CARTESIAN_POINT('Ctrl Pts',(3.79594591694334,2.38047364248689,4.91104148452309));
#19483=CARTESIAN_POINT('Ctrl Pts',(3.6898649644607,2.22478479185514,4.89992769546629));
#19484=CARTESIAN_POINT('Ctrl Pts',(3.5015295908702,2.22947240830188,4.88881390640948));
#19485=CARTESIAN_POINT('Ctrl Pts',(3.40332529948609,2.39024586335038,4.87770011735268));
#19486=CARTESIAN_POINT('Ctrl Pts',(3.48513959192542,2.5599473902907,4.86658632829587));
#19487=CARTESIAN_POINT('Ctrl Pts',(3.67208691848091,2.58324725697266,4.85547253923907));
#19488=CARTESIAN_POINT('Ctrl Pts',(3.79305227102963,2.43881883118157,4.84435875018227));
#19489=CARTESIAN_POINT('Ctrl Pts',(3.73731469054324,2.25885908897487,4.83324496112546));
#19490=CARTESIAN_POINT('Ctrl Pts',(3.55589141654812,2.20808722327608,4.82213117206866));
#19491=CARTESIAN_POINT('Ctrl Pts',(3.41484122921187,2.33297529855171,4.81101738301186));
#19492=CARTESIAN_POINT('Ctrl Pts',(3.44326896462127,2.51921184317472,4.79990359395504));
#19493=CARTESIAN_POINT('Ctrl Pts',(3.61515439416365,2.59633243578568,4.78878980489825));
#19494=CARTESIAN_POINT('Ctrl Pts',(3.77316883486553,2.49374772336074,4.77767601584144));
#19495=CARTESIAN_POINT('Ctrl Pts',(3.77267987714682,2.30535465657222,4.76656222678464));
#19496=CARTESIAN_POINT('Ctrl Pts',(3.61413506955264,2.20359154597435,4.75544843772783));
#19497=CARTESIAN_POINT('Ctrl Pts',(3.44265227249432,2.28160332076952,4.74433464867103));
#19498=CARTESIAN_POINT('Ctrl Pts',(3.41519163486656,2.46798491877402,4.73322085961423));
#19499=CARTESIAN_POINT('Ctrl Pts',(3.55688818971484,2.59213914962324,4.72210707055742));
#19500=CARTESIAN_POINT('Ctrl Pts',(3.73804547343831,2.54042623781615,4.71099328150061));
#19501=CARTESIAN_POINT('Ctrl Pts',(3.79284816978155,2.36017959799409,4.69987949244381));
#19502=CARTESIAN_POINT('Ctrl Pts',(3.67113474927674,2.2163810237221,4.68876570338701));
#19503=CARTESIAN_POINT('Ctrl Pts',(3.48431088603601,2.24065098081811,4.67765191433021));
#19504=CARTESIAN_POINT('Ctrl Pts',(3.4033785808103,2.41077490231207,4.6665381252734));
#19505=CARTESIAN_POINT('Ctrl Pts',(3.50241609040748,2.57103643352413,4.65542433621659));
#19506=CARTESIAN_POINT('Ctrl Pts',(3.69077325913151,2.57474637744638,4.64431054715979));
#19507=CARTESIAN_POINT('Ctrl Pts',(3.79604463433366,2.41850898033344,4.63319675810299));
#19508=CARTESIAN_POINT('Ctrl Pts',(3.72187413243292,2.24533010361481,4.62208296904618));
#19509=CARTESIAN_POINT('Ctrl Pts',(3.5361508549695,2.21372233713422,4.61096917998938));
#19510=CARTESIAN_POINT('Ctrl Pts',(3.40886942405137,2.35261662800557,4.59985539093258));
#19511=CARTESIAN_POINT('Ctrl Pts',(3.45653197686655,2.53488145663037,4.58874160187577));
#19512=CARTESIAN_POINT('Ctrl Pts',(3.63551243829507,2.5936877583357,4.57762781281897));
#19513=CARTESIAN_POINT('Ctrl Pts',(3.78198796221116,2.47520945827968,4.56651402376216));
#19514=CARTESIAN_POINT('Ctrl Pts',(3.76188784043654,2.28789108810318,4.55540023470536));
#19515=CARTESIAN_POINT('Ctrl Pts',(3.5936099423673,2.20318727643507,4.54428644564855));
#19516=CARTESIAN_POINT('Ctrl Pts',(3.43118093653762,2.29862838255851,4.53317265659175));
#19517=CARTESIAN_POINT('Ctrl Pts',(3.42327393399308,2.4868560799498,4.52205886753494));
#19518=CARTESIAN_POINT('Ctrl Pts',(3.57712630395541,2.59558342196495,4.51094507847815));
#19519=CARTESIAN_POINT('Ctrl Pts',(3.75191522715083,2.52529104055601,4.49983128942133));
#19520=CARTESIAN_POINT('Ctrl Pts',(3.78765442042343,2.34031834729253,4.48871750036454));
#19521=CARTESIAN_POINT('Ctrl Pts',(3.65163139388737,2.20997295066536,4.47760371130772));
#19522=CARTESIAN_POINT('Ctrl Pts',(3.4683495682865,2.25356146118509,4.46648992225093));
#19523=CARTESIAN_POINT('Ctrl Pts',(3.40556887324678,2.431186839349,4.45537613319411));
#19524=CARTESIAN_POINT('Ctrl Pts',(3.52075319873735,2.58026652505992,4.44426234413732));
#19525=CARTESIAN_POINT('Ctrl Pts',(3.70847300970163,2.56434626551467,4.43314855508051));
#19526=CARTESIAN_POINT('Ctrl Pts',(3.79690626562936,2.39799790621595,4.4220347660237));
#19527=CARTESIAN_POINT('Ctrl Pts',(3.7051089416811,2.23348228455085,4.4109209769669));
#19528=CARTESIAN_POINT('Ctrl Pts',(3.51710429525804,2.22138181878176,4.3998071879101));
#19529=CARTESIAN_POINT('Ctrl Pts',(3.40497485954275,2.37277339597561,4.38869339885329));
#19530=CARTESIAN_POINT('Ctrl Pts',(3.47135448294965,2.54908419847293,4.37757960979649));
#19531=CARTESIAN_POINT('Ctrl Pts',(3.65548413352142,2.58893973580292,4.36646582073968));
#19532=CARTESIAN_POINT('Ctrl Pts',(3.78882987626983,2.45585019704184,4.35535203168288));
#19533=CARTESIAN_POINT('Ctrl Pts',(3.7493347906086,2.27165314263956,4.34423824262608));
#19534=CARTESIAN_POINT('Ctrl Pts',(3.57315728718835,2.20490778239848,4.33312445356927));
#19535=CARTESIAN_POINT('Ctrl Pts',(3.4215383866044,2.31678389237007,4.32201066451247));
#19536=CARTESIAN_POINT('Ctrl Pts',(3.43328916816391,2.50472575846861,4.31089687545566));
#19537=CARTESIAN_POINT('Ctrl Pts',(3.59758812791782,2.59701775419156,4.29978308639886));
#19538=CARTESIAN_POINT('Ctrl Pts',(3.76418967154123,2.50855366821667,4.28866929734205));
#19539=CARTESIAN_POINT('Ctrl Pts',(3.77483953817107,2.38400982617006,4.28126010463752));
#19540=CARTESIAN_POINT('Ctrl Pts',(3.75264423560529,2.33325198627316,4.27755550828525));
#19541=CARTESIAN_POINT('Ctrl Pts',(3.73677806246588,2.51633123698097,5.20748149723825));
#19542=CARTESIAN_POINT('Ctrl Pts',(3.77546096639785,2.47084927712496,5.20377690088598));
#19543=CARTESIAN_POINT('Ctrl Pts',(3.80318410060701,2.33901172932062,5.19636770818144));
#19544=CARTESIAN_POINT('Ctrl Pts',(3.658752630386,2.19593134317562,5.18525391912464));
#19545=CARTESIAN_POINT('Ctrl Pts',(3.46051057751011,2.24010387529317,5.17414013006783));
#19546=CARTESIAN_POINT('Ctrl Pts',(3.3899635101576,2.43040400586618,5.16302634101103));
#19547=CARTESIAN_POINT('Ctrl Pts',(3.5116556799136,2.59298794555462,5.15191255195423));
#19548=CARTESIAN_POINT('Ctrl Pts',(3.71421518662967,2.57887146826017,5.14079876289742));
#19549=CARTESIAN_POINT('Ctrl Pts',(3.81222985040785,2.40106004905331,5.12968497384063));
#19550=CARTESIAN_POINT('Ctrl Pts',(3.7159893174385,2.22226430270657,5.11857118478381));
#19551=CARTESIAN_POINT('Ctrl Pts',(3.5135818514907,2.20615907268523,5.10745739572702));
#19552=CARTESIAN_POINT('Ctrl Pts',(3.3902741941935,2.36747513785065,5.0963436066702));
#19553=CARTESIAN_POINT('Ctrl Pts',(3.45893079696141,2.55856332785872,5.08522981761341));
#19554=CARTESIAN_POINT('Ctrl Pts',(3.65670971522832,2.60451583195793,5.07411602855659));
#19555=CARTESIAN_POINT('Ctrl Pts',(3.80258155100106,2.46327311197376,5.0630022394998));
#19556=CARTESIAN_POINT('Ctrl Pts',(3.76302821419424,2.26411557718108,5.05188845044299));
#19557=CARTESIAN_POINT('Ctrl Pts',(3.57425329484041,2.18933470441319,5.04077466138619));
#19558=CARTESIAN_POINT('Ctrl Pts',(3.40904463131529,2.30737811148155,5.02966087232938));
#19559=CARTESIAN_POINT('Ctrl Pts',(3.41861958002714,2.51019941063974,5.01854708327258));
#19560=CARTESIAN_POINT('Ctrl Pts',(3.59421408528317,2.61215392594813,5.00743329421578));
#19561=CARTESIAN_POINT('Ctrl Pts',(3.77510450332242,2.51992155361066,4.99631950515897));
#19562=CARTESIAN_POINT('Ctrl Pts',(3.79571978393707,2.31792361987304,4.98520571610216));
#19563=CARTESIAN_POINT('Ctrl Pts',(3.63719052655772,2.19105112936158,4.97409192704537));
#19564=CARTESIAN_POINT('Ctrl Pts',(3.44462035852227,2.25543190894468,4.96297813798855));
#19565=CARTESIAN_POINT('Ctrl Pts',(3.3942709384207,2.4521375022049,4.95186434893175));
#19566=CARTESIAN_POINT('Ctrl Pts',(3.53222766152672,2.6011210482075,4.94075055987495));
#19567=CARTESIAN_POINT('Ctrl Pts',(3.73221717461903,2.56601621802281,4.92963677081814));
#19568=CARTESIAN_POINT('Ctrl Pts',(3.81118680834224,2.37895486067752,4.91852298176134));
#19569=CARTESIAN_POINT('Ctrl Pts',(3.69685476136628,2.21115635804835,4.90740919270453));
#19570=CARTESIAN_POINT('Ctrl Pts',(3.49387045290517,2.21620858251703,4.89629540364774));
#19571=CARTESIAN_POINT('Ctrl Pts',(3.38802772249033,2.38948717575083,4.88518161459092));
#19572=CARTESIAN_POINT('Ctrl Pts',(3.47620562160949,2.57238827624017,4.87406782553412));
#19573=CARTESIAN_POINT('Ctrl Pts',(3.67769391919309,2.59750043247249,4.86295403647732));
#19574=CARTESIAN_POINT('Ctrl Pts',(3.80806809143035,2.44183820305468,4.85184024742052));
#19575=CARTESIAN_POINT('Ctrl Pts',(3.74799517992873,2.24788099190383,4.84072645836371));
#19576=CARTESIAN_POINT('Ctrl Pts',(3.55246060185887,2.19316003401009,4.82961266930691));
#19577=CARTESIAN_POINT('Ctrl Pts',(3.40043937404102,2.32776204271177,4.8184988802501));
#19578=CARTESIAN_POINT('Ctrl Pts',(3.43107825033486,2.52848427295347,4.8073850911933));
#19579=CARTESIAN_POINT('Ctrl Pts',(3.61633311980013,2.61160339105013,4.79627130213649));
#19580=CARTESIAN_POINT('Ctrl Pts',(3.78663809948217,2.50103952557292,4.78515751307969));
#19581=CARTESIAN_POINT('Ctrl Pts',(3.78611111008816,2.29799303647267,4.77404372402288));
#19582=CARTESIAN_POINT('Ctrl Pts',(3.61523451098693,2.18831467792663,4.76292993496608));
#19583=CARTESIAN_POINT('Ctrl Pts',(3.43041359120824,2.27239429534918,4.75181614590927));
#19584=CARTESIAN_POINT('Ctrl Pts',(3.40081703463734,2.47327286138574,4.74070235685248));
#19585=CARTESIAN_POINT('Ctrl Pts',(3.55353490515134,2.60708394642517,4.72958856779567));
#19586=CARTESIAN_POINT('Ctrl Pts',(3.74878280393034,2.55134874680995,4.71847477873887));
#19587=CARTESIAN_POINT('Ctrl Pts',(3.80784811496013,2.35708232282806,4.70736098968206));
#19588=CARTESIAN_POINT('Ctrl Pts',(3.67666768920898,2.2020989354812,4.69624720062525));
#19589=CARTESIAN_POINT('Ctrl Pts',(3.47531245805411,2.22825663683913,4.68513341156846));
#19590=CARTESIAN_POINT('Ctrl Pts',(3.38808514809522,2.41161298620039,4.67401962251165));
#19591=CARTESIAN_POINT('Ctrl Pts',(3.49482590536264,2.58433983759226,4.66290583345484));
#19592=CARTESIAN_POINT('Ctrl Pts',(3.69783370420702,2.58833834507989,4.65179204439804));
#19593=CARTESIAN_POINT('Ctrl Pts',(3.811293204081,2.419948629414,4.64067825534124));
#19594=CARTESIAN_POINT('Ctrl Pts',(3.73135363803182,2.23329970701222,4.62956446628443));
#19595=CARTESIAN_POINT('Ctrl Pts',(3.53118459744037,2.19923345329287,4.61845067722763));
#19596=CARTESIAN_POINT('Ctrl Pts',(3.39400307523184,2.34893109662045,4.60733688817082));
#19597=CARTESIAN_POINT('Ctrl Pts',(3.44537287442694,2.54537268637529,4.59622309911402));
#19598=CARTESIAN_POINT('Ctrl Pts',(3.6382746352513,2.60875300764603,4.58510931005721));
#19599=CARTESIAN_POINT('Ctrl Pts',(3.79614318836354,2.48105933361106,4.57399552100041));
#19600=CARTESIAN_POINT('Ctrl Pts',(3.77447965675701,2.27917113222085,4.56288173194361));
#19601=CARTESIAN_POINT('Ctrl Pts',(3.59311291657604,2.18787896385287,4.5517679428868));
#19602=CARTESIAN_POINT('Ctrl Pts',(3.4180500019796,2.29074358538356,4.54065415383));
#19603=CARTESIAN_POINT('Ctrl Pts',(3.40952798398103,2.4936118424709,4.5295403647732));
#19604=CARTESIAN_POINT('Ctrl Pts',(3.57534716243134,2.61079611810118,4.51842657571639));
#19605=CARTESIAN_POINT('Ctrl Pts',(3.76373136251596,2.53503631706984,4.50731278665959));
#19606=CARTESIAN_POINT('Ctrl Pts',(3.80225038999918,2.33567624195239,4.49619899760278));
#19607=CARTESIAN_POINT('Ctrl Pts',(3.65564734114102,2.19519243537347,4.48508520854597));
#19608=CARTESIAN_POINT('Ctrl Pts',(3.45810965125396,2.24217130873125,4.47397141948918));
#19609=CARTESIAN_POINT('Ctrl Pts',(3.39044580391398,2.4336125864072,4.46285763043236));
#19610=CARTESIAN_POINT('Ctrl Pts',(3.51458929437743,2.59428785591567,4.45174384137557));
#19611=CARTESIAN_POINT('Ctrl Pts',(3.71691016106647,2.57712930087258,4.44063005231875));
#19612=CARTESIAN_POINT('Ctrl Pts',(3.8122218540174,2.39784218113421,4.42951626326196));
#19613=CARTESIAN_POINT('Ctrl Pts',(3.71328443209297,2.22053035140142,4.41840247420515));
#19614=CARTESIAN_POINT('Ctrl Pts',(3.5106565751263,2.2074886979437,4.40728868514835));
#19615=CARTESIAN_POINT('Ctrl Pts',(3.38980558716325,2.3706556804265,4.39617489609155));
#19616=CARTESIAN_POINT('Ctrl Pts',(3.46134829152241,2.56068013327812,4.38506110703473));
#19617=CARTESIAN_POINT('Ctrl Pts',(3.65979975114976,2.60363567863874,4.37394731797794));
#19618=CARTESIAN_POINT('Ctrl Pts',(3.80351727410895,2.46019428749802,4.36283352892113));
#19619=CARTESIAN_POINT('Ctrl Pts',(3.76095021674888,2.26167018129524,4.35171973986433));
#19620=CARTESIAN_POINT('Ctrl Pts',(3.57106943112482,2.18973329268408,4.34060595080752));
#19621=CARTESIAN_POINT('Ctrl Pts',(3.40765744378577,2.31031125094527,4.32949216175072));
#19622=CARTESIAN_POINT('Ctrl Pts',(3.42032221420706,2.51287144446394,4.31837837269392));
#19623=CARTESIAN_POINT('Ctrl Pts',(3.5974005298242,2.61234201428399,4.30726458363711));
#19624=CARTESIAN_POINT('Ctrl Pts',(3.77696052684568,2.51699709329055,4.29615079458031));
#19625=CARTESIAN_POINT('Ctrl Pts',(3.78843875194939,2.38276609266138,4.28874160187577));
#19626=CARTESIAN_POINT('Ctrl Pts',(3.76451707405898,2.328060251512,4.2850370055235));
#19627=CARTESIAN_POINT('Ctrl Pts',(3.74664903694653,2.52472660865709,5.2149629944765));
#19628=CARTESIAN_POINT('Ctrl Pts',(3.78812360169505,2.47596231494597,5.21125839812423));
#19629=CARTESIAN_POINT('Ctrl Pts',(3.81784745404107,2.33461033882977,5.20384920541969));
#19630=CARTESIAN_POINT('Ctrl Pts',(3.66299267959241,2.1812041532484,5.19273541636289));
#19631=CARTESIAN_POINT('Ctrl Pts',(3.4504439300895,2.22856452067679,5.18162162730609));
#19632=CARTESIAN_POINT('Ctrl Pts',(3.3748056347362,2.43259819666406,5.17050783824928));
#19633=CARTESIAN_POINT('Ctrl Pts',(3.5052800629955,2.60691546471448,5.15939404919248));
#19634=CARTESIAN_POINT('Ctrl Pts',(3.72245784756665,2.5917802320391,5.14828026013567));
#19635=CARTESIAN_POINT('Ctrl Pts',(3.82754601587795,2.40113655048171,5.13716647107887));
#19636=CARTESIAN_POINT('Ctrl Pts',(3.72436001352691,2.2094375050414,5.12605268202206));
#19637=CARTESIAN_POINT('Ctrl Pts',(3.5073452421747,2.19216999569193,5.11493889296526));
#19638=CARTESIAN_POINT('Ctrl Pts',(3.37513874016143,2.36512788948001,5.10382510390846));
#19639=CARTESIAN_POINT('Ctrl Pts',(3.44875014022381,2.57000649743315,5.09271131485165));
#19640=CARTESIAN_POINT('Ctrl Pts',(3.660802331703,2.61927529353934,5.08159752579485));
#19641=CARTESIAN_POINT('Ctrl Pts',(3.81720141974412,2.46783939447801,5.07048373673805));
#19642=CARTESIAN_POINT('Ctrl Pts',(3.77479360487843,2.25430909472489,5.05936994768124));
#19643=CARTESIAN_POINT('Ctrl Pts',(3.57239521127782,2.17413144945252,5.04825615862444));
#19644=CARTESIAN_POINT('Ctrl Pts',(3.39526379879546,2.30069379177829,5.03714236956763));
#19645=CARTESIAN_POINT('Ctrl Pts',(3.40552975067466,2.51815226178119,5.02602858051083));
#19646=CARTESIAN_POINT('Ctrl Pts',(3.59379652843607,2.62746461211554,5.01491479145402));
#19647=CARTESIAN_POINT('Ctrl Pts',(3.78774141345684,2.52857603060814,5.00380100239722));
#19648=CARTESIAN_POINT('Ctrl Pts',(3.80984445391536,2.3120003465126,4.99268721334041));
#19649=CARTESIAN_POINT('Ctrl Pts',(3.63987448575377,2.17597174504624,4.98157342428361));
#19650=CARTESIAN_POINT('Ctrl Pts',(3.43340694865093,2.24499874508934,4.9704596352268));
#19651=CARTESIAN_POINT('Ctrl Pts',(3.37942392070334,2.45590015203683,4.95934584617001));
#19652=CARTESIAN_POINT('Ctrl Pts',(3.52733667965797,2.61563551564903,4.94823205711319));
#19653=CARTESIAN_POINT('Ctrl Pts',(3.74175899977021,2.57799724642702,4.9371182680564));
#19654=CARTESIAN_POINT('Ctrl Pts',(3.82642769974115,2.37743607886815,4.92600447899959));
#19655=CARTESIAN_POINT('Ctrl Pts',(3.70384455827186,2.19752792424157,4.91489068994279));
#19656=CARTESIAN_POINT('Ctrl Pts',(3.48621131494014,2.20294475673219,4.90377690088598));
#19657=CARTESIAN_POINT('Ctrl Pts',(3.37273014549458,2.38872848815129,4.89266311182918));
#19658=CARTESIAN_POINT('Ctrl Pts',(3.46727165129357,2.58482916218966,4.88154932277237));
#19659=CARTESIAN_POINT('Ctrl Pts',(3.68330091990526,2.61175360797231,4.87043553371557));
#19660=CARTESIAN_POINT('Ctrl Pts',(3.82308391183106,2.4448575749278,4.85932174465876));
#19661=CARTESIAN_POINT('Ctrl Pts',(3.75867566931422,2.2369028948328,4.84820795560196));
#19662=CARTESIAN_POINT('Ctrl Pts',(3.54902978716961,2.1782328447441,4.83709416654516));
#19663=CARTESIAN_POINT('Ctrl Pts',(3.38603751887018,2.32254878687183,4.82598037748835));
#19664=CARTESIAN_POINT('Ctrl Pts',(3.41888753604845,2.53775670273222,4.81486658843155));
#19665=CARTESIAN_POINT('Ctrl Pts',(3.61751184543661,2.62687434631457,4.80375279937474));
#19666=CARTESIAN_POINT('Ctrl Pts',(3.80010736409881,2.5083313277851,4.79263901031794));
#19667=CARTESIAN_POINT('Ctrl Pts',(3.79954234302951,2.29063141637312,4.78152522126113));
#19668=CARTESIAN_POINT('Ctrl Pts',(3.61633395242122,2.17303780987892,4.77041143220434));
#19669=CARTESIAN_POINT('Ctrl Pts',(3.41817490992216,2.26318526992884,4.75929764314752));
#19670=CARTESIAN_POINT('Ctrl Pts',(3.38644243440813,2.47856080399747,4.74818385409073));
#19671=CARTESIAN_POINT('Ctrl Pts',(3.55018162058784,2.62202874322709,4.73707006503392));
#19672=CARTESIAN_POINT('Ctrl Pts',(3.75952013442236,2.56227125580376,4.72595627597711));
#19673=CARTESIAN_POINT('Ctrl Pts',(3.82284806013872,2.35398504766203,4.71484248692031));
#19674=CARTESIAN_POINT('Ctrl Pts',(3.68220062914122,2.1878168472403,4.7037286978635));
#19675=CARTESIAN_POINT('Ctrl Pts',(3.46631403007222,2.21586229286015,4.6926149088067));
#19676=CARTESIAN_POINT('Ctrl Pts',(3.37279171538014,2.4124510700887,4.6815011197499));
#19677=CARTESIAN_POINT('Ctrl Pts',(3.48723572031781,2.59764324166039,4.67038733069309));
#19678=CARTESIAN_POINT('Ctrl Pts',(3.70489414928252,2.6019303127134,4.65927354163629));
#19679=CARTESIAN_POINT('Ctrl Pts',(3.82654177382834,2.42138827849455,4.64815975257948));
#19680=CARTESIAN_POINT('Ctrl Pts',(3.74083314363071,2.22126931040964,4.63704596352268));
#19681=CARTESIAN_POINT('Ctrl Pts',(3.52621833991124,2.18474456945152,4.62593217446588));
#19682=CARTESIAN_POINT('Ctrl Pts',(3.3791367264123,2.34524556523533,4.61481838540907));
#19683=CARTESIAN_POINT('Ctrl Pts',(3.43421377198734,2.55586391612019,4.60370459635226));
#19684=CARTESIAN_POINT('Ctrl Pts',(3.64103683220752,2.62381825695636,4.59259080729547));
#19685=CARTESIAN_POINT('Ctrl Pts',(3.81029841451592,2.48690920894243,4.58147701823866));
#19686=CARTESIAN_POINT('Ctrl Pts',(3.78707147307748,2.27045117633852,4.57036322918186));
#19687=CARTESIAN_POINT('Ctrl Pts',(3.59261589078479,2.17257065127066,4.55924944012505));
#19688=CARTESIAN_POINT('Ctrl Pts',(3.40491906742157,2.28285878820862,4.54813565106825));
#19689=CARTESIAN_POINT('Ctrl Pts',(3.39578203396899,2.500367604992,4.53702186201145));
#19690=CARTESIAN_POINT('Ctrl Pts',(3.57356802090726,2.62600881423741,4.52590807295463));
#19691=CARTESIAN_POINT('Ctrl Pts',(3.77554749788108,2.54478159358368,4.51479428389784));
#19692=CARTESIAN_POINT('Ctrl Pts',(3.81684635957493,2.33103413661225,4.50368049484102));
#19693=CARTESIAN_POINT('Ctrl Pts',(3.65966328839466,2.18041192008159,4.49256670578423));
#19694=CARTESIAN_POINT('Ctrl Pts',(3.44786973422143,2.23078115627741,4.48145291672742));
#19695=CARTESIAN_POINT('Ctrl Pts',(3.37532273458119,2.43603833346541,4.47033912767062));
#19696=CARTESIAN_POINT('Ctrl Pts',(3.50842539001751,2.60830918677142,4.45922533861381));
#19697=CARTESIAN_POINT('Ctrl Pts',(3.72534731243133,2.58991233623048,4.44811154955701));
#19698=CARTESIAN_POINT('Ctrl Pts',(3.82753744240543,2.39768645605247,4.4369977605002));
#19699=CARTESIAN_POINT('Ctrl Pts',(3.72145992250484,2.20757841825199,4.4258839714434));
#19700=CARTESIAN_POINT('Ctrl Pts',(3.50420885499455,2.19359557710565,4.41477018238659));
#19701=CARTESIAN_POINT('Ctrl Pts',(3.37463631478375,2.36853796487738,4.40365639332979));
#19702=CARTESIAN_POINT('Ctrl Pts',(3.45134210009517,2.57227606808331,4.39254260427299));
#19703=CARTESIAN_POINT('Ctrl Pts',(3.6641153687781,2.61833162147455,4.38142881521619));
#19704=CARTESIAN_POINT('Ctrl Pts',(3.81820467194806,2.46453837795421,4.37031502615938));
#19705=CARTESIAN_POINT('Ctrl Pts',(3.77256564288916,2.25168721995093,4.35920123710258));
#19706=CARTESIAN_POINT('Ctrl Pts',(3.56898157506129,2.17455880296967,4.34808744804577));
#19707=CARTESIAN_POINT('Ctrl Pts',(3.39377650096713,2.30383860952047,4.33697365898897));
#19708=CARTESIAN_POINT('Ctrl Pts',(3.40735526025023,2.52101713045927,4.32585986993216));
#19709=CARTESIAN_POINT('Ctrl Pts',(3.59721293173057,2.62766627437643,4.31474608087536));
#19710=CARTESIAN_POINT('Ctrl Pts',(3.78973138215013,2.52544051836443,4.30363229181856));
#19711=CARTESIAN_POINT('Ctrl Pts',(3.8020379657277,2.3815223591527,4.29622309911402));
#19712=CARTESIAN_POINT('Ctrl Pts',(3.77638991251267,2.32286851675083,4.29251850276175));
#19713=CARTESIAN_POINT('Ctrl Pts',(3.75652001142717,2.53312198033322,5.22244449171475));
#19714=CARTESIAN_POINT('Ctrl Pts',(3.80078623699225,2.48107535276698,5.21873989536248));
#19715=CARTESIAN_POINT('Ctrl Pts',(3.83251080747514,2.33020894833891,5.21133070265794));
#19716=CARTESIAN_POINT('Ctrl Pts',(3.6672327287988,2.16647696332117,5.20021691360114));
#19717=CARTESIAN_POINT('Ctrl Pts',(3.44037728266889,2.21702516606042,5.18910312454433));
#19718=CARTESIAN_POINT('Ctrl Pts',(3.3596477593148,2.43479238746194,5.17798933548753));
#19719=CARTESIAN_POINT('Ctrl Pts',(3.4989044460774,2.62084298387434,5.16687554643073));
#19720=CARTESIAN_POINT('Ctrl Pts',(3.73070050850364,2.60468899581803,5.15576175737391));
#19721=CARTESIAN_POINT('Ctrl Pts',(3.84286218134804,2.40121305191012,5.14464796831713));
#19722=CARTESIAN_POINT('Ctrl Pts',(3.73273070961532,2.19661070737624,5.1335341792603));
#19723=CARTESIAN_POINT('Ctrl Pts',(3.50110863285869,2.17818091869864,5.12242039020352));
#19724=CARTESIAN_POINT('Ctrl Pts',(3.36000328612935,2.36278064110937,5.1113066011467));
#19725=CARTESIAN_POINT('Ctrl Pts',(3.43856948348621,2.58144966700758,5.10019281208991));
#19726=CARTESIAN_POINT('Ctrl Pts',(3.66489494817768,2.63403475512075,5.08907902303309));
#19727=CARTESIAN_POINT('Ctrl Pts',(3.83182128848718,2.47240567698227,5.0779652339763));
#19728=CARTESIAN_POINT('Ctrl Pts',(3.78655899556261,2.24450261226871,5.06685144491949));
#19729=CARTESIAN_POINT('Ctrl Pts',(3.57053712771522,2.15892819449186,5.05573765586269));
#19730=CARTESIAN_POINT('Ctrl Pts',(3.38148296627563,2.29400947207503,5.04462386680588));
#19731=CARTESIAN_POINT('Ctrl Pts',(3.39243992132218,2.52610511292264,5.03351007774908));
#19732=CARTESIAN_POINT('Ctrl Pts',(3.59337897158896,2.64277529828296,5.02239628869227));
#19733=CARTESIAN_POINT('Ctrl Pts',(3.80037832359127,2.53723050760561,5.01128249963547));
#19734=CARTESIAN_POINT('Ctrl Pts',(3.82396912389365,2.30607707315216,5.00016871057866));
#19735=CARTESIAN_POINT('Ctrl Pts',(3.64255844494981,2.16089236073089,4.98905492152186));
#19736=CARTESIAN_POINT('Ctrl Pts',(3.42219353877959,2.234565581234,4.97794113246505));
#19737=CARTESIAN_POINT('Ctrl Pts',(3.36457690298599,2.45966280186876,4.96682734340826));
#19738=CARTESIAN_POINT('Ctrl Pts',(3.52244569778922,2.63014998309056,4.95571355435144));
#19739=CARTESIAN_POINT('Ctrl Pts',(3.7513008249214,2.58997827483123,4.94459976529465));
#19740=CARTESIAN_POINT('Ctrl Pts',(3.84166859114005,2.37591729705878,4.93348597623783));
#19741=CARTESIAN_POINT('Ctrl Pts',(3.71083435517744,2.18389949043478,4.92237218718104));
#19742=CARTESIAN_POINT('Ctrl Pts',(3.47855217697512,2.18968093094735,4.91125839812423));
#19743=CARTESIAN_POINT('Ctrl Pts',(3.35743256849882,2.38796980055174,4.90014460906743));
#19744=CARTESIAN_POINT('Ctrl Pts',(3.45833768097764,2.59727004813914,4.88903082001062));
#19745=CARTESIAN_POINT('Ctrl Pts',(3.68890792061744,2.62600678347214,4.87791703095382));
#19746=CARTESIAN_POINT('Ctrl Pts',(3.83809973223177,2.44787694680091,4.86680324189701));
#19747=CARTESIAN_POINT('Ctrl Pts',(3.76935615869971,2.22592479776177,4.85568945284022));
#19748=CARTESIAN_POINT('Ctrl Pts',(3.54559897248035,2.16330565547811,4.8445756637834));
#19749=CARTESIAN_POINT('Ctrl Pts',(3.37163566369933,2.31733553103189,4.83346187472661));
#19750=CARTESIAN_POINT('Ctrl Pts',(3.40669682176204,2.54702913251096,4.82234808566979));
#19751=CARTESIAN_POINT('Ctrl Pts',(3.61869057107309,2.64214530157901,4.811234296613));
#19752=CARTESIAN_POINT('Ctrl Pts',(3.81357662871545,2.51562312999728,4.80012050755618));
#19753=CARTESIAN_POINT('Ctrl Pts',(3.81297357597085,2.28326979627357,4.78900671849939));
#19754=CARTESIAN_POINT('Ctrl Pts',(3.61743339385551,2.1577609418312,4.77789292944258));
#19755=CARTESIAN_POINT('Ctrl Pts',(3.40593622863608,2.2539762445085,4.76677914038578));
#19756=CARTESIAN_POINT('Ctrl Pts',(3.37206783417891,2.48384874660919,4.75566535132897));
#19757=CARTESIAN_POINT('Ctrl Pts',(3.54682833602434,2.63697354002902,4.74455156227216));
#19758=CARTESIAN_POINT('Ctrl Pts',(3.77025746491439,2.57319376479756,4.73343777321537));
#19759=CARTESIAN_POINT('Ctrl Pts',(3.83784800531731,2.35088777249601,4.72232398415856));
#19760=CARTESIAN_POINT('Ctrl Pts',(3.68773356907346,2.1735347589994,4.71121019510175));
#19761=CARTESIAN_POINT('Ctrl Pts',(3.45731560209032,2.20346794888116,4.70009640604495));
#19762=CARTESIAN_POINT('Ctrl Pts',(3.35749828266505,2.41328915397702,4.68898261698814));
#19763=CARTESIAN_POINT('Ctrl Pts',(3.47964553527297,2.61094664572852,4.67786882793135));
#19764=CARTESIAN_POINT('Ctrl Pts',(3.71195459435803,2.61552228034691,4.66675503887453));
#19765=CARTESIAN_POINT('Ctrl Pts',(3.84179034357568,2.42282792757511,4.65564124981774));
#19766=CARTESIAN_POINT('Ctrl Pts',(3.75031264922961,2.20923891380705,4.64452746076093));
#19767=CARTESIAN_POINT('Ctrl Pts',(3.5212520823821,2.17025568561017,4.63341367170412));
#19768=CARTESIAN_POINT('Ctrl Pts',(3.36427037759277,2.34156003385021,4.62229988264733));
#19769=CARTESIAN_POINT('Ctrl Pts',(3.42305466954774,2.56635514586511,4.61118609359051));
#19770=CARTESIAN_POINT('Ctrl Pts',(3.64379902916374,2.63888350626668,4.60007230453372));
#19771=CARTESIAN_POINT('Ctrl Pts',(3.8244536406683,2.49275908427381,4.5889585154769));
#19772=CARTESIAN_POINT('Ctrl Pts',(3.79966328939795,2.26173122045618,4.57784472642011));
#19773=CARTESIAN_POINT('Ctrl Pts',(3.59211886499353,2.15726233868846,4.56673093736329));
#19774=CARTESIAN_POINT('Ctrl Pts',(3.39178813286355,2.27497399103367,4.55561714830651));
#19775=CARTESIAN_POINT('Ctrl Pts',(3.38203608395695,2.50712336751311,4.54450335924968));
#19776=CARTESIAN_POINT('Ctrl Pts',(3.57178887938318,2.64122151037363,4.5333895701929));
#19777=CARTESIAN_POINT('Ctrl Pts',(3.78736363324621,2.55452687009752,4.52227578113608));
#19778=CARTESIAN_POINT('Ctrl Pts',(3.83144232915068,2.3263920312721,4.51116199207928));
#19779=CARTESIAN_POINT('Ctrl Pts',(3.66367923564831,2.1656314047897,4.50004820302247));
#19780=CARTESIAN_POINT('Ctrl Pts',(3.43762981718889,2.21939100382357,4.48893441396567));
#19781=CARTESIAN_POINT('Ctrl Pts',(3.36019966524839,2.43846408052362,4.47782062490886));
#19782=CARTESIAN_POINT('Ctrl Pts',(3.5022614856576,2.62233051762717,4.46670683585207));
#19783=CARTESIAN_POINT('Ctrl Pts',(3.73378446379617,2.60269537158839,4.45559304679526));
#19784=CARTESIAN_POINT('Ctrl Pts',(3.84285303079348,2.39753073097072,4.44447925773845));
#19785=CARTESIAN_POINT('Ctrl Pts',(3.72963541291671,2.19462648510256,4.43336546868165));
#19786=CARTESIAN_POINT('Ctrl Pts',(3.49776113486282,2.17970245626759,4.42225167962485));
#19787=CARTESIAN_POINT('Ctrl Pts',(3.35946704240424,2.36642024932827,4.41113789056804));
#19788=CARTESIAN_POINT('Ctrl Pts',(3.44133590866794,2.5838720028885,4.40002410151124));
#19789=CARTESIAN_POINT('Ctrl Pts',(3.66843098640644,2.63302756431036,4.38891031245443));
#19790=CARTESIAN_POINT('Ctrl Pts',(3.83289206978718,2.4688824684104,4.37779652339763));
#19791=CARTESIAN_POINT('Ctrl Pts',(3.78418106902943,2.24170425860662,4.36668273434082));
#19792=CARTESIAN_POINT('Ctrl Pts',(3.56689371899776,2.15938431325527,4.35556894528402));
#19793=CARTESIAN_POINT('Ctrl Pts',(3.37989555814849,2.29736596809567,4.34445515622721));
#19794=CARTESIAN_POINT('Ctrl Pts',(3.39438830629339,2.5291628164546,4.33334136717041));
#19795=CARTESIAN_POINT('Ctrl Pts',(3.59702533363695,2.64299053446886,4.32222757811361));
#19796=CARTESIAN_POINT('Ctrl Pts',(3.80250223745458,2.5338839434383,4.3111137890568));
#19797=CARTESIAN_POINT('Ctrl Pts',(3.81563717950601,2.38027862564402,4.30370459635227));
#19798=CARTESIAN_POINT('Ctrl Pts',(3.78826275096636,2.31767678198967,4.3));
#19799=CARTESIAN_POINT('Ctrl Pts',(3.72690708798524,2.50793586530485,5.2));
#19800=CARTESIAN_POINT('Ctrl Pts',(3.7351188943469,2.50027512151453,5.2));
#19801=CARTESIAN_POINT('Ctrl Pts',(3.74243605781657,2.49177396851828,5.2));
#19802=CARTESIAN_POINT('Ctrl Pts',(3.74885415042291,2.48262661237479,5.2));
#19803=CARTESIAN_POINT('Ctrl Pts',(3.75362491760652,2.47582709900174,5.2));
#19804=CARTESIAN_POINT('Ctrl Pts',(3.75789857135109,2.46866923842676,5.2));
#19805=CARTESIAN_POINT('Ctrl Pts',(3.7616631109362,2.46121836915243,5.2));
#19806=CARTESIAN_POINT('Ctrl Pts',(3.76388040997986,2.45682983638691,5.2));
#19807=CARTESIAN_POINT('Ctrl Pts',(3.76592247954252,2.45233444011456,5.2));
#19808=CARTESIAN_POINT('Ctrl Pts',(3.76777440855395,2.44777396604178,5.2));
#19809=CARTESIAN_POINT('Ctrl Pts',(3.77233273486399,2.43654884411541,5.2));
#19810=CARTESIAN_POINT('Ctrl Pts',(3.77575805024602,2.42490557824884,5.2));
#19811=CARTESIAN_POINT('Ctrl Pts',(3.77802226640697,2.41304266545579,5.2));
#19812=CARTESIAN_POINT('Ctrl Pts',(3.7794611438358,2.4055039517268,5.2));
#19813=CARTESIAN_POINT('Ctrl Pts',(3.78043038990374,2.39787565429666,5.2));
#19814=CARTESIAN_POINT('Ctrl Pts',(3.78091323142362,2.39020359559663,5.2));
#19815=CARTESIAN_POINT('Ctrl Pts',(3.78113855699256,2.38662330906275,5.2));
#19816=CARTESIAN_POINT('Ctrl Pts',(3.78125741264451,2.38303694149785,5.2));
#19817=CARTESIAN_POINT('Ctrl Pts',(3.78126865224829,2.37945929304311,5.2));
#19818=CARTESIAN_POINT('Ctrl Pts',(3.7813036985799,2.36830378822358,5.2));
#19819=CARTESIAN_POINT('Ctrl Pts',(3.78029680360483,2.3572059009501,5.2));
#19820=CARTESIAN_POINT('Ctrl Pts',(3.77821424861763,2.34630678216484,5.2));
#19821=CARTESIAN_POINT('Ctrl Pts',(3.77705386628862,2.34023388376937,5.2));
#19822=CARTESIAN_POINT('Ctrl Pts',(3.77555898983988,2.33422245704814,5.2));
#19823=CARTESIAN_POINT('Ctrl Pts',(3.77374834890996,2.32828864283844,5.2));
#19824=CARTESIAN_POINT('Ctrl Pts',(3.7726157055599,2.32457675546527,5.2));
#19825=CARTESIAN_POINT('Ctrl Pts',(3.77135884755536,2.32089372066286,5.2));
#19826=CARTESIAN_POINT('Ctrl Pts',(3.76998347568685,2.31724835341447,5.2));
#19827=CARTESIAN_POINT('Ctrl Pts',(3.76560168937412,2.30563460684914,5.2));
#19828=CARTESIAN_POINT('Ctrl Pts',(3.76005258957863,2.29448378034876,5.2));
#19829=CARTESIAN_POINT('Ctrl Pts',(3.75350159415067,2.28391841534468,5.2));
#19830=CARTESIAN_POINT('Ctrl Pts',(3.74916061754095,2.27691734155978,5.2));
#19831=CARTESIAN_POINT('Ctrl Pts',(3.74437851970176,2.27017319623005,5.2));
#19832=CARTESIAN_POINT('Ctrl Pts',(3.73919188354146,2.26372385230471,5.2));
#19833=CARTESIAN_POINT('Ctrl Pts',(3.73648175856153,2.26035393632525,5.2));
#19834=CARTESIAN_POINT('Ctrl Pts',(3.73365978483958,2.25706319070089,5.2));
#19835=CARTESIAN_POINT('Ctrl Pts',(3.73073434111394,2.25386182215374,5.2));
#19836=CARTESIAN_POINT('Ctrl Pts',(3.72446791350779,2.24700435158764,5.2));
#19837=CARTESIAN_POINT('Ctrl Pts',(3.71775194552741,2.24058263588329,5.2));
#19838=CARTESIAN_POINT('Ctrl Pts',(3.71064052052299,2.23464742809312,5.2));
#19839=CARTESIAN_POINT('Ctrl Pts',(3.70611387191905,2.23086947922341,5.2));
#19840=CARTESIAN_POINT('Ctrl Pts',(3.70142674452504,2.22728872352275,5.2));
#19841=CARTESIAN_POINT('Ctrl Pts',(3.69659089091882,2.22391966825811,5.2));
#19842=CARTESIAN_POINT('Ctrl Pts',(3.69251851777989,2.22108251658222,5.2));
#19843=CARTESIAN_POINT('Ctrl Pts',(3.68834767342073,2.21840053637087,5.2));
#19844=CARTESIAN_POINT('Ctrl Pts',(3.68408917108174,2.21588334611703,5.2));
#19845=CARTESIAN_POINT('Ctrl Pts',(3.67536611602187,2.21072716973562,5.2));
#19846=CARTESIAN_POINT('Ctrl Pts',(3.66627202526677,2.20625880103906,5.2));
#19847=CARTESIAN_POINT('Ctrl Pts',(3.65686566645047,2.20255201748434,5.2));
#19848=CARTESIAN_POINT('Ctrl Pts',(3.65562635833217,2.2020636407339,5.2));
#19849=CARTESIAN_POINT('Ctrl Pts',(3.65438161447105,2.20158850411268,5.2));
#19850=CARTESIAN_POINT('Ctrl Pts',(3.65313162618094,2.20112654952031,5.2));
#19851=CARTESIAN_POINT('Ctrl Pts',(3.43326717741735,2.39986996798437,5.08714803633902));
#19852=CARTESIAN_POINT('Ctrl Pts',(3.43319402496042,2.39134538728232,5.08771939403666));
#19853=CARTESIAN_POINT('Ctrl Pts',(3.43379133263065,2.38283109195966,5.08829075173431));
#19854=CARTESIAN_POINT('Ctrl Pts',(3.43509475123467,2.374426308808,5.08886210943196));
#19855=CARTESIAN_POINT('Ctrl Pts',(3.44354591908595,2.31993097404037,5.09256670578422));
#19856=CARTESIAN_POINT('Ctrl Pts',(3.48168218994633,2.27003956185944,5.0962713021365));
#19857=CARTESIAN_POINT('Ctrl Pts',(3.53205035213375,2.24758434755118,5.09997589848876));
#19858=CARTESIAN_POINT('Ctrl Pts',(3.58241851432117,2.22512913324292,5.10368049484103));
#19859=CARTESIAN_POINT('Ctrl Pts',(3.64501856783563,2.23011011680733,5.1073850911933));
#19860=CARTESIAN_POINT('Ctrl Pts',(3.69120110519081,2.26024934979839,5.11108968754557));
#19861=CARTESIAN_POINT('Ctrl Pts',(3.73738364254598,2.29038858278945,5.11479428389783));
#19862=CARTESIAN_POINT('Ctrl Pts',(3.76714866374187,2.34568606520718,5.1184988802501));
#19863=CARTESIAN_POINT('Ctrl Pts',(3.76687431446563,2.40083133255876,5.12220347660237));
#19864=CARTESIAN_POINT('Ctrl Pts',(3.7665999651894,2.45597659991035,5.12590807295464));
#19865=CARTESIAN_POINT('Ctrl Pts',(3.73628624544104,2.51096965219579,5.12961266930691));
#19866=CARTESIAN_POINT('Ctrl Pts',(3.68980584742337,2.54064913199077,5.13331726565917));
#19867=CARTESIAN_POINT('Ctrl Pts',(3.6433254494057,2.57032861178575,5.13702186201144));
#19868=CARTESIAN_POINT('Ctrl Pts',(3.5806783731187,2.57469451909026,5.14072645836371));
#19869=CARTESIAN_POINT('Ctrl Pts',(3.53053651643308,2.5517357041881,5.14443105471598));
#19870=CARTESIAN_POINT('Ctrl Pts',(3.48039465974747,2.52877688928595,5.14813565106825));
#19871=CARTESIAN_POINT('Ctrl Pts',(3.44275802266323,2.47849335217712,5.15184024742051));
#19872=CARTESIAN_POINT('Ctrl Pts',(3.43484901067973,2.42392381942959,5.15554484377278));
#19873=CARTESIAN_POINT('Ctrl Pts',(3.43370811542309,2.41605202441919,5.15607924129486));
#19874=CARTESIAN_POINT('Ctrl Pts',(3.43318581643692,2.40809104297335,5.15661363881694));
#19875=CARTESIAN_POINT('Ctrl Pts',(3.43325215340634,2.40012157034435,5.15714803633902));
#19876=CARTESIAN_POINT('Ctrl Pts',(3.54698297828114,2.20148256743283,5.2));
#19877=CARTESIAN_POINT('Ctrl Pts',(3.48097120902544,2.21911198848201,5.19629540364773));
#19878=CARTESIAN_POINT('Ctrl Pts',(3.36906718698604,2.32515231990061,5.1888862109432));
#19879=CARTESIAN_POINT('Ctrl Pts',(3.41187706889408,2.55382793971174,5.17777242188639));
#19880=CARTESIAN_POINT('Ctrl Pts',(3.62721323264599,2.64128528195604,5.16665863282959));
#19881=CARTESIAN_POINT('Ctrl Pts',(3.81747536314189,2.50809334538988,5.15554484377278));
#19882=CARTESIAN_POINT('Ctrl Pts',(3.80876232811303,2.27586209318291,5.14443105471598));
#19883=CARTESIAN_POINT('Ctrl Pts',(3.60892557137656,2.15730570431671,5.13331726565918));
#19884=CARTESIAN_POINT('Ctrl Pts',(3.40093971248811,2.26086517215761,5.12220347660237));
#19885=CARTESIAN_POINT('Ctrl Pts',(3.37514571617861,2.4917888042929,5.11108968754557));
#19886=CARTESIAN_POINT('Ctrl Pts',(3.55516852834243,2.63869087044012,5.09997589848876));
#19887=CARTESIAN_POINT('Ctrl Pts',(3.77622353148193,2.56711958879047,5.08886210943196));
#19888=CARTESIAN_POINT('Ctrl Pts',(3.8359804180852,2.34258029751366,5.07774832037515));
#19889=CARTESIAN_POINT('Ctrl Pts',(3.6797411123384,2.17059868763558,5.06663453131835));
#19890=CARTESIAN_POINT('Ctrl Pts',(3.45051418153466,2.2085903127083,5.05552074226155));
#19891=CARTESIAN_POINT('Ctrl Pts',(3.3581131561336,2.4217815890047,5.04440695320474));
#19892=CARTESIAN_POINT('Ctrl Pts',(3.48711398178203,2.61503583311392,5.03329316414794));
#19893=CARTESIAN_POINT('Ctrl Pts',(3.71944062032543,2.61146538882495,5.02217937509113));
#19894=CARTESIAN_POINT('Ctrl Pts',(3.84244192441188,2.41433825182845,5.01106558603433));
#19895=CARTESIAN_POINT('Ctrl Pts',(3.74353337567863,2.20408716238119,4.99995179697753));
#19896=CARTESIAN_POINT('Ctrl Pts',(3.51324710536571,2.17315730898832,4.98883800792072));
#19897=CARTESIAN_POINT('Ctrl Pts',(3.36236674087989,2.34985914625667,4.97772421886392));
#19898=CARTESIAN_POINT('Ctrl Pts',(3.42899479464802,2.5724554740903,4.96661042980711));
#19899=CARTESIAN_POINT('Ctrl Pts',(3.652145851588,2.63720135146115,4.95549664075031));
#19900=CARTESIAN_POINT('Ctrl Pts',(3.82756721950384,2.48483414141864,4.9443828516935));
#19901=CARTESIAN_POINT('Ctrl Pts',(3.79469373046592,2.25481727983819,4.9332690626367));
#19902=CARTESIAN_POINT('Ctrl Pts',(3.58361486203243,2.15768780841241,4.9221552735799));
#19903=CARTESIAN_POINT('Ctrl Pts',(3.38753349616232,2.28234943400059,4.91104148452309));
#19904=CARTESIAN_POINT('Ctrl Pts',(3.38592513080807,2.51469795687288,4.89992769546629));
#19905=CARTESIAN_POINT('Ctrl Pts',(3.58026192098975,2.64206213906777,4.88881390640948));
#19906=CARTESIAN_POINT('Ctrl Pts',(3.79266519873933,2.54786410019675,4.87770011735268));
#19907=CARTESIAN_POINT('Ctrl Pts',(3.82871983510845,2.3183243735256,4.86658632829587));
#19908=CARTESIAN_POINT('Ctrl Pts',(3.65542461254465,2.16354327402962,4.85547253923907));
#19909=CARTESIAN_POINT('Ctrl Pts',(3.43139861356028,2.22519369741672,4.84435875018226));
#19910=CARTESIAN_POINT('Ctrl Pts',(3.36169537565425,2.44684631199623,4.83324496112547));
#19911=CARTESIAN_POINT('Ctrl Pts',(3.51011506296999,2.62561996593247,4.82213117206865));
#19912=CARTESIAN_POINT('Ctrl Pts',(3.74080745251389,2.59788110634618,4.81101738301186));
#19913=CARTESIAN_POINT('Ctrl Pts',(3.84261718390667,2.38901942599691,4.79990359395504));
#19914=CARTESIAN_POINT('Ctrl Pts',(3.72235665540369,2.19020838956081,4.78878980489825));
#19915=CARTESIAN_POINT('Ctrl Pts',(3.49010169259086,2.18342199335841,4.77767601584144));
#19916=CARTESIAN_POINT('Ctrl Pts',(3.35843789688119,2.37487190279669,4.76656222678464));
#19917=CARTESIAN_POINT('Ctrl Pts',(3.44787863365674,2.58932184457717,4.75544843772783));
#19918=CARTESIAN_POINT('Ctrl Pts',(3.67655778221991,2.63048335496042,4.74433464867103));
#19919=CARTESIAN_POINT('Ctrl Pts',(3.8351627244929,2.46068083668937,4.73322085961423));
#19920=CARTESIAN_POINT('Ctrl Pts',(3.77852055811084,2.23533646042905,4.72210707055742));
#19921=CARTESIAN_POINT('Ctrl Pts',(3.55847650032912,2.16071048934957,4.71099328150062));
#19922=CARTESIAN_POINT('Ctrl Pts',(3.37643937270466,2.30510892109605,4.69987949244382));
#19923=CARTESIAN_POINT('Ctrl Pts',(3.39902982259358,2.53636223350135,4.68876570338701));
#19924=CARTESIAN_POINT('Ctrl Pts',(3.60557055501943,2.64280164712995,4.67765191433021));
#19925=CARTESIAN_POINT('Ctrl Pts',(3.80701249526159,2.52700195958257,4.6665381252734));
#19926=CARTESIAN_POINT('Ctrl Pts',(3.81897355090948,2.29495593812904,4.65542433621659));
#19927=CARTESIAN_POINT('Ctrl Pts',(3.63050563208088,2.15905793778677,4.6443105471598));
#19928=CARTESIAN_POINT('Ctrl Pts',(3.41411556225142,2.24369693945694,4.63319675810298));
#19929=CARTESIAN_POINT('Ctrl Pts',(3.3678676263658,2.47140190503977,4.62208296904619));
#19930=CARTESIAN_POINT('Ctrl Pts',(3.53409308462842,2.63375189718637,4.61096917998938));
#19931=CARTESIAN_POINT('Ctrl Pts',(3.76064388996454,2.58214612691277,4.59985539093257));
#19932=CARTESIAN_POINT('Ctrl Pts',(3.84015552099323,2.36381994099575,4.58874160187577));
#19933=CARTESIAN_POINT('Ctrl Pts',(3.6998500801025,2.17860977340027,4.57762781281896));
#19934=CARTESIAN_POINT('Ctrl Pts',(3.46815072852799,2.1960405909371,4.56651402376216));
#19935=CARTESIAN_POINT('Ctrl Pts',(3.3571345103823,2.40015776866696,4.55540023470536));
#19936=CARTESIAN_POINT('Ctrl Pts',(3.46841582920963,2.6041305389052,4.54428644564855));
#19937=CARTESIAN_POINT('Ctrl Pts',(3.70013763173937,2.6212603119689,4.53317265659175));
#19938=CARTESIAN_POINT('Ctrl Pts',(3.84020232447629,2.43586801205837,4.52205886753494));
#19939=CARTESIAN_POINT('Ctrl Pts',(3.76040710518764,2.21764531427324,4.51094507847815));
#19940=CARTESIAN_POINT('Ctrl Pts',(3.53378944408678,2.16633392770918,4.49983128942133));
#19941=CARTESIAN_POINT('Ctrl Pts',(3.36777505427786,2.32889974840269,4.48871750036454));
#19942=CARTESIAN_POINT('Ctrl Pts',(3.4143187937299,2.55654443303944,4.47760371130772));
#19943=CARTESIAN_POINT('Ctrl Pts',(3.63081864137997,2.64090222813732,4.46648992225093));
#19944=CARTESIAN_POINT('Ctrl Pts',(3.81910984841827,2.50475947107891,4.45537613319412));
#19945=CARTESIAN_POINT('Ctrl Pts',(3.80684730359907,2.27272920356226,4.44426234413732));
#19946=CARTESIAN_POINT('Ctrl Pts',(3.60525512148808,2.15719129638054,4.43314855508051));
#19947=CARTESIAN_POINT('Ctrl Pts',(3.39885277598246,2.26389903533996,4.42203476602371));
#19948=CARTESIAN_POINT('Ctrl Pts',(3.3765629481812,2.49518135839549,4.4109209769669));
#19949=CARTESIAN_POINT('Ctrl Pts',(3.55878722266986,2.63934344974957,4.3998071879101));
#19950=CARTESIAN_POINT('Ctrl Pts',(3.77873475080197,2.56443107632444,4.38869339885329));
#19951=CARTESIAN_POINT('Ctrl Pts',(3.8350828706128,2.33901445723046,4.37757960979649));
#19952=CARTESIAN_POINT('Ctrl Pts',(3.67625990394949,2.16941582752504,4.36646582073968));
#19953=CARTESIAN_POINT('Ctrl Pts',(3.44762951395987,2.21087905095695,4.35535203168288));
#19954=CARTESIAN_POINT('Ctrl Pts',(3.35847730739013,2.42543572165447,4.34423824262608));
#19955=CARTESIAN_POINT('Ctrl Pts',(3.49037003538787,2.61673301642169,4.33312445356927));
#19956=CARTESIAN_POINT('Ctrl Pts',(3.72265542052987,2.60960761604941,4.32201066451248));
#19957=CARTESIAN_POINT('Ctrl Pts',(3.84257850979074,2.41071512516748,4.31089687545566));
#19958=CARTESIAN_POINT('Ctrl Pts',(3.7406568756376,2.20183613957205,4.29978308639887));
#19959=CARTESIAN_POINT('Ctrl Pts',(3.50959639242813,2.17470169312488,4.28866929734205));
#19960=CARTESIAN_POINT('Ctrl Pts',(3.41142456563631,2.29356865430551,4.28126010463752));
#19961=CARTESIAN_POINT('Ctrl Pts',(3.39833241385534,2.360627924571,4.27755550828525));
#19962=CARTESIAN_POINT('Ctrl Pts',(3.55032651029123,2.21400211999972,5.20748149723825));
#19963=CARTESIAN_POINT('Ctrl Pts',(3.48847779011663,2.2305197371096,5.20377690088598));
#19964=CARTESIAN_POINT('Ctrl Pts',(3.38363102379655,2.32987260795489,5.19636770818144));
#19965=CARTESIAN_POINT('Ctrl Pts',(3.42374108957258,2.54412674142112,5.18525391912464));
#19966=CARTESIAN_POINT('Ctrl Pts',(3.62549702318155,2.62606856404868,5.17414013006783));
#19967=CARTESIAN_POINT('Ctrl Pts',(3.8037602238433,2.50127641096634,5.16302634101103));
#19968=CARTESIAN_POINT('Ctrl Pts',(3.79559667859298,2.28369088196908,5.15191255195422));
#19969=CARTESIAN_POINT('Ctrl Pts',(3.60836267793897,2.1726112820345,5.14079876289743));
#19970=CARTESIAN_POINT('Ctrl Pts',(3.41349350034069,2.269639745597,5.12968497384062));
#19971=CARTESIAN_POINT('Ctrl Pts',(3.38932620899373,2.48600011991624,5.11857118478381));
#19972=CARTESIAN_POINT('Ctrl Pts',(3.55799583654811,2.62363776975738,5.10745739572701));
#19973=CARTESIAN_POINT('Ctrl Pts',(3.76510994947867,2.55658014925731,5.0963436066702));
#19974=CARTESIAN_POINT('Ctrl Pts',(3.82109825277221,2.34620148571036,5.08522981761341));
#19975=CARTESIAN_POINT('Ctrl Pts',(3.67471221873066,2.18506593996663,5.0741160285566));
#19976=CARTESIAN_POINT('Ctrl Pts',(3.45994154284032,2.22066161350478,5.0630022394998));
#19977=CARTESIAN_POINT('Ctrl Pts',(3.37336781169642,2.42040792753322,5.05188845044299));
#19978=CARTESIAN_POINT('Ctrl Pts',(3.49423316734106,2.60147454339935,5.04077466138619));
#19979=CARTESIAN_POINT('Ctrl Pts',(3.71190806711109,2.59812927009101,5.02966087232938));
#19980=CARTESIAN_POINT('Ctrl Pts',(3.82715226255275,2.41343400631629,5.01854708327258));
#19981=CARTESIAN_POINT('Ctrl Pts',(3.73448140669699,2.21644245550271,5.00743329421577));
#19982=CARTESIAN_POINT('Ctrl Pts',(3.51871819881407,2.18746320121053,4.99631950515897));
#19983=CARTESIAN_POINT('Ctrl Pts',(3.37735314303472,2.35302129199909,4.98520571610216));
#19984=CARTESIAN_POINT('Ctrl Pts',(3.43977928158165,2.56157952558844,4.97409192704536));
#19985=CARTESIAN_POINT('Ctrl Pts',(3.64885726014462,2.62224218767309,4.96297813798855));
#19986=CARTESIAN_POINT('Ctrl Pts',(3.81321563470729,2.47948405463168,4.95186434893176));
#19987=CARTESIAN_POINT('Ctrl Pts',(3.78241532064824,2.26397326515074,4.94075055987495));
#19988=CARTESIAN_POINT('Ctrl Pts',(3.58464819494153,2.17296928863785,4.92963677081815));
#19989=CARTESIAN_POINT('Ctrl Pts',(3.40093275047013,2.28976909698186,4.91852298176134));
#19990=CARTESIAN_POINT('Ctrl Pts',(3.39942581708757,2.50746450093999,4.90740919270454));
#19991=CARTESIAN_POINT('Ctrl Pts',(3.58150670798172,2.62679642846834,4.89629540364773));
#19992=CARTESIAN_POINT('Ctrl Pts',(3.78051471879288,2.53853901296773,4.88518161459093));
#19993=CARTESIAN_POINT('Ctrl Pts',(3.81429556031454,2.32347526776122,4.87406782553412));
#19994=CARTESIAN_POINT('Ctrl Pts',(3.65192924520447,2.17845547782099,4.86295403647733));
#19995=CARTESIAN_POINT('Ctrl Pts',(3.4420315030405,2.23621790151766,4.85184024742051));
#19996=CARTESIAN_POINT('Ctrl Pts',(3.37672411762845,2.4438919373702,4.84072645836372));
#19997=CARTESIAN_POINT('Ctrl Pts',(3.51578367947165,2.61139118517954,4.8296126693069));
#19998=CARTESIAN_POINT('Ctrl Pts',(3.73192739457257,2.58540168385487,4.81849888025011));
#19999=CARTESIAN_POINT('Ctrl Pts',(3.82731646926276,2.38971191869978,4.8073850911933));
#20000=CARTESIAN_POINT('Ctrl Pts',(3.71464020169267,2.20343895103354,4.7962713021365));
#20001=CARTESIAN_POINT('Ctrl Pts',(3.49703245740495,2.19708054064022,4.78515751307969));
#20002=CARTESIAN_POINT('Ctrl Pts',(3.37367207258585,2.37645661266209,4.77404372402289));
#20003=CARTESIAN_POINT('Ctrl Pts',(3.45747220646219,2.57738221411453,4.76292993496608));
#20004=CARTESIAN_POINT('Ctrl Pts',(3.6717296461388,2.6159478633368,4.75181614590928));
#20005=CARTESIAN_POINT('Ctrl Pts',(3.82033212723505,2.45685398423157,4.74070235685248));
#20006=CARTESIAN_POINT('Ctrl Pts',(3.7672621135368,2.24572100859114,4.72958856779567));
#20007=CARTESIAN_POINT('Ctrl Pts',(3.56109519043692,2.17580134343001,4.71847477873887));
#20008=CARTESIAN_POINT('Ctrl Pts',(3.39053828074069,2.31109325121307,4.70736098968206));
#20009=CARTESIAN_POINT('Ctrl Pts',(3.41170405813995,2.52776251443194,4.69624720062526));
#20010=CARTESIAN_POINT('Ctrl Pts',(3.60521924654496,2.62748929926577,4.68513341156846));
#20011=CARTESIAN_POINT('Ctrl Pts',(3.79395719939706,2.51899254857754,4.67401962251165));
#20012=CARTESIAN_POINT('Ctrl Pts',(3.80516392801682,2.30158056870897,4.66290583345484));
#20013=CARTESIAN_POINT('Ctrl Pts',(3.62858178660552,2.17425301045342,4.65179204439804));
#20014=CARTESIAN_POINT('Ctrl Pts',(3.42583841177484,2.25355423187469,4.64067825534123));
#20015=CARTESIAN_POINT('Ctrl Pts',(3.38250711377307,2.46689892566933,4.62956446628444));
#20016=CARTESIAN_POINT('Ctrl Pts',(3.53824952107254,2.61901027411281,4.61845067722762));
#20017=CARTESIAN_POINT('Ctrl Pts',(3.7505128420311,2.57065903491661,4.60733688817083));
#20018=CARTESIAN_POINT('Ctrl Pts',(3.82501005174943,2.36610164565372,4.59622309911402));
#20019=CARTESIAN_POINT('Ctrl Pts',(3.69355300930883,2.19257180456232,4.58510931005721));
#20020=CARTESIAN_POINT('Ctrl Pts',(3.47646583649485,2.20890334314105,4.57399552100041));
#20021=CARTESIAN_POINT('Ctrl Pts',(3.37245088448926,2.4001478189457,4.5628817319436));
#20022=CARTESIAN_POINT('Ctrl Pts',(3.47671421853432,2.59125699435405,4.55176794288681));
#20023=CARTESIAN_POINT('Ctrl Pts',(3.69382242642831,2.60730647390622,4.54065415382999));
#20024=CARTESIAN_POINT('Ctrl Pts',(3.82505390355888,2.43360598672071,4.5295403647732));
#20025=CARTESIAN_POINT('Ctrl Pts',(3.75029099014661,2.22914555908425,4.51842657571639));
#20026=CARTESIAN_POINT('Ctrl Pts',(3.53796502969918,2.18107013821379,4.50731278665959));
#20027=CARTESIAN_POINT('Ctrl Pts',(3.3824203797675,2.33338370392177,4.49619899760278));
#20028=CARTESIAN_POINT('Ctrl Pts',(3.42602882640825,2.54667191840358,4.48508520854598));
#20029=CARTESIAN_POINT('Ctrl Pts',(3.62887505589326,2.62570966761684,4.47397141948917));
#20030=CARTESIAN_POINT('Ctrl Pts',(3.80529162988842,2.49815278828994,4.46285763043237));
#20031=CARTESIAN_POINT('Ctrl Pts',(3.79380242558891,2.28075556883219,4.45174384137556));
#20032=CARTESIAN_POINT('Ctrl Pts',(3.60492370590979,2.17250408926403,4.44063005231877));
#20033=CARTESIAN_POINT('Ctrl Pts',(3.41153817701856,2.2724822774232,4.42951626326195));
#20034=CARTESIAN_POINT('Ctrl Pts',(3.39065406289825,2.48917872172821,4.41840247420516));
#20035=CARTESIAN_POINT('Ctrl Pts',(3.56138631699392,2.62424919398607,4.40728868514835));
#20036=CARTESIAN_POINT('Ctrl Pts',(3.76746279811117,2.55406118851634,4.39617489609155));
#20037=CARTESIAN_POINT('Ctrl Pts',(3.82025730936029,2.342860526055,4.38506110703474));
#20038=CARTESIAN_POINT('Ctrl Pts',(3.67145055363756,2.18395767723095,4.37394731797794));
#20039=CARTESIAN_POINT('Ctrl Pts',(3.4572387975626,2.22280601189145,4.36283352892113));
#20040=CARTESIAN_POINT('Ctrl Pts',(3.37370899766098,2.42383161137452,4.35171973986432));
#20041=CARTESIAN_POINT('Ctrl Pts',(3.49728387709496,2.60306469340852,4.34060595080753));
#20042=CARTESIAN_POINT('Ctrl Pts',(3.71492012511989,2.59638865822985,4.32949216175072));
#20043=CARTESIAN_POINT('Ctrl Pts',(3.82728023413982,2.4100393730632,4.31837837269392));
#20044=CARTESIAN_POINT('Ctrl Pts',(3.73178631386543,2.21433339402172,4.30726458363711));
#20045=CARTESIAN_POINT('Ctrl Pts',(3.51529771901994,2.18891018836724,4.29615079458031));
#20046=CARTESIAN_POINT('Ctrl Pts',(3.42331712354828,2.30028077429395,4.28874160187577));
#20047=CARTESIAN_POINT('Ctrl Pts',(3.41105063166184,2.36311093455973,4.2850370055235));
#20048=CARTESIAN_POINT('Ctrl Pts',(3.55367004230132,2.22652167256662,5.2149629944765));
#20049=CARTESIAN_POINT('Ctrl Pts',(3.49598437120782,2.24192748573719,5.21125839812423));
#20050=CARTESIAN_POINT('Ctrl Pts',(3.39819486060706,2.33459289600918,5.20384920541969));
#20051=CARTESIAN_POINT('Ctrl Pts',(3.43560511025108,2.5344255431305,5.19273541636289));
#20052=CARTESIAN_POINT('Ctrl Pts',(3.62378081371712,2.61085184614133,5.18162162730608));
#20053=CARTESIAN_POINT('Ctrl Pts',(3.79004508454469,2.4944594765428,5.17050783824928));
#20054=CARTESIAN_POINT('Ctrl Pts',(3.78243102907294,2.29151967075525,5.15939404919247));
#20055=CARTESIAN_POINT('Ctrl Pts',(3.60779978450139,2.18791685975229,5.14828026013568));
#20056=CARTESIAN_POINT('Ctrl Pts',(3.42604728819327,2.27841431903638,5.13716647107886));
#20057=CARTESIAN_POINT('Ctrl Pts',(3.40350670180884,2.48021143553957,5.12605268202207));
#20058=CARTESIAN_POINT('Ctrl Pts',(3.56082314475379,2.60858466907463,5.11493889296526));
#20059=CARTESIAN_POINT('Ctrl Pts',(3.75399636747541,2.54604070972415,5.10382510390846));
#20060=CARTESIAN_POINT('Ctrl Pts',(3.80621608745921,2.34982267390707,5.09271131485165));
#20061=CARTESIAN_POINT('Ctrl Pts',(3.66968332512291,2.19953319229768,5.08159752579485));
#20062=CARTESIAN_POINT('Ctrl Pts',(3.46936890414598,2.23273291430124,5.07048373673804));
#20063=CARTESIAN_POINT('Ctrl Pts',(3.38862246725923,2.41903426606174,5.05936994768124));
#20064=CARTESIAN_POINT('Ctrl Pts',(3.50135235290009,2.58791325368478,5.04825615862443));
#20065=CARTESIAN_POINT('Ctrl Pts',(3.70437551389675,2.58479315135706,5.03714236956764));
#20066=CARTESIAN_POINT('Ctrl Pts',(3.81186260069363,2.41252976080414,5.02602858051082));
#20067=CARTESIAN_POINT('Ctrl Pts',(3.72542943771535,2.22879774862422,5.01491479145403));
#20068=CARTESIAN_POINT('Ctrl Pts',(3.52418929226243,2.20176909343275,5.00380100239722));
#20069=CARTESIAN_POINT('Ctrl Pts',(3.39233954518956,2.35618343774151,4.99268721334042));
#20070=CARTESIAN_POINT('Ctrl Pts',(3.45056376851527,2.55070357708658,4.98157342428361));
#20071=CARTESIAN_POINT('Ctrl Pts',(3.64556866870124,2.60728302388504,4.9704596352268));
#20072=CARTESIAN_POINT('Ctrl Pts',(3.79886404991074,2.47413396784473,4.95934584617));
#20073=CARTESIAN_POINT('Ctrl Pts',(3.77013691083056,2.27312925046329,4.9482320571132));
#20074=CARTESIAN_POINT('Ctrl Pts',(3.58568152785062,2.18825076886329,4.93711826805639));
#20075=CARTESIAN_POINT('Ctrl Pts',(3.41433200477794,2.29718875996312,4.92600447899959));
#20076=CARTESIAN_POINT('Ctrl Pts',(3.41292650336706,2.5002310450071,4.91489068994278));
#20077=CARTESIAN_POINT('Ctrl Pts',(3.58275149497368,2.61153071786889,4.90377690088598));
#20078=CARTESIAN_POINT('Ctrl Pts',(3.76836423884643,2.52921392573871,4.89266311182918));
#20079=CARTESIAN_POINT('Ctrl Pts',(3.79987128552062,2.32862616199684,4.88154932277237));
#20080=CARTESIAN_POINT('Ctrl Pts',(3.64843387786428,2.19336768161237,4.87043553371557));
#20081=CARTESIAN_POINT('Ctrl Pts',(3.45266439252072,2.24724210561861,4.85932174465876));
#20082=CARTESIAN_POINT('Ctrl Pts',(3.39175285960263,2.44093756274417,4.84820795560197));
#20083=CARTESIAN_POINT('Ctrl Pts',(3.52145229597333,2.59716240442661,4.83709416654515));
#20084=CARTESIAN_POINT('Ctrl Pts',(3.72304733663125,2.57292226136356,4.82598037748836));
#20085=CARTESIAN_POINT('Ctrl Pts',(3.81201575461885,2.39040441140265,4.81486658843155));
#20086=CARTESIAN_POINT('Ctrl Pts',(3.70692374798164,2.21666951250626,4.80375279937475));
#20087=CARTESIAN_POINT('Ctrl Pts',(3.50396322221905,2.21073908792203,4.79263901031794));
#20088=CARTESIAN_POINT('Ctrl Pts',(3.3889062482905,2.37804132252749,4.78152522126113));
#20089=CARTESIAN_POINT('Ctrl Pts',(3.46706577926762,2.56544258365188,4.77041143220433));
#20090=CARTESIAN_POINT('Ctrl Pts',(3.66690151005769,2.60141237171319,4.75929764314753));
#20091=CARTESIAN_POINT('Ctrl Pts',(3.80550152997722,2.45302713177377,4.74818385409072));
#20092=CARTESIAN_POINT('Ctrl Pts',(3.75600366896275,2.25610555675324,4.73707006503392));
#20093=CARTESIAN_POINT('Ctrl Pts',(3.56371388054473,2.19089219751045,4.72595627597711));
#20094=CARTESIAN_POINT('Ctrl Pts',(3.40463718877671,2.31707758133011,4.71484248692031));
#20095=CARTESIAN_POINT('Ctrl Pts',(3.42437829368633,2.51916279536252,4.7037286978635));
#20096=CARTESIAN_POINT('Ctrl Pts',(3.60486793807048,2.61217695140159,4.69261490880671));
#20097=CARTESIAN_POINT('Ctrl Pts',(3.78090190353252,2.51098313757252,4.6815011197499));
#20098=CARTESIAN_POINT('Ctrl Pts',(3.79135430512417,2.3082051992889,4.67038733069309));
#20099=CARTESIAN_POINT('Ctrl Pts',(3.62665794113017,2.18944808312007,4.65927354163629));
#20100=CARTESIAN_POINT('Ctrl Pts',(3.43756126129826,2.26341152429244,4.64815975257949));
#20101=CARTESIAN_POINT('Ctrl Pts',(3.39714660118035,2.46239594629889,4.63704596352268));
#20102=CARTESIAN_POINT('Ctrl Pts',(3.54240595751667,2.60426865103925,4.62593217446588));
#20103=CARTESIAN_POINT('Ctrl Pts',(3.74038179409766,2.55917194292045,4.61481838540907));
#20104=CARTESIAN_POINT('Ctrl Pts',(3.80986458250562,2.36838335031169,4.60370459635227));
#20105=CARTESIAN_POINT('Ctrl Pts',(3.68725593851517,2.20653383572437,4.59259080729547));
#20106=CARTESIAN_POINT('Ctrl Pts',(3.48478094446172,2.221766095345,4.58147701823866));
#20107=CARTESIAN_POINT('Ctrl Pts',(3.38776725859624,2.40013786922444,4.57036322918186));
#20108=CARTESIAN_POINT('Ctrl Pts',(3.48501260785902,2.57838344980291,4.55924944012505));
#20109=CARTESIAN_POINT('Ctrl Pts',(3.68750722111726,2.59335263584353,4.54813565106824));
#20110=CARTESIAN_POINT('Ctrl Pts',(3.80990548264146,2.43134396138305,4.53702186201145));
#20111=CARTESIAN_POINT('Ctrl Pts',(3.74017487510557,2.24064580389526,4.52590807295464));
#20112=CARTESIAN_POINT('Ctrl Pts',(3.54214061531159,2.19580634871841,4.51479428389784));
#20113=CARTESIAN_POINT('Ctrl Pts',(3.39706570525713,2.33786765944084,4.50368049484103));
#20114=CARTESIAN_POINT('Ctrl Pts',(3.4377388590866,2.53679940376773,4.49256670578423));
#20115=CARTESIAN_POINT('Ctrl Pts',(3.62693147040654,2.61051710709635,4.48145291672742));
#20116=CARTESIAN_POINT('Ctrl Pts',(3.79147341135858,2.49154610550097,4.47033912767062));
#20117=CARTESIAN_POINT('Ctrl Pts',(3.78075754757875,2.28878193410212,4.45922533861381));
#20118=CARTESIAN_POINT('Ctrl Pts',(3.60459229033149,2.18781688214753,4.44811154955701));
#20119=CARTESIAN_POINT('Ctrl Pts',(3.42422357805467,2.28106551950643,4.43699776050021));
#20120=CARTESIAN_POINT('Ctrl Pts',(3.4047451776153,2.48317608506094,4.4258839714434));
#20121=CARTESIAN_POINT('Ctrl Pts',(3.56398541131798,2.60915493822257,4.4147701823866));
#20122=CARTESIAN_POINT('Ctrl Pts',(3.75619084542037,2.54369130070823,4.40365639332979));
#20123=CARTESIAN_POINT('Ctrl Pts',(3.80543174810779,2.34670659487954,4.39254260427299));
#20124=CARTESIAN_POINT('Ctrl Pts',(3.66664120332562,2.19849952693685,4.38142881521618));
#20125=CARTESIAN_POINT('Ctrl Pts',(3.46684808116532,2.23473297282595,4.37031502615938));
#20126=CARTESIAN_POINT('Ctrl Pts',(3.38894068793183,2.42222750109457,4.35920123710257));
#20127=CARTESIAN_POINT('Ctrl Pts',(3.50419771880206,2.58939637039535,4.34808744804578));
#20128=CARTESIAN_POINT('Ctrl Pts',(3.70718482970991,2.5831697004103,4.33697365898896));
#20129=CARTESIAN_POINT('Ctrl Pts',(3.81198195848891,2.40936362095891,4.32585986993217));
#20130=CARTESIAN_POINT('Ctrl Pts',(3.72291575209325,2.22683064847139,4.31474608087536));
#20131=CARTESIAN_POINT('Ctrl Pts',(3.52099904561175,2.2031186836096,4.30363229181856));
#20132=CARTESIAN_POINT('Ctrl Pts',(3.43520968146025,2.30699289428239,4.29622309911402));
#20133=CARTESIAN_POINT('Ctrl Pts',(3.42376884946835,2.36559394454846,4.29251850276175));
#20134=CARTESIAN_POINT('Ctrl Pts',(3.55701357431141,2.23904122513352,5.22244449171475));
#20135=CARTESIAN_POINT('Ctrl Pts',(3.50349095229901,2.25333523436478,5.21873989536248));
#20136=CARTESIAN_POINT('Ctrl Pts',(3.41275869741756,2.33931318406347,5.21133070265794));
#20137=CARTESIAN_POINT('Ctrl Pts',(3.44746913092958,2.52472434483988,5.20021691360114));
#20138=CARTESIAN_POINT('Ctrl Pts',(3.62206460425269,2.59563512823397,5.18910312454433));
#20139=CARTESIAN_POINT('Ctrl Pts',(3.77632994524609,2.48764254211926,5.17798933548754));
#20140=CARTESIAN_POINT('Ctrl Pts',(3.76926537955289,2.29934845954141,5.16687554643072));
#20141=CARTESIAN_POINT('Ctrl Pts',(3.60723689106381,2.20322243747008,5.15576175737393));
#20142=CARTESIAN_POINT('Ctrl Pts',(3.43860107604584,2.28718889247577,5.14464796831712));
#20143=CARTESIAN_POINT('Ctrl Pts',(3.41768719462395,2.47442275116291,5.13353417926031));
#20144=CARTESIAN_POINT('Ctrl Pts',(3.56365045295948,2.59353156839189,5.12242039020351));
#20145=CARTESIAN_POINT('Ctrl Pts',(3.74288278547214,2.53550127019098,5.1113066011467));
#20146=CARTESIAN_POINT('Ctrl Pts',(3.79133392214622,2.35344386210378,5.1001928120899));
#20147=CARTESIAN_POINT('Ctrl Pts',(3.66465443151516,2.21400044462873,5.0890790230331));
#20148=CARTESIAN_POINT('Ctrl Pts',(3.47879626545164,2.24480421509772,5.0779652339763));
#20149=CARTESIAN_POINT('Ctrl Pts',(3.40387712282204,2.41766060459026,5.06685144491948));
#20150=CARTESIAN_POINT('Ctrl Pts',(3.50847153845911,2.57435196397021,5.05573765586269));
#20151=CARTESIAN_POINT('Ctrl Pts',(3.69684296068241,2.57145703262312,5.04462386680587));
#20152=CARTESIAN_POINT('Ctrl Pts',(3.7965729388345,2.41162551529198,5.03351007774909));
#20153=CARTESIAN_POINT('Ctrl Pts',(3.71637746873371,2.24115304174574,5.02239628869227));
#20154=CARTESIAN_POINT('Ctrl Pts',(3.5296603857108,2.21607498565497,5.01128249963547));
#20155=CARTESIAN_POINT('Ctrl Pts',(3.40732594734439,2.35934558348393,5.00016871057866));
#20156=CARTESIAN_POINT('Ctrl Pts',(3.46134825544889,2.53982762858472,4.98905492152187));
#20157=CARTESIAN_POINT('Ctrl Pts',(3.64228007725786,2.59232386009698,4.97794113246505));
#20158=CARTESIAN_POINT('Ctrl Pts',(3.7845124651142,2.46878388105777,4.96682734340826));
#20159=CARTESIAN_POINT('Ctrl Pts',(3.75785850101288,2.28228523577585,4.95571355435144));
#20160=CARTESIAN_POINT('Ctrl Pts',(3.58671486075972,2.20353224908873,4.94459976529465));
#20161=CARTESIAN_POINT('Ctrl Pts',(3.42773125908574,2.30460842294439,4.93348597623783));
#20162=CARTESIAN_POINT('Ctrl Pts',(3.42642718964655,2.4929975890742,4.92237218718104));
#20163=CARTESIAN_POINT('Ctrl Pts',(3.58399628196565,2.59626500726946,4.91125839812423));
#20164=CARTESIAN_POINT('Ctrl Pts',(3.75621375889998,2.51988883850969,4.90014460906743));
#20165=CARTESIAN_POINT('Ctrl Pts',(3.7854470107267,2.33377705623246,4.88903082001062));
#20166=CARTESIAN_POINT('Ctrl Pts',(3.6449385105241,2.20827988540375,4.87791703095382));
#20167=CARTESIAN_POINT('Ctrl Pts',(3.46329728200094,2.25826630971955,4.86680324189701));
#20168=CARTESIAN_POINT('Ctrl Pts',(3.40678160157682,2.43798318811813,4.85568945284022));
#20169=CARTESIAN_POINT('Ctrl Pts',(3.527120912475,2.58293362367368,4.8445756637834));
#20170=CARTESIAN_POINT('Ctrl Pts',(3.71416727868993,2.56044283887224,4.8334618747266));
#20171=CARTESIAN_POINT('Ctrl Pts',(3.79671503997494,2.39109690410553,4.82234808566979));
#20172=CARTESIAN_POINT('Ctrl Pts',(3.69920729427062,2.22990007397898,4.811234296613));
#20173=CARTESIAN_POINT('Ctrl Pts',(3.51089398703315,2.22439763520385,4.80012050755619));
#20174=CARTESIAN_POINT('Ctrl Pts',(3.40414042399517,2.37962603239289,4.78900671849938));
#20175=CARTESIAN_POINT('Ctrl Pts',(3.47665935207306,2.55350295318923,4.77789292944258));
#20176=CARTESIAN_POINT('Ctrl Pts',(3.66207337397658,2.58687688008957,4.76677914038578));
#20177=CARTESIAN_POINT('Ctrl Pts',(3.79067093271938,2.44920027931597,4.75566535132897));
#20178=CARTESIAN_POINT('Ctrl Pts',(3.7447452243887,2.26649010491534,4.74455156227217));
#20179=CARTESIAN_POINT('Ctrl Pts',(3.56633257065254,2.20598305159089,4.73343777321536));
#20180=CARTESIAN_POINT('Ctrl Pts',(3.41873609681274,2.32306191144714,4.72232398415856));
#20181=CARTESIAN_POINT('Ctrl Pts',(3.4370525292327,2.5105630762931,4.71121019510175));
#20182=CARTESIAN_POINT('Ctrl Pts',(3.604516629596,2.59686460353741,4.70009640604495));
#20183=CARTESIAN_POINT('Ctrl Pts',(3.76784660766799,2.50297372656749,4.68898261698814));
#20184=CARTESIAN_POINT('Ctrl Pts',(3.77754468223151,2.31482982986883,4.67786882793134));
#20185=CARTESIAN_POINT('Ctrl Pts',(3.62473409565482,2.20464315578672,4.66675503887454));
#20186=CARTESIAN_POINT('Ctrl Pts',(3.44928411082169,2.27326881671019,4.65564124981774));
#20187=CARTESIAN_POINT('Ctrl Pts',(3.41178608858762,2.45789296692846,4.64452746076093));
#20188=CARTESIAN_POINT('Ctrl Pts',(3.5465623939608,2.58952702796569,4.63341367170412));
#20189=CARTESIAN_POINT('Ctrl Pts',(3.73025074616421,2.54768485092428,4.62229988264732));
#20190=CARTESIAN_POINT('Ctrl Pts',(3.79471911326182,2.37066505496967,4.61118609359052));
#20191=CARTESIAN_POINT('Ctrl Pts',(3.6809588677215,2.22049586688641,4.60007230453371));
#20192=CARTESIAN_POINT('Ctrl Pts',(3.49309605242859,2.23462884754895,4.58895851547691));
#20193=CARTESIAN_POINT('Ctrl Pts',(3.4030836327032,2.40012791950318,4.5778447264201));
#20194=CARTESIAN_POINT('Ctrl Pts',(3.49331099718372,2.56550990525176,4.56673093736331));
#20195=CARTESIAN_POINT('Ctrl Pts',(3.6811920158062,2.57939879778085,4.55561714830649));
#20196=CARTESIAN_POINT('Ctrl Pts',(3.79475706172405,2.42908193604538,4.5445033592497));
#20197=CARTESIAN_POINT('Ctrl Pts',(3.73005876006454,2.25214604870627,4.53338957019289));
#20198=CARTESIAN_POINT('Ctrl Pts',(3.54631620092399,2.21054255922302,4.52227578113609));
#20199=CARTESIAN_POINT('Ctrl Pts',(3.41171103074677,2.34235161495991,4.51116199207928));
#20200=CARTESIAN_POINT('Ctrl Pts',(3.44944889176494,2.52692688913187,4.50004820302248));
#20201=CARTESIAN_POINT('Ctrl Pts',(3.62498788491984,2.59532454657587,4.48893441396567));
#20202=CARTESIAN_POINT('Ctrl Pts',(3.77765519282873,2.484939422712,4.47782062490886));
#20203=CARTESIAN_POINT('Ctrl Pts',(3.76771266956859,2.29680829937205,4.46670683585207));
#20204=CARTESIAN_POINT('Ctrl Pts',(3.6042608747532,2.20312967503102,4.45559304679526));
#20205=CARTESIAN_POINT('Ctrl Pts',(3.43690897909078,2.28964876158967,4.44447925773845));
#20206=CARTESIAN_POINT('Ctrl Pts',(3.41883629233234,2.47717344839367,4.43336546868165));
#20207=CARTESIAN_POINT('Ctrl Pts',(3.56658450564204,2.59406068245907,4.42225167962485));
#20208=CARTESIAN_POINT('Ctrl Pts',(3.74491889272957,2.53332141290012,4.41113789056804));
#20209=CARTESIAN_POINT('Ctrl Pts',(3.7906061868553,2.35055266370407,4.40002410151124));
#20210=CARTESIAN_POINT('Ctrl Pts',(3.66183185301368,2.21304137664276,4.38891031245443));
#20211=CARTESIAN_POINT('Ctrl Pts',(3.47645736476805,2.24665993376045,4.37779652339763));
#20212=CARTESIAN_POINT('Ctrl Pts',(3.40417237820268,2.42062339081462,4.36668273434083));
#20213=CARTESIAN_POINT('Ctrl Pts',(3.51111156050916,2.57572804738218,4.35556894528402));
#20214=CARTESIAN_POINT('Ctrl Pts',(3.69944953429992,2.56995074259074,4.34445515622722));
#20215=CARTESIAN_POINT('Ctrl Pts',(3.796683682838,2.40868786885462,4.33334136717041));
#20216=CARTESIAN_POINT('Ctrl Pts',(3.71404519032108,2.23932790292106,4.32222757811361));
#20217=CARTESIAN_POINT('Ctrl Pts',(3.52670037220356,2.21732717885196,4.3111137890568));
#20218=CARTESIAN_POINT('Ctrl Pts',(3.44710223937223,2.31370501427082,4.30370459635227));
#20219=CARTESIAN_POINT('Ctrl Pts',(3.43648706727485,2.36807695453719,4.3));
#20220=CARTESIAN_POINT('Ctrl Pts',(3.43361558566414,2.40009421455432,5.13785196366098));
#20221=CARTESIAN_POINT('Ctrl Pts',(3.43350387426567,2.42168271797136,5.13641270219409));
#20222=CARTESIAN_POINT('Ctrl Pts',(3.43740295903752,2.4432325339629,5.1349734407272));
#20223=CARTESIAN_POINT('Ctrl Pts',(3.44550005125019,2.46306857758655,5.13353417926031));
#20224=CARTESIAN_POINT('Ctrl Pts',(3.46634161406913,2.51412569023923,5.12982958290805));
#20225=CARTESIAN_POINT('Ctrl Pts',(3.5149960335143,2.55382862931556,5.12612498655578));
#20226=CARTESIAN_POINT('Ctrl Pts',(3.56919529865567,2.56400838248691,5.12242039020351));
#20227=CARTESIAN_POINT('Ctrl Pts',(3.62339456379703,2.57418813565826,5.11871579385124));
#20228=CARTESIAN_POINT('Ctrl Pts',(3.68313867463459,2.55484470292462,5.11501119749897));
#20229=CARTESIAN_POINT('Ctrl Pts',(3.72108591949905,2.51483008520994,5.1113066011467));
#20230=CARTESIAN_POINT('Ctrl Pts',(3.7590331643635,2.47481546749525,5.10760200479444));
#20231=CARTESIAN_POINT('Ctrl Pts',(3.77518354325486,2.41412966479952,5.10389740844217));
#20232=CARTESIAN_POINT('Ctrl Pts',(3.76214548426203,2.36054619387247,5.1001928120899));
#20233=CARTESIAN_POINT('Ctrl Pts',(3.7491074252692,2.30696272294543,5.09648821573763));
#20234=CARTESIAN_POINT('Ctrl Pts',(3.70688092839218,2.26048158378708,5.09278361938537));
#20235=CARTESIAN_POINT('Ctrl Pts',(3.65479131894308,2.24237497595273,5.0890790230331));
#20236=CARTESIAN_POINT('Ctrl Pts',(3.60270170949399,2.22426836811839,5.08537442668083));
#20237=CARTESIAN_POINT('Ctrl Pts',(3.54074898747281,2.23453629160805,5.08166983032856));
#20238=CARTESIAN_POINT('Ctrl Pts',(3.49728610269062,2.26847965160164,5.0779652339763));
#20239=CARTESIAN_POINT('Ctrl Pts',(3.45773596364813,2.29936726097326,5.07459414387119));
#20240=CARTESIAN_POINT('Ctrl Pts',(3.43349641790554,2.34985942255505,5.07122305376608));
#20241=CARTESIAN_POINT('Ctrl Pts',(3.43317938608394,2.40008640134203,5.06785196366098));
#20242=CARTESIAN_POINT('Ctrl Pts',(3.54698297828114,2.20148256743283,5.2));
#20243=CARTESIAN_POINT('Ctrl Pts',(3.5345795220974,2.20607510740599,5.2));
#20244=CARTESIAN_POINT('Ctrl Pts',(3.52273022202852,2.21193437307052,5.2));
#20245=CARTESIAN_POINT('Ctrl Pts',(3.51155282869243,2.21889712518446,5.2));
#20246=CARTESIAN_POINT('Ctrl Pts',(3.50588663673039,2.22242677551307,5.2));
#20247=CARTESIAN_POINT('Ctrl Pts',(3.50039354941666,2.2262407482932,5.2));
#20248=CARTESIAN_POINT('Ctrl Pts',(3.49509234222245,2.23032135431632,5.2));
#20249=CARTESIAN_POINT('Ctrl Pts',(3.49050523644823,2.2338522805309,5.2));
#20250=CARTESIAN_POINT('Ctrl Pts',(3.48606182302158,2.23758289719759,5.2));
#20251=CARTESIAN_POINT('Ctrl Pts',(3.48177607353762,2.24150262969935,5.2));
#20252=CARTESIAN_POINT('Ctrl Pts',(3.4786657164721,2.24434735212827,5.2));
#20253=CARTESIAN_POINT('Ctrl Pts',(3.47564458925343,2.24728626535177,5.2));
#20254=CARTESIAN_POINT('Ctrl Pts',(3.47272209234032,2.25030915184069,5.2));
#20255=CARTESIAN_POINT('Ctrl Pts',(3.4637771038367,2.25956140622969,5.2));
#20256=CARTESIAN_POINT('Ctrl Pts',(3.45573639448352,2.26961351156597,5.2));
#20257=CARTESIAN_POINT('Ctrl Pts',(3.44873900472013,2.28033442966861,5.2));
#20258=CARTESIAN_POINT('Ctrl Pts',(3.44420815653473,2.28727628284152,5.2));
#20259=CARTESIAN_POINT('Ctrl Pts',(3.44011557094646,2.29449912284867,5.2));
#20260=CARTESIAN_POINT('Ctrl Pts',(3.43651072814608,2.30197002765831,5.2));
#20261=CARTESIAN_POINT('Ctrl Pts',(3.43484397915084,2.30542430396786,5.2));
#20262=CARTESIAN_POINT('Ctrl Pts',(3.43328563163244,2.30892352292903,5.2));
#20263=CARTESIAN_POINT('Ctrl Pts',(3.43184081732517,2.31246073059787,5.2));
#20264=CARTESIAN_POINT('Ctrl Pts',(3.42783869836044,2.3222587550377,5.2));
#20265=CARTESIAN_POINT('Ctrl Pts',(3.42470154623616,2.33235626573064,5.2));
#20266=CARTESIAN_POINT('Ctrl Pts',(3.42252347569321,2.34267987754179,5.2));
#20267=CARTESIAN_POINT('Ctrl Pts',(3.42066968522458,2.35146646769115,5.2));
#20268=CARTESIAN_POINT('Ctrl Pts',(3.41951139095334,2.36041732716722,5.2));
#20269=CARTESIAN_POINT('Ctrl Pts',(3.41903596356978,2.36945415649734,5.2));
#20270=CARTESIAN_POINT('Ctrl Pts',(3.41886682155969,2.37266917424891,5.2));
#20271=CARTESIAN_POINT('Ctrl Pts',(3.41878447232058,2.37589363434567,5.2));
#20272=CARTESIAN_POINT('Ctrl Pts',(3.41878798568376,2.3791143017356,5.2));
#20273=CARTESIAN_POINT('Ctrl Pts',(3.41880075844281,2.39082297128446,5.2));
#20274=CARTESIAN_POINT('Ctrl Pts',(3.41994282155898,2.40251786108517,5.2));
#20275=CARTESIAN_POINT('Ctrl Pts',(3.42216878897262,2.41402665747967,5.2));
#20276=CARTESIAN_POINT('Ctrl Pts',(3.42331180168116,2.41993631296624,5.2));
#20277=CARTESIAN_POINT('Ctrl Pts',(3.42474130312271,2.42579671745434,5.2));
#20278=CARTESIAN_POINT('Ctrl Pts',(3.4264550762976,2.43158227576526,5.2));
#20279=CARTESIAN_POINT('Ctrl Pts',(3.42814231216907,2.43727824630656,5.2));
#20280=CARTESIAN_POINT('Ctrl Pts',(3.43010783958643,2.44290710782216,5.2));
#20281=CARTESIAN_POINT('Ctrl Pts',(3.43233768577066,2.4484115412056,5.2));
#20282=CARTESIAN_POINT('Ctrl Pts',(3.43579440729991,2.4569445483329,5.2));
#20283=CARTESIAN_POINT('Ctrl Pts',(3.43988798414899,2.46519216359733,5.2));
#20284=CARTESIAN_POINT('Ctrl Pts',(3.44460907372922,2.4730585225122,5.2));
#20285=CARTESIAN_POINT('Ctrl Pts',(3.44702309019998,2.47708079738387,5.2));
#20286=CARTESIAN_POINT('Ctrl Pts',(3.44960209705083,2.48100348334585,5.2));
#20287=CARTESIAN_POINT('Ctrl Pts',(3.45233605468006,2.48480007154667,5.2));
#20288=CARTESIAN_POINT('Ctrl Pts',(3.45777065901345,2.49234698978257,5.2));
#20289=CARTESIAN_POINT('Ctrl Pts',(3.46382415870923,2.499410402925,5.2));
#20290=CARTESIAN_POINT('Ctrl Pts',(3.47049190322584,2.5058791831385,5.2));
#20291=CARTESIAN_POINT('Ctrl Pts',(3.47127037259775,2.50663442312367,5.2));
#20292=CARTESIAN_POINT('Ctrl Pts',(3.47205722899383,2.5073815321984,5.2));
#20293=CARTESIAN_POINT('Ctrl Pts',(3.47285231527688,2.50812044463164,5.2));
#20294=CARTESIAN_POINT('Origin',(3.6,2.4,4.7));
#20295=CARTESIAN_POINT('Origin',(3.6,-2.4,4.2));
#20296=CARTESIAN_POINT('Origin',(-3.6,-2.4,4.2));
#20297=CARTESIAN_POINT('Origin',(-3.6,2.4,4.2));
#20298=CARTESIAN_POINT('Origin',(3.6,2.4,4.2));
#20299=CARTESIAN_POINT('Origin',(-4.6,0.,0.3));
#20300=CARTESIAN_POINT('',(-4.9,3.67394039744206E-17,0.6));
#20301=CARTESIAN_POINT('Origin',(-4.6,0.,0.6));
#20302=CARTESIAN_POINT('',(-4.9,3.67394039744206E-17,0.));
#20303=CARTESIAN_POINT('',(-4.9,3.67394039744206E-17,0.3));
#20304=CARTESIAN_POINT('Origin',(-4.6,0.,0.));
#20305=CARTESIAN_POINT('Origin',(4.6,0.,0.3));
#20306=CARTESIAN_POINT('',(4.3,3.67394039744206E-17,0.6));
#20307=CARTESIAN_POINT('Origin',(4.6,0.,0.6));
#20308=CARTESIAN_POINT('',(4.3,3.67394039744206E-17,0.));
#20309=CARTESIAN_POINT('',(4.3,3.67394039744206E-17,0.3));
#20310=CARTESIAN_POINT('Origin',(4.6,0.,0.));
#20311=CARTESIAN_POINT('Origin',(5.2,1.,0.));
#20312=CARTESIAN_POINT('',(5.2,1.,0.));
#20313=CARTESIAN_POINT('',(4.,1.,0.));
#20314=CARTESIAN_POINT('',(5.2,1.,0.));
#20315=CARTESIAN_POINT('',(4.,1.,0.6));
#20316=CARTESIAN_POINT('',(4.,1.,0.));
#20317=CARTESIAN_POINT('',(5.2,1.,0.6));
#20318=CARTESIAN_POINT('',(5.2,1.,0.6));
#20319=CARTESIAN_POINT('',(5.2,1.,0.));
#20320=CARTESIAN_POINT('Origin',(5.2,-1.,0.));
#20321=CARTESIAN_POINT('',(5.2,-1.,0.));
#20322=CARTESIAN_POINT('',(5.2,-1.,0.));
#20323=CARTESIAN_POINT('',(5.2,-1.,0.6));
#20324=CARTESIAN_POINT('',(5.2,-1.,0.6));
#20325=CARTESIAN_POINT('',(5.2,-1.,0.));
#20326=CARTESIAN_POINT('Origin',(4.,-1.,0.));
#20327=CARTESIAN_POINT('',(4.,-1.,0.));
#20328=CARTESIAN_POINT('',(4.,-1.,0.));
#20329=CARTESIAN_POINT('',(4.,-1.,0.6));
#20330=CARTESIAN_POINT('',(4.,-1.,0.6));
#20331=CARTESIAN_POINT('',(4.,-1.,0.));
#20332=CARTESIAN_POINT('Origin',(4.6,0.,0.6));
#20333=CARTESIAN_POINT('',(4.,-1.4,0.6));
#20334=CARTESIAN_POINT('Origin',(-4.,1.,0.));
#20335=CARTESIAN_POINT('',(-4.,1.,0.));
#20336=CARTESIAN_POINT('',(-5.2,1.,0.));
#20337=CARTESIAN_POINT('',(-4.,1.,0.));
#20338=CARTESIAN_POINT('',(-5.2,1.,0.6));
#20339=CARTESIAN_POINT('',(-5.2,1.,0.));
#20340=CARTESIAN_POINT('',(-4.,1.,0.6));
#20341=CARTESIAN_POINT('',(-4.,1.,0.6));
#20342=CARTESIAN_POINT('',(-4.,1.,0.));
#20343=CARTESIAN_POINT('Origin',(-5.2,-1.,0.));
#20344=CARTESIAN_POINT('',(-5.2,-1.,0.));
#20345=CARTESIAN_POINT('',(-4.,-1.,0.));
#20346=CARTESIAN_POINT('',(-5.2,-1.,0.));
#20347=CARTESIAN_POINT('',(-4.,-1.,0.6));
#20348=CARTESIAN_POINT('',(-4.,-1.,0.));
#20349=CARTESIAN_POINT('',(-5.2,-1.,0.6));
#20350=CARTESIAN_POINT('',(-5.2,-1.,0.6));
#20351=CARTESIAN_POINT('',(-5.2,-1.,0.));
#20352=CARTESIAN_POINT('Origin',(-5.2,1.,0.));
#20353=CARTESIAN_POINT('',(-5.2,1.,0.));
#20354=CARTESIAN_POINT('',(-5.2,1.,0.6));
#20355=CARTESIAN_POINT('Origin',(-4.6,0.,0.6));
#20356=CARTESIAN_POINT('',(-4.,1.4,0.6));
#20357=CARTESIAN_POINT('Origin',(0.,0.,0.8));
#20358=CARTESIAN_POINT('',(-0.65,-7.9602041944578E-17,1.6));
#20359=CARTESIAN_POINT('Origin',(0.,0.,1.6));
#20360=CARTESIAN_POINT('',(-0.65,-7.9602041944578E-17,0.8));
#20361=CARTESIAN_POINT('',(-0.65,-7.9602041944578E-17,0.8));
#20362=CARTESIAN_POINT('Origin',(0.,0.,0.8));
#20363=CARTESIAN_POINT('Origin',(0.,0.,0.8));
#20364=CARTESIAN_POINT('',(-0.8,-9.79717439317883E-17,1.6));
#20365=CARTESIAN_POINT('Origin',(0.,0.,1.6));
#20366=CARTESIAN_POINT('',(-0.8,-9.79717439317883E-17,0.8));
#20367=CARTESIAN_POINT('Origin',(0.,0.,1.6));
#20368=CARTESIAN_POINT('Origin',(-3.2,-2.,5.2));
#20369=CARTESIAN_POINT('',(-3.2,-1.,5.2));
#20370=CARTESIAN_POINT('Origin',(0.,0.,0.8));
#20371=CARTESIAN_POINT('Origin',(4.,2.8,0.));
#20372=CARTESIAN_POINT('',(4.,2.8,0.));
#20373=CARTESIAN_POINT('',(-4.,2.8,0.));
#20374=CARTESIAN_POINT('',(4.,2.8,0.));
#20375=CARTESIAN_POINT('',(-4.,2.8,5.2));
#20376=CARTESIAN_POINT('',(-4.,2.8,0.));
#20377=CARTESIAN_POINT('',(4.,2.8,5.2));
#20378=CARTESIAN_POINT('',(4.,2.8,5.2));
#20379=CARTESIAN_POINT('',(4.,2.8,0.));
#20380=CARTESIAN_POINT('Origin',(4.,-2.8,0.));
#20381=CARTESIAN_POINT('',(4.,-2.8,0.));
#20382=CARTESIAN_POINT('',(4.,-2.8,5.2));
#20383=CARTESIAN_POINT('',(4.,-2.8,5.2));
#20384=CARTESIAN_POINT('',(4.,-2.8,0.));
#20385=CARTESIAN_POINT('',(4.,-2.8,0.));
#20386=CARTESIAN_POINT('',(4.,-2.8,0.));
#20387=CARTESIAN_POINT('Origin',(-4.,-2.8,0.));
#20388=CARTESIAN_POINT('',(-4.,-2.8,0.));
#20389=CARTESIAN_POINT('',(-4.,-2.8,0.));
#20390=CARTESIAN_POINT('',(-4.,-2.8,5.2));
#20391=CARTESIAN_POINT('',(-4.,-2.8,5.2));
#20392=CARTESIAN_POINT('',(-4.,-2.8,0.));
#20393=CARTESIAN_POINT('Origin',(-4.,2.8,0.));
#20394=CARTESIAN_POINT('',(-4.,2.8,0.));
#20395=CARTESIAN_POINT('',(-4.,2.8,5.2));
#20396=CARTESIAN_POINT('',(-4.,2.8,0.));
#20397=CARTESIAN_POINT('Origin',(0.,0.,5.2));
#20398=CARTESIAN_POINT('Origin',(0.,0.,0.));
#36446=UNCERTAINTY_MEASURE_WITH_UNIT(LENGTH_MEASURE(0.001),#36483,
'DISTANCE_ACCURACY_VALUE',
'Maximum model space distance between geometric entities at asserted c
onnectivities');
#36463=UNCERTAINTY_MEASURE_WITH_UNIT(LENGTH_MEASURE(0.001),#36483,
'DISTANCE_ACCURACY_VALUE',
'Maximum model space distance between geometric entities at asserted c
onnectivities');
#36465=(
GEOMETRIC_REPRESENTATION_CONTEXT(3)
GLOBAL_UNCERTAINTY_ASSIGNED_CONTEXT((#36446))
GLOBAL_UNIT_ASSIGNED_CONTEXT((#36483,#36485,#36486))
REPRESENTATION_CONTEXT('','3D')
);
#36482=(
GEOMETRIC_REPRESENTATION_CONTEXT(3)
GLOBAL_UNCERTAINTY_ASSIGNED_CONTEXT((#36463))
GLOBAL_UNIT_ASSIGNED_CONTEXT((#36483,#36485,#36486))
REPRESENTATION_CONTEXT('','3D')
);
#36483=(
LENGTH_UNIT()
NAMED_UNIT(*)
SI_UNIT(.CENTI.,.METRE.)
);
#36485=(
NAMED_UNIT(*)
PLANE_ANGLE_UNIT()
SI_UNIT($,.RADIAN.)
);
#36486=(
NAMED_UNIT(*)
SI_UNIT($,.STERADIAN.)
SOLID_ANGLE_UNIT()
);
#36488=SHAPE_DEFINITION_REPRESENTATION(#36506,#36555);
#36506=PRODUCT_DEFINITION_SHAPE('',$,#36574);
#36555=SHAPE_REPRESENTATION('',(#9973),#36465);
#36572=PRODUCT_DEFINITION_CONTEXT('part definition',#36628,'design');
#36574=PRODUCT_DEFINITION('Switch housing','Switch housing',#36592,#36572);
#36592=PRODUCT_DEFINITION_FORMATION('',$,#36631);
#36628=APPLICATION_CONTEXT(
'Core Data for Automotive Mechanical Design Process');
#36629=PRODUCT_CONTEXT('part definition',#36628,'mechanical');
#36631=PRODUCT('Switch housing','Switch housing',$,(#36629));
#36649=PRESENTATION_STYLE_ASSIGNMENT((#36663));
#36663=SURFACE_STYLE_USAGE(.BOTH.,#36677);
#36677=SURFACE_SIDE_STYLE('',(#36691));
#36691=SURFACE_STYLE_FILL_AREA(#36705);
#36705=FILL_AREA_STYLE('Dark blue',(#36719));
#36719=FILL_AREA_STYLE_COLOUR('Dark blue',#36733);
#36733=COLOUR_RGB('Dark blue',0.0901960784313725,0.270588235294118,0.513725490196078);
ENDSEC;
END-ISO-10303-21;
